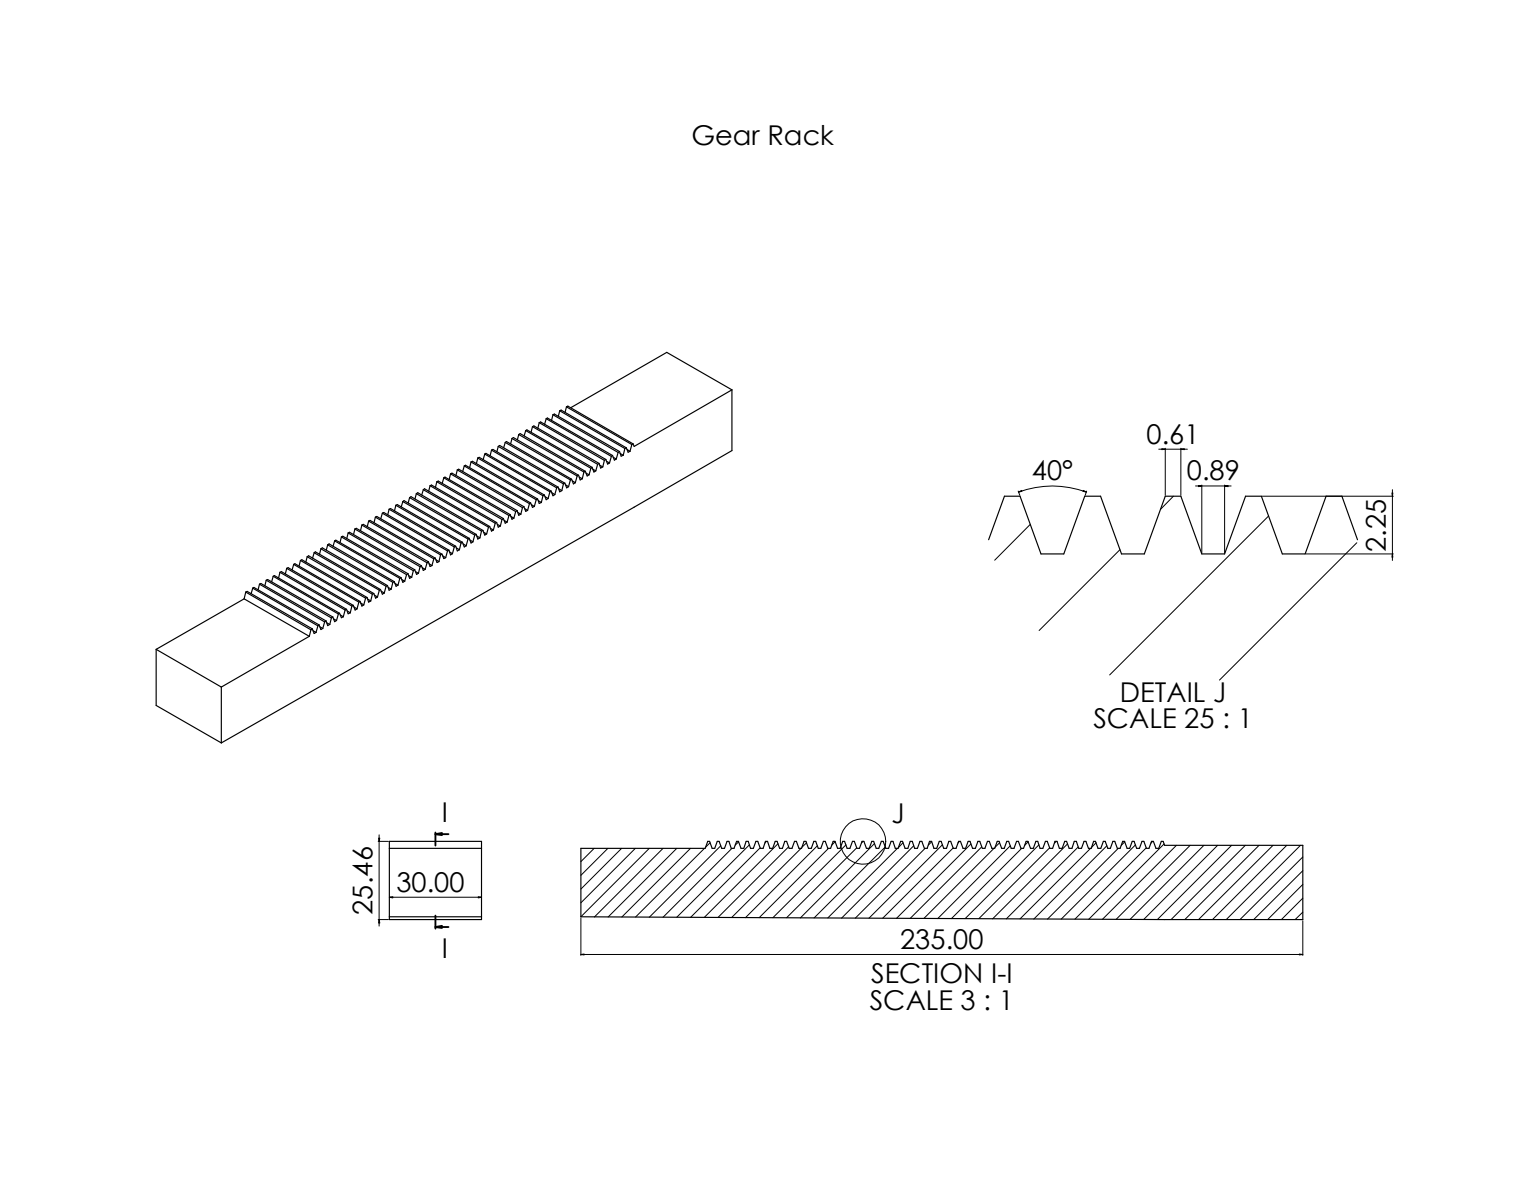
ISO-10303-21;
HEADER;
FILE_DESCRIPTION (('STEP AP214'),
    '1' );
FILE_NAME ('Gear Rack.step',
    '2026-10-21T18:33:49',
    ( '' ),
    ( '' ),
    'SwSTEP 2.0',
    'SolidWorks 2025',
    '' );
FILE_SCHEMA (( 'AUTOMOTIVE_DESIGN' ));
ENDSEC;

DATA;
#3=EDGE_CURVE ( 'NONE', #15101, #1867, #14100, .T. ) ;
#5=DIRECTION ( 'NONE',  ( 0.000000000000000000, 1.000000000000000000, 0.000000000000000000 ) ) ;
#8=FACE_OUTER_BOUND ( 'NONE', #9764, .T. ) ;
#9=EDGE_CURVE ( 'NONE', #4281, #6184, #12794, .T. ) ;
#10=CARTESIAN_POINT ( 'NONE',  ( -68.99615306438082030, 67.98345733813023628, 15.00000000000006928 ) ) ;
#22=ORIENTED_EDGE ( 'NONE', *, *, #922, .F. ) ;
#25=ORIENTED_EDGE ( 'NONE', *, *, #4430, .T. ) ;
#29=VECTOR ( 'NONE', #2801, 1000.000000000000000 ) ;
#33=CARTESIAN_POINT ( 'NONE',  ( -68.99615306438083451, 95.64293533166268446, -15.00000000000001421 ) ) ;
#34=ORIENTED_EDGE ( 'NONE', *, *, #18366, .F. ) ;
#43=CARTESIAN_POINT ( 'NONE',  ( -71.24615306438076345, 119.9567435045637609, 15.00000000000006928 ) ) ;
#54=ORIENTED_EDGE ( 'NONE', *, *, #5988, .F. ) ;
#57=DIRECTION ( 'NONE',  ( 0.000000000000000000, 0.000000000000000000, 1.000000000000000000 ) ) ;
#59=CARTESIAN_POINT ( 'NONE',  ( -71.24615306438080609, 110.5319655545637403, -15.00000000000001421 ) ) ;
#67=DIRECTION ( 'NONE',  ( 1.000000000000000000, 0.000000000000000000, 0.000000000000000000 ) ) ;
#68=DIRECTION ( 'NONE',  ( 0.000000000000000000, 0.000000000000000000, -1.000000000000000000 ) ) ;
#69=LINE ( 'NONE', #1924, #3643 ) ;
#73=LINE ( 'NONE', #1738, #2546 ) ;
#74=CARTESIAN_POINT ( 'NONE',  ( -71.24615306438114715, 12.25372266522925457, -15.00000000000001421 ) ) ;
#76=CARTESIAN_POINT ( 'NONE',  ( -68.99615306438099083, 39.70912348813027393, -15.00000000000001421 ) ) ;
#77=ORIENTED_EDGE ( 'NONE', *, *, #12373, .F. ) ;
#78=ORIENTED_EDGE ( 'NONE', *, *, #14054, .T. ) ;
#79=VECTOR ( 'NONE', #3026, 1000.000000000000000 ) ;
#80=FACE_OUTER_BOUND ( 'NONE', #8908, .T. ) ;
#82=VECTOR ( 'NONE', #10770, 1000.000000000000000 ) ;
#87=CARTESIAN_POINT ( 'NONE',  ( -71.24615306438086293, 87.65194626522927024, 15.00000000000006928 ) ) ;
#88=CARTESIAN_POINT ( 'NONE',  ( -71.24615306438103346, 41.41692725456378099, 15.00000000000006928 ) ) ;
#93=ORIENTED_EDGE ( 'NONE', *, *, #600, .F. ) ;
#95=AXIS2_PLACEMENT_3D ( 'NONE', #13870, #16563, #957 ) ;
#100=VECTOR ( 'NONE', #7999, 1000.000000000000000 ) ;
#101=CARTESIAN_POINT ( 'NONE',  ( -71.24615306438103346, 46.81124181522922356, -167.1454815528550739 ) ) ;
#102=ORIENTED_EDGE ( 'NONE', *, *, #5033, .T. ) ;
#103=VERTEX_POINT ( 'NONE', #8932 ) ;
#105=EDGE_CURVE ( 'NONE', #6184, #7713, #7257, .T. ) ;
#106=DIRECTION ( 'NONE',  ( 0.000000000000000000, 0.000000000000000000, 1.000000000000000000 ) ) ;
#107=CARTESIAN_POINT ( 'NONE',  ( -68.99615306438077766, 111.3508985816626335, 15.00000000000006928 ) ) ;
#108=DIRECTION ( 'NONE',  ( 0.9396926207859110924, 0.3420201433256612189, 4.890320548438462711E-16 ) ) ;
#109=CARTESIAN_POINT ( 'NONE',  ( -68.99615306438083451, 96.25779118813026969, 15.00000000000006928 ) ) ;
#112=CARTESIAN_POINT ( 'NONE',  ( -68.99615306438094819, 64.84186468813030046, -167.1454815528550739 ) ) ;
#115=VERTEX_POINT ( 'NONE', #11567 ) ;
#120=ADVANCED_FACE ( 'NONE', ( #317 ), #17523, .T. ) ;
#123=EDGE_CURVE ( 'NONE', #14184, #1161, #17431, .T. ) ;
#127=ORIENTED_EDGE ( 'NONE', *, *, #11107, .F. ) ;
#131=DIRECTION ( 'NONE',  ( 0.000000000000000000, 1.000000000000000000, 0.000000000000000000 ) ) ;
#132=CLOSED_SHELL ( 'NONE', ( #16819, #11674, #2033, #11644, #4371, #4122, #1296, #5932, #17847, #120, #2885, #7783, #14078, #8551, #16458, #7777, #18333, #11455, #10717, #14761, #5893, #8655, #18440, #16557, #12743, #9060, #2113, #2878, #10557, #2402, #8018, #1483, #10883, #4144, #6355, #12130, #16320, #4815, #13864, #11004, #16568, #13389, #1952, #7426, #15874, #4708, #2702, #9166, #6647, #9938, #17322, #16215, #6855, #13752, #18352, #9497, #4258, #1742, #6653, #8457, #4789, #9269, #18511, #11812, #1620, #13520, #17365, #6946, #1859, #1613, #14320, #1393, #8249, #8120, #5145, #15892, #8683, #10886, #4488, #15641, #15634, #1683, #17355, #13695, #2863, #11359, #9380, #16584, #2602, #1587, #18091, #10091, #697, #5265, #11665, #1664, #1494, #15112, #7329, #13942, #12957, #5269, #13366, #4588, #17837, #11471, #8147, #8734, #4244, #11669, #7993, #15996, #11378, #16587, #15586, #9173, #1719, #9985, #9137, #3228, #3620, #3217, #7092, #3899, #10422, #4564, #11884, #18090, #10942, #9980, #5134, #5026, #2281, #4013, #13406, #12017, #13887, #8689, #14413, #199, #11412, #7110, #12033, #2993, #2286, #360, #17572, #10733, #12952, #12754, #9744, #1961, #13863, #8387, #17357, #7212, #8267, #16341, #10832, #3777, #7577, #14524, #13388, #3293, #4798, #16330, #4522, #14219, #18302, #4015, #3342, #248, #17345, #4135, #15214, #12844, #9850, #14995, #14426, #12814, #8137, #5256, #5374, #4240, #691, #4541, #672, #7328, #12390, #3982, #7563, #1284, #2154, #15527, #5570, #7390, #1348, #13976, #16311 ) ) ;
#133=ORIENTED_EDGE ( 'NONE', *, *, #16066, .F. ) ;
#135=ORIENTED_EDGE ( 'NONE', *, *, #18293, .T. ) ;
#136=VECTOR ( 'NONE', #9589, 1000.000000000000000 ) ;
#137=EDGE_CURVE ( 'NONE', #18033, #6955, #3220, .T. ) ;
#140=EDGE_CURVE ( 'NONE', #5342, #10434, #506, .T. ) ;
#141=AXIS2_PLACEMENT_3D ( 'NONE', #1798, #14535, #303 ) ;
#142=CARTESIAN_POINT ( 'NONE',  ( -71.24615306438106188, 35.13374195456378146, 15.00000000000006928 ) ) ;
#146=VECTOR ( 'NONE', #7240, 1000.000000000000114 ) ;
#158=DIRECTION ( 'NONE',  ( 0.000000000000000000, 0.000000000000000000, -1.000000000000000000 ) ) ;
#160=CARTESIAN_POINT ( 'NONE',  ( -68.99615306438087714, 64.84186468813027204, 15.00000000000006928 ) ) ;
#161=LINE ( 'NONE', #5851, #4306 ) ;
#163=CARTESIAN_POINT ( 'NONE',  ( -71.24615306438072082, 129.3815214545637104, -15.00000000000001421 ) ) ;
#165=DIRECTION ( 'NONE',  ( 0.000000000000000000, 1.000000000000000000, 0.000000000000000000 ) ) ;
#167=ORIENTED_EDGE ( 'NONE', *, *, #3319, .T. ) ;
#168=DIRECTION ( 'NONE',  ( 0.000000000000000000, -1.000000000000000000, 0.000000000000000000 ) ) ;
#172=VECTOR ( 'NONE', #13804, 1000.000000000000000 ) ;
#174=VECTOR ( 'NONE', #6629, 999.9999999999998863 ) ;
#178=EDGE_LOOP ( 'NONE', ( #16402, #10742, #3348, #2661 ) ) ;
#182=VECTOR ( 'NONE', #7830, 1000.000000000000000 ) ;
#185=ORIENTED_EDGE ( 'NONE', *, *, #7525, .T. ) ;
#189=DIRECTION ( 'NONE',  ( -0.9396926207859084279, 0.3420201433256686574, -4.890320548438448905E-16 ) ) ;
#196=CARTESIAN_POINT ( 'NONE',  ( -93.73308511844572877, 147.7866419848965052, 15.00000000000006928 ) ) ;
#198=ORIENTED_EDGE ( 'NONE', *, *, #17480, .F. ) ;
#199=ADVANCED_FACE ( 'NONE', ( #6677 ), #6475, .T. ) ;
#202=LINE ( 'NONE', #14676, #5765 ) ;
#207=CARTESIAN_POINT ( 'NONE',  ( -68.99615306438072082, 139.6252324316626812, -15.00000000000001421 ) ) ;
#211=CARTESIAN_POINT ( 'NONE',  ( -71.24615306438094819, 65.66079771522920794, 15.00000000000006928 ) ) ;
#213=ORIENTED_EDGE ( 'NONE', *, *, #3679, .F. ) ;
#218=DIRECTION ( 'NONE',  ( 0.000000000000000000, 0.000000000000000000, 1.000000000000000000 ) ) ;
#222=FACE_OUTER_BOUND ( 'NONE', #11208, .T. ) ;
#224=CARTESIAN_POINT ( 'NONE',  ( -68.99615306438066398, 143.3816809381303585, -15.00000000000001421 ) ) ;
#226=EDGE_CURVE ( 'NONE', #10713, #3636, #7893, .T. ) ;
#228=ORIENTED_EDGE ( 'NONE', *, *, #586, .F. ) ;
#230=EDGE_LOOP ( 'NONE', ( #6684, #5867, #2533, #3953 ) ) ;
#232=EDGE_CURVE ( 'NONE', #7225, #15152, #10982, .T. ) ;
#235=CARTESIAN_POINT ( 'NONE',  ( -68.99615306438097662, 57.94382353166266597, 15.00000000000006928 ) ) ;
#238=CARTESIAN_POINT ( 'NONE',  ( -68.99615306438094819, 52.27549408813023746, -15.00000000000001421 ) ) ;
#239=CARTESIAN_POINT ( 'NONE',  ( -68.99615306438091977, 76.79337943166271430, 15.00000000000006928 ) ) ;
#242=EDGE_CURVE ( 'NONE', #13281, #15993, #13414, .T. ) ;
#243=CARTESIAN_POINT ( 'NONE',  ( 0.000000000000000000, -47.21335801510345220, 0.000000000000000000 ) ) ;
#245=DIRECTION ( 'NONE',  ( 0.000000000000000000, 1.000000000000000000, 0.000000000000000000 ) ) ;
#246=CARTESIAN_POINT ( 'NONE',  ( -68.99615306438089135, 67.36860148166267948, -15.00000000000001421 ) ) ;
#248=ADVANCED_FACE ( 'NONE', ( #16665 ), #17710, .T. ) ;
#250=EDGE_CURVE ( 'NONE', #2407, #15787, #4070, .T. ) ;
#252=DIRECTION ( 'NONE',  ( 0.000000000000000000, 0.000000000000000000, 1.000000000000000000 ) ) ;
#254=EDGE_LOOP ( 'NONE', ( #4957, #10703, #17741, #2803 ) ) ;
#260=DIRECTION ( 'NONE',  ( 1.000000000000000000, 0.000000000000000000, 0.000000000000000000 ) ) ;
#261=VECTOR ( 'NONE', #17294, 1000.000000000000000 ) ;
#276=LINE ( 'NONE', #12841, #12086 ) ;
#277=CARTESIAN_POINT ( 'NONE',  ( -71.24615306438070661, 137.9174286652292096, -15.00000000000001421 ) ) ;
#278=CARTESIAN_POINT ( 'NONE',  ( -68.99615306438091977, 76.79337943166271430, 15.00000000000006928 ) ) ;
#279=DIRECTION ( 'NONE',  ( -0.9396926207859097602, 0.3420201433256649937, 1.086737899652991371E-16 ) ) ;
#280=CARTESIAN_POINT ( 'NONE',  ( -93.73308511844572877, 147.7866419848965052, -167.1454815528550739 ) ) ;
#281=CARTESIAN_POINT ( 'NONE',  ( -71.24615306438117557, 2.828944715229236628, -15.00000000000001421 ) ) ;
#282=ORIENTED_EDGE ( 'NONE', *, *, #10987, .T. ) ;
#287=CARTESIAN_POINT ( 'NONE',  ( -71.24615306438091977, 78.22716831522920700, -167.1454815528550739 ) ) ;
#288=VERTEX_POINT ( 'NONE', #1257 ) ;
#289=LINE ( 'NONE', #11809, #4058 ) ;
#291=ORIENTED_EDGE ( 'NONE', *, *, #13628, .T. ) ;
#292=VECTOR ( 'NONE', #17881, 1000.000000000000000 ) ;
#294=AXIS2_PLACEMENT_3D ( 'NONE', #10449, #2985, #15881 ) ;
#296=LINE ( 'NONE', #5733, #146 ) ;
#298=LINE ( 'NONE', #4419, #17998 ) ;
#300=ORIENTED_EDGE ( 'NONE', *, *, #349, .T. ) ;
#303=DIRECTION ( 'NONE',  ( -0.9396926207859083169, 0.3420201433256687129, 0.000000000000000000 ) ) ;
#308=PLANE ( 'NONE',  #11935 ) ;
#312=AXIS2_PLACEMENT_3D ( 'NONE', #18500, #6897, #18319 ) ;
#316=VECTOR ( 'NONE', #2722, 1000.000000000000000 ) ;
#317=FACE_OUTER_BOUND ( 'NONE', #5144, .T. ) ;
#320=LINE ( 'NONE', #12982, #15345 ) ;
#324=FACE_OUTER_BOUND ( 'NONE', #5532, .T. ) ;
#327=CARTESIAN_POINT ( 'NONE',  ( -71.24615306438086293, 101.1071876045637055, 15.00000000000006928 ) ) ;
#333=EDGE_CURVE ( 'NONE', #677, #12056, #6961, .T. ) ;
#338=ORIENTED_EDGE ( 'NONE', *, *, #1743, .T. ) ;
#339=ORIENTED_EDGE ( 'NONE', *, *, #18046, .F. ) ;
#341=EDGE_LOOP ( 'NONE', ( #13382, #1827, #3873, #1999 ) ) ;
#342=EDGE_CURVE ( 'NONE', #6852, #6867, #8831, .T. ) ;
#344=EDGE_CURVE ( 'NONE', #16643, #10257, #17318, .T. ) ;
#346=LINE ( 'NONE', #14229, #2566 ) ;
#349=EDGE_CURVE ( 'NONE', #6911, #16349, #396, .T. ) ;
#354=AXIS2_PLACEMENT_3D ( 'NONE', #17589, #6266, #16189 ) ;
#360=ADVANCED_FACE ( 'NONE', ( #11718 ), #4683, .T. ) ;
#364=EDGE_LOOP ( 'NONE', ( #17923, #6580, #8232, #7279 ) ) ;
#366=EDGE_CURVE ( 'NONE', #16976, #11956, #1702, .T. ) ;
#368=( LENGTH_UNIT ( ) NAMED_UNIT ( * ) SI_UNIT ( .MILLI., .METRE. ) );
#371=AXIS2_PLACEMENT_3D ( 'NONE', #10964, #16647, #17683 ) ;
#372=EDGE_LOOP ( 'NONE', ( #7742, #5661, #16335, #12943 ) ) ;
#376=EDGE_CURVE ( 'NONE', #3236, #18474, #3199, .T. ) ;
#379=AXIS2_PLACEMENT_3D ( 'NONE', #9478, #9862, #8069 ) ;
#381=DIRECTION ( 'NONE',  ( 0.9396926207859097602, 0.3420201433256649937, -1.086737899652991371E-16 ) ) ;
#382=ORIENTED_EDGE ( 'NONE', *, *, #14734, .F. ) ;
#383=DIRECTION ( 'NONE',  ( 0.000000000000000000, 1.000000000000000000, 0.000000000000000000 ) ) ;
#385=VECTOR ( 'NONE', #2920, 999.9999999999998863 ) ;
#387=DIRECTION ( 'NONE',  ( 0.000000000000000000, 1.000000000000000000, 0.000000000000000000 ) ) ;
#393=AXIS2_PLACEMENT_3D ( 'NONE', #6338, #7848, #6238 ) ;
#396=LINE ( 'NONE', #4417, #4324 ) ;
#403=DIRECTION ( 'NONE',  ( -0.9396926207859103153, 0.3420201433256634949, -4.890320548438458766E-16 ) ) ;
#405=DIRECTION ( 'NONE',  ( 1.000000000000000000, 0.000000000000000000, 0.000000000000000000 ) ) ;
#406=DIRECTION ( 'NONE',  ( 0.000000000000000000, 0.000000000000000000, 1.000000000000000000 ) ) ;
#407=ORIENTED_EDGE ( 'NONE', *, *, #6384, .T. ) ;
#409=VERTEX_POINT ( 'NONE', #8909 ) ;
#410=VECTOR ( 'NONE', #11298, 1000.000000000000000 ) ;
#411=FACE_OUTER_BOUND ( 'NONE', #8890, .T. ) ;
#413=ORIENTED_EDGE ( 'NONE', *, *, #7885, .T. ) ;
#418=CARTESIAN_POINT ( 'NONE',  ( -71.24615306438117557, 6.859408104563785358, -15.00000000000001421 ) ) ;
#419=ORIENTED_EDGE ( 'NONE', *, *, #16175, .T. ) ;
#422=VECTOR ( 'NONE', #7146, 1000.000000000000000 ) ;
#423=PLANE ( 'NONE',  #11407 ) ;
#425=VERTEX_POINT ( 'NONE', #6170 ) ;
#427=CARTESIAN_POINT ( 'NONE',  ( -68.99615306438070661, 136.4836397816626743, -167.1454815528550739 ) ) ;
#438=ORIENTED_EDGE ( 'NONE', *, *, #10980, .F. ) ;
#442=LINE ( 'NONE', #4723, #8228 ) ;
#444=PLANE ( 'NONE',  #8468 ) ;
#446=ORIENTED_EDGE ( 'NONE', *, *, #6478, .T. ) ;
#448=CARTESIAN_POINT ( 'NONE',  ( -71.24615306438118978, 0.5762228045637974860, -15.00000000000001421 ) ) ;
#450=FACE_OUTER_BOUND ( 'NONE', #16283, .T. ) ;
#455=VERTEX_POINT ( 'NONE', #1621 ) ;
#459=EDGE_CURVE ( 'NONE', #18478, #6989, #7332, .T. ) ;
#462=ORIENTED_EDGE ( 'NONE', *, *, #9043, .F. ) ;
#463=ORIENTED_EDGE ( 'NONE', *, *, #6166, .F. ) ;
#464=VECTOR ( 'NONE', #12334, 1000.000000000000000 ) ;
#471=CARTESIAN_POINT ( 'NONE',  ( -71.24615306438091977, 72.83285375456371469, 15.00000000000006928 ) ) ;
#473=DIRECTION ( 'NONE',  ( 0.3420201433256686574, -0.9396926207859084279, 0.000000000000000000 ) ) ;
#474=PLANE ( 'NONE',  #12259 ) ;
#478=EDGE_CURVE ( 'NONE', #12432, #2231, #13393, .T. ) ;
#483=DIRECTION ( 'NONE',  ( -1.000000000000000000, 0.000000000000000000, -5.022391976381918634E-16 ) ) ;
#490=CARTESIAN_POINT ( 'NONE',  ( -68.99615306438077766, 111.3508985816626335, -167.1454815528550739 ) ) ;
#494=LINE ( 'NONE', #576, #5416 ) ;
#495=ORIENTED_EDGE ( 'NONE', *, *, #6626, .T. ) ;
#499=CARTESIAN_POINT ( 'NONE',  ( -71.24615306438114715, 10.00100075456375492, -167.1454815528550739 ) ) ;
#500=ORIENTED_EDGE ( 'NONE', *, *, #3536, .F. ) ;
#501=ORIENTED_EDGE ( 'NONE', *, *, #3133, .T. ) ;
#506=LINE ( 'NONE', #10147, #14475 ) ;
#508=ORIENTED_EDGE ( 'NONE', *, *, #8600, .F. ) ;
#509=LINE ( 'NONE', #239, #10786 ) ;
#515=DIRECTION ( 'NONE',  ( -0.9396926207859008784, 0.3420201433256891965, 0.000000000000000000 ) ) ;
#520=ORIENTED_EDGE ( 'NONE', *, *, #4378, .T. ) ;
#521=ORIENTED_EDGE ( 'NONE', *, *, #1743, .F. ) ;
#527=CARTESIAN_POINT ( 'NONE',  ( -68.99615306438094819, 54.80223088166269463, 15.00000000000006928 ) ) ;
#529=CARTESIAN_POINT ( 'NONE',  ( -68.99615306438074924, 121.3905323881302962, -167.1454815528550739 ) ) ;
#531=CARTESIAN_POINT ( 'NONE',  ( -71.24615306438101925, 31.99214930456378880, 15.00000000000006928 ) ) ;
#533=VECTOR ( 'NONE', #2270, 1000.000000000000000 ) ;
#536=LINE ( 'NONE', #14927, #15963 ) ;
#547=CARTESIAN_POINT ( 'NONE',  ( -71.24615306438089135, 81.36876096522922808, 15.00000000000006928 ) ) ;
#555=LINE ( 'NONE', #16078, #14389 ) ;
#557=DIRECTION ( 'NONE',  ( -0.9396926207859093161, 0.3420201433256661594, 0.000000000000000000 ) ) ;
#558=VECTOR ( 'NONE', #1688, 1000.000000000000000 ) ;
#560=EDGE_CURVE ( 'NONE', #11029, #18478, #7961, .T. ) ;
#562=DIRECTION ( 'NONE',  ( 0.000000000000000000, 0.000000000000000000, 1.000000000000000000 ) ) ;
#564=ORIENTED_EDGE ( 'NONE', *, *, #8838, .T. ) ;
#568=DIRECTION ( 'NONE',  ( 0.3420201433256649937, -0.9396926207859097602, 0.000000000000000000 ) ) ;
#574=CARTESIAN_POINT ( 'NONE',  ( -71.24615306438076345, 132.5231141045637457, -15.00000000000001421 ) ) ;
#576=CARTESIAN_POINT ( 'NONE',  ( -71.24615306438084872, 72.83285375456374311, 15.00000000000006928 ) ) ;
#581=DIRECTION ( 'NONE',  ( -0.9396926207859084279, 0.3420201433256686574, 1.086737899652989892E-16 ) ) ;
#584=CARTESIAN_POINT ( 'NONE',  ( -71.24615306438091977, 71.94398301522919326, 15.00000000000006928 ) ) ;
#585=ORIENTED_EDGE ( 'NONE', *, *, #478, .F. ) ;
#586=EDGE_CURVE ( 'NONE', #15423, #5470, #3374, .T. ) ;
#587=EDGE_CURVE ( 'NONE', #1317, #10161, #1984, .T. ) ;
#589=ORIENTED_EDGE ( 'NONE', *, *, #5376, .F. ) ;
#590=VECTOR ( 'NONE', #9664, 1000.000000000000000 ) ;
#593=VERTEX_POINT ( 'NONE', #12274 ) ;
#594=CARTESIAN_POINT ( 'NONE',  ( -68.99615306438083451, 95.64293533166268446, -167.1454815528550739 ) ) ;
#596=DIRECTION ( 'NONE',  ( -0.9396926207859171987, 0.3420201433256445100, -4.890320548438495251E-16 ) ) ;
#599=VECTOR ( 'NONE', #9080, 1000.000000000000000 ) ;
#600=EDGE_CURVE ( 'NONE', #16048, #10561, #5150, .T. ) ;
#603=PLANE ( 'NONE',  #8410 ) ;
#613=DIRECTION ( 'NONE',  ( 0.000000000000000000, 0.000000000000000000, 1.000000000000000000 ) ) ;
#617=VECTOR ( 'NONE', #5671, 1000.000000000000000 ) ;
#618=EDGE_LOOP ( 'NONE', ( #14564, #14000, #6336, #1242 ) ) ;
#619=LINE ( 'NONE', #17908, #9368 ) ;
#625=CARTESIAN_POINT ( 'NONE',  ( -68.99615306438089135, 79.93497208166267853, -167.1454815528550739 ) ) ;
#628=CARTESIAN_POINT ( 'NONE',  ( -71.24615306438089135, 84.51035361522924916, -167.1454815528550739 ) ) ;
#629=DIRECTION ( 'NONE',  ( 0.3420201433256649937, -0.9396926207859097602, 0.000000000000000000 ) ) ;
#631=DIRECTION ( 'NONE',  ( 0.000000000000000000, 0.000000000000000000, 1.000000000000000000 ) ) ;
#633=ORIENTED_EDGE ( 'NONE', *, *, #7187, .F. ) ;
#636=CARTESIAN_POINT ( 'NONE',  ( -71.24615306438086293, 90.79353891522923448, 15.00000000000006928 ) ) ;
#638=ORIENTED_EDGE ( 'NONE', *, *, #9, .F. ) ;
#639=DIRECTION ( 'NONE',  ( 0.000000000000000000, 1.000000000000000000, 0.000000000000000000 ) ) ;
#645=LINE ( 'NONE', #6439, #5474 ) ;
#649=DIRECTION ( 'NONE',  ( 0.000000000000000000, 0.000000000000000000, 1.000000000000000000 ) ) ;
#650=DIRECTION ( 'NONE',  ( 0.000000000000000000, 0.000000000000000000, -1.000000000000000000 ) ) ;
#651=PLANE ( 'NONE',  #16727 ) ;
#652=LINE ( 'NONE', #7583, #6407 ) ;
#653=LINE ( 'NONE', #5038, #16770 ) ;
#657=DIRECTION ( 'NONE',  ( 0.9396926207859097602, 0.3420201433256649937, -1.086737899652991371E-16 ) ) ;
#663=VERTEX_POINT ( 'NONE', #5536 ) ;
#664=ORIENTED_EDGE ( 'NONE', *, *, #16224, .F. ) ;
#668=LINE ( 'NONE', #15256, #2163 ) ;
#671=ORIENTED_EDGE ( 'NONE', *, *, #12194, .T. ) ;
#672=ADVANCED_FACE ( 'NONE', ( #7128 ), #8252, .T. ) ;
#675=VECTOR ( 'NONE', #2082, 1000.000000000000000 ) ;
#677=VERTEX_POINT ( 'NONE', #15453 ) ;
#684=FACE_OUTER_BOUND ( 'NONE', #230, .T. ) ;
#686=VECTOR ( 'NONE', #9007, 1000.000000000000000 ) ;
#688=LINE ( 'NONE', #4887, #17550 ) ;
#689=VERTEX_POINT ( 'NONE', #6938 ) ;
#691=ADVANCED_FACE ( 'NONE', ( #15360 ), #11052, .T. ) ;
#693=AXIS2_PLACEMENT_3D ( 'NONE', #2208, #12136, #2384 ) ;
#694=ORIENTED_EDGE ( 'NONE', *, *, #12829, .T. ) ;
#697=ADVANCED_FACE ( 'NONE', ( #8543 ), #8438, .T. ) ;
#698=ORIENTED_EDGE ( 'NONE', *, *, #15200, .T. ) ;
#699=EDGE_CURVE ( 'NONE', #12065, #18179, #4050, .T. ) ;
#702=DIRECTION ( 'NONE',  ( 0.9396926207859097602, 0.3420201433256649381, 4.890320548438455808E-16 ) ) ;
#704=EDGE_CURVE ( 'NONE', #3211, #1616, #14247, .T. ) ;
#711=ORIENTED_EDGE ( 'NONE', *, *, #17825, .T. ) ;
#714=LINE ( 'NONE', #6406, #14338 ) ;
#716=EDGE_CURVE ( 'NONE', #3636, #2613, #10963, .T. ) ;
#722=DIRECTION ( 'NONE',  ( 0.9396926207859185309, 0.3420201433256406798, -1.086737899653001478E-16 ) ) ;
#723=LINE ( 'NONE', #6211, #4284 ) ;
#724=ORIENTED_EDGE ( 'NONE', *, *, #2535, .T. ) ;
#725=FACE_OUTER_BOUND ( 'NONE', #5235, .T. ) ;
#729=ORIENTED_EDGE ( 'NONE', *, *, #18046, .T. ) ;
#731=CARTESIAN_POINT ( 'NONE',  ( -68.99615306438083451, 101.9261206316626698, -15.00000000000001421 ) ) ;
#732=DIRECTION ( 'NONE',  ( 0.000000000000000000, 0.000000000000000000, -1.000000000000000000 ) ) ;
#733=FACE_OUTER_BOUND ( 'NONE', #14539, .T. ) ;
#736=VECTOR ( 'NONE', #16621, 1000.000000000000000 ) ;
#737=VECTOR ( 'NONE', #7847, 1000.000000000000000 ) ;
#738=LINE ( 'NONE', #6614, #17449 ) ;
#740=ORIENTED_EDGE ( 'NONE', *, *, #13031, .T. ) ;
#743=ORIENTED_EDGE ( 'NONE', *, *, #17825, .F. ) ;
#744=EDGE_LOOP ( 'NONE', ( #10644, #10859, #13993, #8792 ) ) ;
#750=CARTESIAN_POINT ( 'NONE',  ( -71.24615306438106188, 34.24487121522926003, -167.1454815528550739 ) ) ;
#751=DIRECTION ( 'NONE',  ( -0.9396926207859068736, 0.3420201433256726542, 0.000000000000000000 ) ) ;
#754=DIRECTION ( 'NONE',  ( 0.000000000000000000, 0.000000000000000000, 1.000000000000000000 ) ) ;
#760=ORIENTED_EDGE ( 'NONE', *, *, #9977, .T. ) ;
#761=AXIS2_PLACEMENT_3D ( 'NONE', #9787, #18401, #5568 ) ;
#762=EDGE_CURVE ( 'NONE', #13170, #4868, #14675, .T. ) ;
#765=CARTESIAN_POINT ( 'NONE',  ( -68.99615306438089135, 79.93497208166267853, -15.00000000000001421 ) ) ;
#770=CARTESIAN_POINT ( 'NONE',  ( -68.99615306438093398, 55.41708673813027985, -15.00000000000001421 ) ) ;
#771=DIRECTION ( 'NONE',  ( 0.000000000000000000, 0.000000000000000000, 1.000000000000000000 ) ) ;
#772=DIRECTION ( 'NONE',  ( 0.000000000000000000, 1.000000000000000000, 0.000000000000000000 ) ) ;
#773=VERTEX_POINT ( 'NONE', #14509 ) ;
#775=CARTESIAN_POINT ( 'NONE',  ( -71.24615306438109030, 31.99214930456376038, -167.1454815528550739 ) ) ;
#776=ORIENTED_EDGE ( 'NONE', *, *, #15222, .T. ) ;
#783=ORIENTED_EDGE ( 'NONE', *, *, #8501, .F. ) ;
#786=EDGE_CURVE ( 'NONE', #3445, #7663, #276, .T. ) ;
#789=DIRECTION ( 'NONE',  ( 0.000000000000000000, 0.000000000000000000, 1.000000000000000000 ) ) ;
#790=ORIENTED_EDGE ( 'NONE', *, *, #9217, .T. ) ;
#792=EDGE_CURVE ( 'NONE', #14885, #13327, #7392, .T. ) ;
#793=DIRECTION ( 'NONE',  ( 0.3420201433256686574, 0.9396926207859084279, -0.000000000000000000 ) ) ;
#794=VERTEX_POINT ( 'NONE', #4665 ) ;
#795=EDGE_CURVE ( 'NONE', #3445, #14282, #1597, .T. ) ;
#797=VERTEX_POINT ( 'NONE', #1868 ) ;
#808=PLANE ( 'NONE',  #6070 ) ;
#810=ORIENTED_EDGE ( 'NONE', *, *, #7346, .F. ) ;
#811=PLANE ( 'NONE',  #4935 ) ;
#814=DIRECTION ( 'NONE',  ( -0.9396926207859084279, 0.3420201433256686574, 1.086737899652989892E-16 ) ) ;
#816=PLANE ( 'NONE',  #16541 ) ;
#817=ORIENTED_EDGE ( 'NONE', *, *, #18293, .F. ) ;
#823=CARTESIAN_POINT ( 'NONE',  ( -68.99615306438094819, 64.84186468813030046, -15.00000000000001421 ) ) ;
#824=ORIENTED_EDGE ( 'NONE', *, *, #14638, .T. ) ;
#825=DIRECTION ( 'NONE',  ( 0.000000000000000000, 1.000000000000000000, 0.000000000000000000 ) ) ;
#826=CARTESIAN_POINT ( 'NONE',  ( -68.99615306438080609, 105.6825691381303045, -15.00000000000001421 ) ) ;
#831=ORIENTED_EDGE ( 'NONE', *, *, #18311, .F. ) ;
#839=DIRECTION ( 'NONE',  ( 0.3420201433256481738, -0.9396926207859158664, 0.000000000000000000 ) ) ;
#842=EDGE_LOOP ( 'NONE', ( #4394, #7797, #7453, #15371 ) ) ;
#844=DIRECTION ( 'NONE',  ( 0.000000000000000000, 0.000000000000000000, -1.000000000000000000 ) ) ;
#846=DIRECTION ( 'NONE',  ( -0.9396926207859069846, 0.3420201433256723766, 1.086737899652988166E-16 ) ) ;
#852=DIRECTION ( 'NONE',  ( 0.000000000000000000, 0.000000000000000000, 1.000000000000000000 ) ) ;
#854=LINE ( 'NONE', #17968, #13566 ) ;
#858=VECTOR ( 'NONE', #7679, 999.9999999999998863 ) ;
#863=CARTESIAN_POINT ( 'NONE',  ( -68.99615306438110451, 5.151604338130280070, 15.00000000000006928 ) ) ;
#865=CARTESIAN_POINT ( 'NONE',  ( -71.24615306438070661, 141.0590213152292449, -167.1454815528550739 ) ) ;
#866=ORIENTED_EDGE ( 'NONE', *, *, #15274, .T. ) ;
#869=ORIENTED_EDGE ( 'NONE', *, *, #6051, .T. ) ;
#876=ORIENTED_EDGE ( 'NONE', *, *, #587, .F. ) ;
#881=VERTEX_POINT ( 'NONE', #4402 ) ;
#886=VECTOR ( 'NONE', #5156, 999.9999999999998863 ) ;
#887=DIRECTION ( 'NONE',  ( 0.000000000000000000, 0.000000000000000000, -1.000000000000000000 ) ) ;
#894=LINE ( 'NONE', #16235, #100 ) ;
#895=ORIENTED_EDGE ( 'NONE', *, *, #333, .F. ) ;
#900=DIRECTION ( 'NONE',  ( 1.000000000000000000, 0.000000000000000000, 0.000000000000000000 ) ) ;
#901=ORIENTED_EDGE ( 'NONE', *, *, #13495, .T. ) ;
#903=EDGE_CURVE ( 'NONE', #18067, #18272, #17218, .T. ) ;
#907=EDGE_CURVE ( 'NONE', #9806, #11339, #8716, .T. ) ;
#910=ORIENTED_EDGE ( 'NONE', *, *, #13180, .T. ) ;
#912=DIRECTION ( 'NONE',  ( 1.000000000000000000, 0.000000000000000000, -1.434969136109119680E-16 ) ) ;
#913=FACE_OUTER_BOUND ( 'NONE', #3223, .T. ) ;
#915=ORIENTED_EDGE ( 'NONE', *, *, #2895, .F. ) ;
#917=VECTOR ( 'NONE', #6803, 1000.000000000000000 ) ;
#921=VECTOR ( 'NONE', #6892, 1000.000000000000000 ) ;
#922=EDGE_CURVE ( 'NONE', #10354, #6955, #14771, .T. ) ;
#923=ORIENTED_EDGE ( 'NONE', *, *, #11202, .T. ) ;
#926=ORIENTED_EDGE ( 'NONE', *, *, #14093, .F. ) ;
#930=EDGE_CURVE ( 'NONE', #5159, #18464, #2044, .T. ) ;
#933=VECTOR ( 'NONE', #4425, 1000.000000000000000 ) ;
#935=VECTOR ( 'NONE', #17439, 1000.000000000000114 ) ;
#936=CARTESIAN_POINT ( 'NONE',  ( -68.99615306438094819, 64.22700883166265839, -167.1454815528550739 ) ) ;
#940=DIRECTION ( 'NONE',  ( 1.000000000000000000, 0.000000000000000000, 0.000000000000000000 ) ) ;
#943=ORIENTED_EDGE ( 'NONE', *, *, #13071, .T. ) ;
#945=DIRECTION ( 'NONE',  ( 0.3420201433256407353, -0.9396926207859186420, 0.000000000000000000 ) ) ;
#950=VECTOR ( 'NONE', #1065, 1000.000000000000000 ) ;
#953=ORIENTED_EDGE ( 'NONE', *, *, #16934, .T. ) ;
#956=CARTESIAN_POINT ( 'NONE',  ( -71.24615306438097662, 57.12489050456376560, -15.00000000000001421 ) ) ;
#957=DIRECTION ( 'NONE',  ( -0.9396926207859084279, 0.3420201433256686574, 0.000000000000000000 ) ) ;
#960=DIRECTION ( 'NONE',  ( 0.000000000000000000, 0.000000000000000000, -1.000000000000000000 ) ) ;
#965=ORIENTED_EDGE ( 'NONE', *, *, #11845, .T. ) ;
#969=LINE ( 'NONE', #17982, #8971 ) ;
#977=FACE_OUTER_BOUND ( 'NONE', #9258, .T. ) ;
#978=ORIENTED_EDGE ( 'NONE', *, *, #7449, .T. ) ;
#983=LINE ( 'NONE', #5281, #7196 ) ;
#984=CARTESIAN_POINT ( 'NONE',  ( -68.99615306438100504, 42.85071613813029501, -15.00000000000001421 ) ) ;
#988=CARTESIAN_POINT ( 'NONE',  ( -71.24615306438091977, 75.97444640456376419, 15.00000000000006928 ) ) ;
#991=VECTOR ( 'NONE', #5970, 1000.000000000000000 ) ;
#995=ORIENTED_EDGE ( 'NONE', *, *, #7003, .T. ) ;
#1003=DIRECTION ( 'NONE',  ( 0.000000000000000000, 0.000000000000000000, 1.000000000000000000 ) ) ;
#1006=FACE_OUTER_BOUND ( 'NONE', #11409, .T. ) ;
#1011=DIRECTION ( 'NONE',  ( 0.000000000000000000, 1.000000000000000000, 0.000000000000000000 ) ) ;
#1013=ORIENTED_EDGE ( 'NONE', *, *, #11348, .F. ) ;
#1017=EDGE_LOOP ( 'NONE', ( #4962, #4427, #3232, #11663 ) ) ;
#1019=LINE ( 'NONE', #2037, #18246 ) ;
#1022=VERTEX_POINT ( 'NONE', #17767 ) ;
#1028=ORIENTED_EDGE ( 'NONE', *, *, #8577, .F. ) ;
#1030=DIRECTION ( 'NONE',  ( -0.9396926207859022107, 0.3420201433256853663, 0.000000000000000000 ) ) ;
#1031=CARTESIAN_POINT ( 'NONE',  ( -68.99615306438069240, 121.3905323881302678, 15.00000000000006928 ) ) ;
#1032=VECTOR ( 'NONE', #279, 1000.000000000000000 ) ;
#1048=CARTESIAN_POINT ( 'NONE',  ( -71.24615306438080609, 104.2487802545637408, -15.00000000000001421 ) ) ;
#1057=ORIENTED_EDGE ( 'NONE', *, *, #13713, .F. ) ;
#1061=PLANE ( 'NONE',  #11505 ) ;
#1064=CARTESIAN_POINT ( 'NONE',  ( -68.99615306438100504, 45.37745293166267402, -15.00000000000001421 ) ) ;
#1065=DIRECTION ( 'NONE',  ( -0.9396926207859167546, 0.3420201433256456203, 1.086737899652999506E-16 ) ) ;
#1068=DIRECTION ( 'NONE',  ( 1.000000000000000000, 0.000000000000000000, 0.000000000000000000 ) ) ;
#1074=EDGE_CURVE ( 'NONE', #7990, #15187, #15432, .T. ) ;
#1076=EDGE_CURVE ( 'NONE', #6989, #4422, #2617, .T. ) ;
#1077=DIRECTION ( 'NONE',  ( 0.9396926207859135349, 0.3420201433256546686, 0.000000000000000000 ) ) ;
#1082=ORIENTED_EDGE ( 'NONE', *, *, #6863, .T. ) ;
#1088=EDGE_LOOP ( 'NONE', ( #7238, #671, #17616, #2992 ) ) ;
#1090=DIRECTION ( 'NONE',  ( 0.000000000000000000, 0.000000000000000000, 1.000000000000000000 ) ) ;
#1093=FACE_OUTER_BOUND ( 'NONE', #6815, .T. ) ;
#1094=LINE ( 'NONE', #12504, #13236 ) ;
#1098=CARTESIAN_POINT ( 'NONE',  ( -71.24615306438103346, 40.52805651522925245, -15.00000000000001421 ) ) ;
#1106=CARTESIAN_POINT ( 'NONE',  ( -71.24615306438109030, 24.82009326522924297, 15.00000000000006928 ) ) ;
#1107=DIRECTION ( 'NONE',  ( 0.3420201433256481738, -0.9396926207859158664, 0.000000000000000000 ) ) ;
#1108=DIRECTION ( 'NONE',  ( 0.000000000000000000, 0.000000000000000000, 1.000000000000000000 ) ) ;
#1110=LINE ( 'NONE', #13923, #617 ) ;
#1112=CARTESIAN_POINT ( 'NONE',  ( -68.99615306438117557, 1.395155831662692192, -15.00000000000001421 ) ) ;
#1121=PLANE ( 'NONE',  #17134 ) ;
#1129=ORIENTED_EDGE ( 'NONE', *, *, #14826, .T. ) ;
#1136=ORIENTED_EDGE ( 'NONE', *, *, #8714, .T. ) ;
#1144=DIRECTION ( 'NONE',  ( 0.9396926207859110924, 0.3420201433256611634, 0.000000000000000000 ) ) ;
#1145=CARTESIAN_POINT ( 'NONE',  ( -71.24615306438079188, 112.7846874652292399, -167.1454815528550739 ) ) ;
#1146=CARTESIAN_POINT ( 'NONE',  ( -71.24615306438077766, 113.6735582045637045, -15.00000000000001421 ) ) ;
#1150=CARTESIAN_POINT ( 'NONE',  ( -94.45685920050698314, -47.21335801510345220, -15.00000000000001421 ) ) ;
#1154=CARTESIAN_POINT ( 'NONE',  ( -71.24615306438070661, 187.7866419848965052, -167.1454815528550739 ) ) ;
#1158=ORIENTED_EDGE ( 'NONE', *, *, #5375, .T. ) ;
#1161=VERTEX_POINT ( 'NONE', #9914 ) ;
#1162=EDGE_CURVE ( 'NONE', #5195, #5717, #8229, .T. ) ;
#1165=LINE ( 'NONE', #7065, #14167 ) ;
#1167=VERTEX_POINT ( 'NONE', #12644 ) ;
#1174=CARTESIAN_POINT ( 'NONE',  ( -71.24615306438079188, 113.6735582045637045, -15.00000000000001421 ) ) ;
#1176=EDGE_CURVE ( 'NONE', #8598, #5018, #18146, .T. ) ;
#1177=CARTESIAN_POINT ( 'NONE',  ( -68.99615306438074924, 121.3905323881302962, -15.00000000000001421 ) ) ;
#1178=VERTEX_POINT ( 'NONE', #13742 ) ;
#1181=ORIENTED_EDGE ( 'NONE', *, *, #10655, .T. ) ;
#1182=DIRECTION ( 'NONE',  ( 0.9396926207859097602, 0.3420201433256649937, -1.086737899652991371E-16 ) ) ;
#1183=VECTOR ( 'NONE', #13108, 1000.000000000000114 ) ;
#1188=EDGE_CURVE ( 'NONE', #18272, #5560, #346, .T. ) ;
#1189=DIRECTION ( 'NONE',  ( 0.000000000000000000, 0.000000000000000000, -1.000000000000000000 ) ) ;
#1191=LINE ( 'NONE', #2388, #921 ) ;
#1193=PLANE ( 'NONE',  #15871 ) ;
#1194=VECTOR ( 'NONE', #8379, 1000.000000000000000 ) ;
#1196=ORIENTED_EDGE ( 'NONE', *, *, #12856, .T. ) ;
#1197=LINE ( 'NONE', #5490, #8699 ) ;
#1201=LINE ( 'NONE', #3900, #6019 ) ;
#1202=LINE ( 'NONE', #15607, #11135 ) ;
#1204=CARTESIAN_POINT ( 'NONE',  ( -71.24615306438117557, 6.859408104563785358, -167.1454815528550739 ) ) ;
#1212=ORIENTED_EDGE ( 'NONE', *, *, #3868, .T. ) ;
#1215=DIRECTION ( 'NONE',  ( 0.000000000000000000, 0.000000000000000000, 1.000000000000000000 ) ) ;
#1219=CARTESIAN_POINT ( 'NONE',  ( -71.24615306438094819, 66.54966845456371516, 15.00000000000006928 ) ) ;
#1221=EDGE_LOOP ( 'NONE', ( #3061, #6392, #5611, #17061 ) ) ;
#1222=VECTOR ( 'NONE', #4657, 1000.000000000000000 ) ;
#1225=DIRECTION ( 'NONE',  ( 0.9396926207859171987, 0.3420201433256444545, -1.086737899652999999E-16 ) ) ;
#1226=ORIENTED_EDGE ( 'NONE', *, *, #7620, .T. ) ;
#1230=VERTEX_POINT ( 'NONE', #14391 ) ;
#1233=VECTOR ( 'NONE', #6721, 1000.000000000000114 ) ;
#1242=ORIENTED_EDGE ( 'NONE', *, *, #7340, .F. ) ;
#1243=DIRECTION ( 'NONE',  ( 0.000000000000000000, 1.000000000000000000, 0.000000000000000000 ) ) ;
#1246=DIRECTION ( 'NONE',  ( -0.9396926207859068736, 0.3420201433256726542, 1.086737899652988043E-16 ) ) ;
#1251=VECTOR ( 'NONE', #17613, 1000.000000000000000 ) ;
#1257=CARTESIAN_POINT ( 'NONE',  ( -71.24615306438089135, 85.39922435456371375, -15.00000000000001421 ) ) ;
#1261=VERTEX_POINT ( 'NONE', #17913 ) ;
#1264=LINE ( 'NONE', #12691, #11810 ) ;
#1268=PLANE ( 'NONE',  #14700 ) ;
#1269=EDGE_CURVE ( 'NONE', #13855, #11938, #442, .T. ) ;
#1271=EDGE_CURVE ( 'NONE', #14048, #12123, #11852, .T. ) ;
#1275=EDGE_CURVE ( 'NONE', #6461, #5649, #7644, .T. ) ;
#1277=CARTESIAN_POINT ( 'NONE',  ( -68.99615306438100504, 39.09426763166271002, -167.1454815528550739 ) ) ;
#1281=ORIENTED_EDGE ( 'NONE', *, *, #1838, .T. ) ;
#1284=ADVANCED_FACE ( 'NONE', ( #10445 ), #17638, .T. ) ;
#1287=PLANE ( 'NONE',  #7582 ) ;
#1292=DIRECTION ( 'NONE',  ( 0.000000000000000000, 0.000000000000000000, 1.000000000000000000 ) ) ;
#1295=EDGE_LOOP ( 'NONE', ( #11443, #1864, #4182, #1863 ) ) ;
#1296=ADVANCED_FACE ( 'NONE', ( #725 ), #811, .T. ) ;
#1303=ORIENTED_EDGE ( 'NONE', *, *, #9270, .T. ) ;
#1306=CARTESIAN_POINT ( 'NONE',  ( -68.99615306438094819, 70.51019413166270056, -167.1454815528550739 ) ) ;
#1309=CARTESIAN_POINT ( 'NONE',  ( -68.99615306438077766, 123.9172691816626610, -167.1454815528550739 ) ) ;
#1310=CARTESIAN_POINT ( 'NONE',  ( -71.24615306438086293, 87.65194626522927024, -15.00000000000001421 ) ) ;
#1312=ORIENTED_EDGE ( 'NONE', *, *, #15097, .T. ) ;
#1315=AXIS2_PLACEMENT_3D ( 'NONE', #12349, #13837, #16264 ) ;
#1317=VERTEX_POINT ( 'NONE', #16413 ) ;
#1318=CARTESIAN_POINT ( 'NONE',  ( -68.99615306438070661, 124.5321250381302463, 15.00000000000006928 ) ) ;
#1321=ORIENTED_EDGE ( 'NONE', *, *, #5948, .T. ) ;
#1322=LINE ( 'NONE', #4025, #1514 ) ;
#1326=EDGE_LOOP ( 'NONE', ( #17659, #2695, #11593, #11689 ) ) ;
#1328=VECTOR ( 'NONE', #6888, 1000.000000000000000 ) ;
#1329=AXIS2_PLACEMENT_3D ( 'NONE', #12687, #9772, #2750 ) ;
#1330=CARTESIAN_POINT ( 'NONE',  ( -68.99615306438077766, 123.9172691816626610, 15.00000000000006928 ) ) ;
#1333=CARTESIAN_POINT ( 'NONE',  ( -71.24615306438076345, 119.0678727652292253, -15.00000000000001421 ) ) ;
#1335=ORIENTED_EDGE ( 'NONE', *, *, #1955, .T. ) ;
#1337=AXIS2_PLACEMENT_3D ( 'NONE', #5488, #5388, #2600 ) ;
#1339=DIRECTION ( 'NONE',  ( 0.000000000000000000, 1.000000000000000000, 0.000000000000000000 ) ) ;
#1345=VERTEX_POINT ( 'NONE', #6127 ) ;
#1346=CARTESIAN_POINT ( 'NONE',  ( -68.99615306438086293, 93.11619853813030545, -167.1454815528550739 ) ) ;
#1348=ADVANCED_FACE ( 'NONE', ( #3426 ), #11941, .F. ) ;
#1350=DIRECTION ( 'NONE',  ( 0.9396926207859145341, 0.3420201433256520596, -1.086737899652996918E-16 ) ) ;
#1359=CARTESIAN_POINT ( 'NONE',  ( -71.24615306438113294, 16.28418605456381130, -15.00000000000001421 ) ) ;
#1361=VECTOR ( 'NONE', #3702, 1000.000000000000000 ) ;
#1362=ORIENTED_EDGE ( 'NONE', *, *, #12939, .F. ) ;
#1364=VECTOR ( 'NONE', #13661, 1000.000000000000000 ) ;
#1366=LINE ( 'NONE', #15572, #10483 ) ;
#1371=LINE ( 'NONE', #4348, #2465 ) ;
#1373=DIRECTION ( 'NONE',  ( 1.000000000000000000, 0.000000000000000000, 0.000000000000000000 ) ) ;
#1376=EDGE_LOOP ( 'NONE', ( #11061, #102, #5489, #7491 ) ) ;
#1378=VECTOR ( 'NONE', #1756, 1000.000000000000114 ) ;
#1384=ORIENTED_EDGE ( 'NONE', *, *, #15430, .T. ) ;
#1388=ORIENTED_EDGE ( 'NONE', *, *, #3398, .T. ) ;
#1389=DIRECTION ( 'NONE',  ( 0.000000000000000000, 1.000000000000000000, 0.000000000000000000 ) ) ;
#1393=ADVANCED_FACE ( 'NONE', ( #18167 ), #2448, .T. ) ;
#1396=LINE ( 'NONE', #14119, #8408 ) ;
#1397=LINE ( 'NONE', #14298, #14637 ) ;
#1406=CARTESIAN_POINT ( 'NONE',  ( -68.99615306438109030, 17.10311908166270456, 15.00000000000006928 ) ) ;
#1409=ORIENTED_EDGE ( 'NONE', *, *, #12225, .F. ) ;
#1411=FACE_OUTER_BOUND ( 'NONE', #8639, .T. ) ;
#1418=LINE ( 'NONE', #7121, #16123 ) ;
#1422=ORIENTED_EDGE ( 'NONE', *, *, #17047, .T. ) ;
#1425=EDGE_CURVE ( 'NONE', #15985, #9812, #6533, .T. ) ;
#1427=DIRECTION ( 'NONE',  ( 0.000000000000000000, 0.000000000000000000, 1.000000000000000000 ) ) ;
#1428=CARTESIAN_POINT ( 'NONE',  ( -68.99615306438106188, 23.38630438166269698, 15.00000000000006928 ) ) ;
#1432=LINE ( 'NONE', #1154, #8770 ) ;
#1434=EDGE_LOOP ( 'NONE', ( #6050, #2066, #16636, #4642 ) ) ;
#1435=CARTESIAN_POINT ( 'NONE',  ( -68.99615306438084872, 77.40823528813027110, 15.00000000000006928 ) ) ;
#1449=LINE ( 'NONE', #15934, #17350 ) ;
#1452=ORIENTED_EDGE ( 'NONE', *, *, #344, .T. ) ;
#1454=VERTEX_POINT ( 'NONE', #11037 ) ;
#1455=ORIENTED_EDGE ( 'NONE', *, *, #11815, .T. ) ;
#1460=VERTEX_POINT ( 'NONE', #10275 ) ;
#1463=DIRECTION ( 'NONE',  ( 0.9396926207859084279, 0.3420201433256686574, -1.086737899652989892E-16 ) ) ;
#1464=DIRECTION ( 'NONE',  ( 0.000000000000000000, 0.000000000000000000, 1.000000000000000000 ) ) ;
#1465=DIRECTION ( 'NONE',  ( 0.000000000000000000, 0.000000000000000000, -1.000000000000000000 ) ) ;
#1467=ORIENTED_EDGE ( 'NONE', *, *, #13031, .F. ) ;
#1468=PLANE ( 'NONE',  #7795 ) ;
#1469=AXIS2_PLACEMENT_3D ( 'NONE', #9795, #9990, #12519 ) ;
#1470=LINE ( 'NONE', #7366, #10220 ) ;
#1475=EDGE_CURVE ( 'NONE', #11152, #12417, #4207, .T. ) ;
#1477=CARTESIAN_POINT ( 'NONE',  ( -68.99615306438120399, -1.746436818337276931, -15.00000000000001421 ) ) ;
#1478=ORIENTED_EDGE ( 'NONE', *, *, #12242, .F. ) ;
#1480=VECTOR ( 'NONE', #6149, 1000.000000000000000 ) ;
#1482=ORIENTED_EDGE ( 'NONE', *, *, #9753, .F. ) ;
#1483=ADVANCED_FACE ( 'NONE', ( #1411 ), #5955, .T. ) ;
#1484=AXIS2_PLACEMENT_3D ( 'NONE', #18009, #16226, #9221 ) ;
#1486=DIRECTION ( 'NONE',  ( 0.000000000000000000, 0.000000000000000000, 1.000000000000000000 ) ) ;
#1487=CARTESIAN_POINT ( 'NONE',  ( -71.24615306438076345, 119.9567435045637609, -167.1454815528550739 ) ) ;
#1490=CARTESIAN_POINT ( 'NONE',  ( -68.99615306438094819, 54.80223088166269463, -15.00000000000001421 ) ) ;
#1491=CARTESIAN_POINT ( 'NONE',  ( -68.99615306438077766, 115.1073470881302541, -167.1454815528550739 ) ) ;
#1492=EDGE_LOOP ( 'NONE', ( #3530, #10028, #18416, #8612 ) ) ;
#1494=ADVANCED_FACE ( 'NONE', ( #1673 ), #15883, .T. ) ;
#1499=EDGE_CURVE ( 'NONE', #16011, #4288, #11679, .T. ) ;
#1500=CARTESIAN_POINT ( 'NONE',  ( -68.99615306438083451, 96.25779118813026969, -15.00000000000001421 ) ) ;
#1501=VECTOR ( 'NONE', #11263, 999.9999999999998863 ) ;
#1503=ORIENTED_EDGE ( 'NONE', *, *, #8170, .T. ) ;
#1509=LINE ( 'NONE', #8625, #8478 ) ;
#1510=AXIS2_PLACEMENT_3D ( 'NONE', #11710, #6160, #4861 ) ;
#1511=CARTESIAN_POINT ( 'NONE',  ( -68.99615306438080609, 108.8241617881302545, -15.00000000000001421 ) ) ;
#1512=EDGE_CURVE ( 'NONE', #425, #18243, #17284, .T. ) ;
#1514=VECTOR ( 'NONE', #5414, 999.9999999999998863 ) ;
#1516=VECTOR ( 'NONE', #2698, 1000.000000000000000 ) ;
#1519=VERTEX_POINT ( 'NONE', #12751 ) ;
#1522=ORIENTED_EDGE ( 'NONE', *, *, #8000, .F. ) ;
#1527=VECTOR ( 'NONE', #9452, 1000.000000000000000 ) ;
#1533=DIRECTION ( 'NONE',  ( 1.000000000000000000, 0.000000000000000000, 0.000000000000000000 ) ) ;
#1534=DIRECTION ( 'NONE',  ( 0.3420201433256686574, 0.9396926207859084279, -0.000000000000000000 ) ) ;
#1535=VERTEX_POINT ( 'NONE', #4302 ) ;
#1538=DIRECTION ( 'NONE',  ( 0.9396926207859148672, 0.3420201433256507273, 0.000000000000000000 ) ) ;
#1543=LINE ( 'NONE', #2766, #3559 ) ;
#1544=ORIENTED_EDGE ( 'NONE', *, *, #15274, .F. ) ;
#1545=EDGE_LOOP ( 'NONE', ( #2115, #5640, #5377, #8327 ) ) ;
#1547=ORIENTED_EDGE ( 'NONE', *, *, #16169, .F. ) ;
#1550=ORIENTED_EDGE ( 'NONE', *, *, #13051, .T. ) ;
#1552=ORIENTED_EDGE ( 'NONE', *, *, #7421, .T. ) ;
#1553=CARTESIAN_POINT ( 'NONE',  ( -68.99615306438070661, 140.2400882881302948, -15.00000000000001421 ) ) ;
#1555=DIRECTION ( 'NONE',  ( 0.000000000000000000, 0.000000000000000000, 1.000000000000000000 ) ) ;
#1558=AXIS2_PLACEMENT_3D ( 'NONE', #9037, #14726, #7811 ) ;
#1559=CARTESIAN_POINT ( 'NONE',  ( -68.99615306438072082, 127.0588618316627105, -167.1454815528550739 ) ) ;
#1565=VECTOR ( 'NONE', #8531, 1000.000000000000000 ) ;
#1566=CARTESIAN_POINT ( 'NONE',  ( -68.99615306438094819, 70.51019413166270056, -15.00000000000001421 ) ) ;
#1569=ORIENTED_EDGE ( 'NONE', *, *, #3664, .F. ) ;
#1572=VECTOR ( 'NONE', #9277, 1000.000000000000000 ) ;
#1576=CARTESIAN_POINT ( 'NONE',  ( -71.24615306438106188, 37.38646386522923137, -15.00000000000001421 ) ) ;
#1581=PLANE ( 'NONE',  #6951 ) ;
#1582=ORIENTED_EDGE ( 'NONE', *, *, #9376, .T. ) ;
#1587=ADVANCED_FACE ( 'NONE', ( #2907 ), #8693, .T. ) ;
#1591=DIRECTION ( 'NONE',  ( 0.000000000000000000, 1.000000000000000000, 0.000000000000000000 ) ) ;
#1594=EDGE_LOOP ( 'NONE', ( #5775, #9382, #2860, #1057 ) ) ;
#1595=VECTOR ( 'NONE', #6503, 1000.000000000000000 ) ;
#1597=LINE ( 'NONE', #17127, #15379 ) ;
#1609=LINE ( 'NONE', #17494, #12670 ) ;
#1613=ADVANCED_FACE ( 'NONE', ( #17468 ), #13270, .T. ) ;
#1616=VERTEX_POINT ( 'NONE', #8880 ) ;
#1617=AXIS2_PLACEMENT_3D ( 'NONE', #17088, #18415, #11303 ) ;
#1619=ORIENTED_EDGE ( 'NONE', *, *, #795, .T. ) ;
#1620=ADVANCED_FACE ( 'NONE', ( #450 ), #11946, .T. ) ;
#1621=CARTESIAN_POINT ( 'NONE',  ( -68.99615306438089135, 86.21815738166266385, -15.00000000000001421 ) ) ;
#1622=EDGE_CURVE ( 'NONE', #288, #455, #4830, .T. ) ;
#1624=LINE ( 'NONE', #7334, #18309 ) ;
#1626=ORIENTED_EDGE ( 'NONE', *, *, #3642, .T. ) ;
#1627=EDGE_CURVE ( 'NONE', #2025, #11979, #10549, .T. ) ;
#1633=FACE_OUTER_BOUND ( 'NONE', #16999, .T. ) ;
#1637=VECTOR ( 'NONE', #1965, 1000.000000000000000 ) ;
#1641=ORIENTED_EDGE ( 'NONE', *, *, #14385, .T. ) ;
#1642=VECTOR ( 'NONE', #3579, 1000.000000000000000 ) ;
#1644=VECTOR ( 'NONE', #9718, 1000.000000000000000 ) ;
#1645=AXIS2_PLACEMENT_3D ( 'NONE', #15236, #839, #5130 ) ;
#1648=DIRECTION ( 'NONE',  ( 0.000000000000000000, 1.000000000000000000, 0.000000000000000000 ) ) ;
#1649=LINE ( 'NONE', #13075, #8345 ) ;
#1650=CARTESIAN_POINT ( 'NONE',  ( -68.99615306438094819, 51.66063823166267355, 15.00000000000006928 ) ) ;
#1651=DIRECTION ( 'NONE',  ( 0.000000000000000000, 0.000000000000000000, -1.000000000000000000 ) ) ;
#1652=ORIENTED_EDGE ( 'NONE', *, *, #11348, .T. ) ;
#1653=DIRECTION ( 'NONE',  ( 1.000000000000000000, 0.000000000000000000, 0.000000000000000000 ) ) ;
#1654=CARTESIAN_POINT ( 'NONE',  ( -71.24615306438109030, 31.10327856522923540, -167.1454815528550739 ) ) ;
#1658=AXIS2_PLACEMENT_3D ( 'NONE', #8609, #14313, #12919 ) ;
#1662=VERTEX_POINT ( 'NONE', #4932 ) ;
#1664=ADVANCED_FACE ( 'NONE', ( #3518 ), #9151, .T. ) ;
#1670=PLANE ( 'NONE',  #4317 ) ;
#1671=ORIENTED_EDGE ( 'NONE', *, *, #12257, .F. ) ;
#1673=FACE_OUTER_BOUND ( 'NONE', #10403, .T. ) ;
#1674=CARTESIAN_POINT ( 'NONE',  ( -71.24615306438080609, 103.3599095152292193, -167.1454815528550739 ) ) ;
#1678=LINE ( 'NONE', #15889, #13452 ) ;
#1680=DIRECTION ( 'NONE',  ( -0.9396926207859008784, 0.3420201433256891965, -4.890320548438409462E-16 ) ) ;
#1681=CARTESIAN_POINT ( 'NONE',  ( -68.99615306438077766, 114.4924912316626688, 15.00000000000006928 ) ) ;
#1683=ADVANCED_FACE ( 'NONE', ( #16145 ), #6424, .T. ) ;
#1684=ORIENTED_EDGE ( 'NONE', *, *, #18102, .F. ) ;
#1685=ORIENTED_EDGE ( 'NONE', *, *, #6372, .F. ) ;
#1686=DIRECTION ( 'NONE',  ( 0.000000000000000000, 0.000000000000000000, 1.000000000000000000 ) ) ;
#1687=CARTESIAN_POINT ( 'NONE',  ( -68.99615306438083451, 102.5409764881302692, -167.1454815528550739 ) ) ;
#1688=DIRECTION ( 'NONE',  ( 0.000000000000000000, 1.000000000000000000, 0.000000000000000000 ) ) ;
#1692=ORIENTED_EDGE ( 'NONE', *, *, #9138, .F. ) ;
#1696=EDGE_LOOP ( 'NONE', ( #13023, #4065, #7411, #10027 ) ) ;
#1697=CARTESIAN_POINT ( 'NONE',  ( -68.99615306438106188, 23.38630438166269698, -167.1454815528550739 ) ) ;
#1702=LINE ( 'NONE', #16087, #17458 ) ;
#1704=CARTESIAN_POINT ( 'NONE',  ( -68.99615306438117557, 2.010011688130281193, 15.00000000000006928 ) ) ;
#1706=ORIENTED_EDGE ( 'NONE', *, *, #8132, .F. ) ;
#1707=EDGE_CURVE ( 'NONE', #14706, #2059, #13179, .T. ) ;
#1709=CARTESIAN_POINT ( 'NONE',  ( -68.99615306438073503, 105.6825691381302761, 15.00000000000006928 ) ) ;
#1716=VERTEX_POINT ( 'NONE', #1851 ) ;
#1718=ORIENTED_EDGE ( 'NONE', *, *, #903, .F. ) ;
#1719=ADVANCED_FACE ( 'NONE', ( #9711 ), #5392, .T. ) ;
#1721=EDGE_CURVE ( 'NONE', #7210, #14794, #5491, .T. ) ;
#1722=ORIENTED_EDGE ( 'NONE', *, *, #15781, .F. ) ;
#1730=DIRECTION ( 'NONE',  ( -0.9396926207859069846, 0.3420201433256723766, 1.086737899652988166E-16 ) ) ;
#1731=CARTESIAN_POINT ( 'NONE',  ( -71.24615306438076345, 132.5231141045637457, 15.00000000000006928 ) ) ;
#1733=ORIENTED_EDGE ( 'NONE', *, *, #16224, .T. ) ;
#1734=PLANE ( 'NONE',  #3910 ) ;
#1737=ORIENTED_EDGE ( 'NONE', *, *, #5821, .T. ) ;
#1738=CARTESIAN_POINT ( 'NONE',  ( -68.99615306438109030, 17.71797493813028268, -167.1454815528550739 ) ) ;
#1742=ADVANCED_FACE ( 'NONE', ( #6607 ), #6898, .T. ) ;
#1743=EDGE_CURVE ( 'NONE', #4878, #13376, #18026, .T. ) ;
#1745=VERTEX_POINT ( 'NONE', #18129 ) ;
#1751=VECTOR ( 'NONE', #2825, 1000.000000000000000 ) ;
#1756=DIRECTION ( 'NONE',  ( -0.9396926207859171987, 0.3420201433256444545, 1.086737899652999999E-16 ) ) ;
#1759=CARTESIAN_POINT ( 'NONE',  ( -71.24615306438076345, 125.3510580652292248, 15.00000000000006928 ) ) ;
#1760=ORIENTED_EDGE ( 'NONE', *, *, #18165, .T. ) ;
#1772=LINE ( 'NONE', #1871, #3126 ) ;
#1775=LINE ( 'NONE', #1428, #14980 ) ;
#1776=ORIENTED_EDGE ( 'NONE', *, *, #16329, .F. ) ;
#1777=AXIS2_PLACEMENT_3D ( 'NONE', #6183, #16658, #11066 ) ;
#1782=DIRECTION ( 'NONE',  ( 0.9396926207859157554, 0.3420201433256481738, 4.890320548438487362E-16 ) ) ;
#1783=ORIENTED_EDGE ( 'NONE', *, *, #5382, .T. ) ;
#1790=VECTOR ( 'NONE', #11526, 1000.000000000000114 ) ;
#1791=DIRECTION ( 'NONE',  ( 0.000000000000000000, 0.000000000000000000, 1.000000000000000000 ) ) ;
#1793=CARTESIAN_POINT ( 'NONE',  ( -68.99615306438072082, 133.3420471316626958, 15.00000000000006928 ) ) ;
#1797=DIRECTION ( 'NONE',  ( 0.000000000000000000, 1.000000000000000000, 0.000000000000000000 ) ) ;
#1798=CARTESIAN_POINT ( 'NONE',  ( -68.99615306438106188, 30.28434553813027108, -167.1454815528550739 ) ) ;
#1800=EDGE_CURVE ( 'NONE', #17240, #9888, #2217, .T. ) ;
#1802=ORIENTED_EDGE ( 'NONE', *, *, #13045, .T. ) ;
#1803=VECTOR ( 'NONE', #8241, 1000.000000000000114 ) ;
#1804=CARTESIAN_POINT ( 'NONE',  ( -93.54007869656271623, 187.7866419848965052, -167.1454815528550739 ) ) ;
#1806=VECTOR ( 'NONE', #12722, 1000.000000000000000 ) ;
#1807=FACE_OUTER_BOUND ( 'NONE', #3297, .T. ) ;
#1812=VECTOR ( 'NONE', #17999, 1000.000000000000000 ) ;
#1815=ORIENTED_EDGE ( 'NONE', *, *, #15689, .T. ) ;
#1818=DIRECTION ( 'NONE',  ( 0.000000000000000000, 0.000000000000000000, 1.000000000000000000 ) ) ;
#1821=DIRECTION ( 'NONE',  ( 0.000000000000000000, 0.000000000000000000, 1.000000000000000000 ) ) ;
#1827=ORIENTED_EDGE ( 'NONE', *, *, #10358, .T. ) ;
#1828=VECTOR ( 'NONE', #11972, 1000.000000000000000 ) ;
#1829=LINE ( 'NONE', #3233, #12097 ) ;
#1835=VECTOR ( 'NONE', #10206, 1000.000000000000000 ) ;
#1836=ORIENTED_EDGE ( 'NONE', *, *, #15430, .F. ) ;
#1837=ORIENTED_EDGE ( 'NONE', *, *, #14416, .T. ) ;
#1838=EDGE_CURVE ( 'NONE', #14417, #5330, #4515, .T. ) ;
#1839=VERTEX_POINT ( 'NONE', #1899 ) ;
#1846=DIRECTION ( 'NONE',  ( 0.000000000000000000, 1.000000000000000000, 0.000000000000000000 ) ) ;
#1848=LINE ( 'NONE', #448, #5404 ) ;
#1851=CARTESIAN_POINT ( 'NONE',  ( -71.24615306438094819, 66.54966845456371516, -15.00000000000001421 ) ) ;
#1854=CARTESIAN_POINT ( 'NONE',  ( -71.24615306438070661, 135.6647067545637242, -167.1454815528550739 ) ) ;
#1859=ADVANCED_FACE ( 'NONE', ( #1633 ), #13321, .T. ) ;
#1863=ORIENTED_EDGE ( 'NONE', *, *, #4574, .F. ) ;
#1864=ORIENTED_EDGE ( 'NONE', *, *, #15087, .T. ) ;
#1867=VERTEX_POINT ( 'NONE', #15936 ) ;
#1868=CARTESIAN_POINT ( 'NONE',  ( -68.99615306438072082, 127.6737176881302958, -15.00000000000001421 ) ) ;
#1869=CARTESIAN_POINT ( 'NONE',  ( -68.99615306438111872, 11.43478963813029914, -15.00000000000001421 ) ) ;
#1871=CARTESIAN_POINT ( 'NONE',  ( -68.99615306438117557, 4.536748481662661092, 15.00000000000006928 ) ) ;
#1873=DIRECTION ( 'NONE',  ( 0.000000000000000000, 0.000000000000000000, 1.000000000000000000 ) ) ;
#1875=DIRECTION ( 'NONE',  ( 0.000000000000000000, 0.000000000000000000, -1.000000000000000000 ) ) ;
#1878=CARTESIAN_POINT ( 'NONE',  ( -68.99615306438086293, 89.35975003166268493, -167.1454815528550739 ) ) ;
#1881=PLANE ( 'NONE',  #7756 ) ;
#1883=DIRECTION ( 'NONE',  ( 0.000000000000000000, 0.000000000000000000, 1.000000000000000000 ) ) ;
#1886=AXIS2_PLACEMENT_3D ( 'NONE', #16649, #8687, #3844 ) ;
#1887=EDGE_LOOP ( 'NONE', ( #13670, #1802, #10861, #14344 ) ) ;
#1890=VECTOR ( 'NONE', #14889, 1000.000000000000000 ) ;
#1892=LINE ( 'NONE', #16184, #10888 ) ;
#1899=CARTESIAN_POINT ( 'NONE',  ( -71.24615306438120399, 0.5762228045637918239, -15.00000000000001421 ) ) ;
#1901=ORIENTED_EDGE ( 'NONE', *, *, #10256, .T. ) ;
#1902=LINE ( 'NONE', #1804, #13137 ) ;
#1909=EDGE_LOOP ( 'NONE', ( #2214, #7127, #13459, #10693 ) ) ;
#1915=DIRECTION ( 'NONE',  ( 0.9396926207859084279, 0.3420201433256686574, -1.086737899652989892E-16 ) ) ;
#1917=LINE ( 'NONE', #2959, #18274 ) ;
#1918=PLANE ( 'NONE',  #3131 ) ;
#1919=ORIENTED_EDGE ( 'NONE', *, *, #8256, .T. ) ;
#1924=CARTESIAN_POINT ( 'NONE',  ( -68.99615306438080609, 108.2093059316626693, -15.00000000000001421 ) ) ;
#1929=CARTESIAN_POINT ( 'NONE',  ( -71.24615306438111872, 22.56737135456379661, -167.1454815528550739 ) ) ;
#1930=VECTOR ( 'NONE', #702, 1000.000000000000114 ) ;
#1941=VECTOR ( 'NONE', #8824, 1000.000000000000114 ) ;
#1943=EDGE_CURVE ( 'NONE', #15911, #13807, #6093, .T. ) ;
#1948=VECTOR ( 'NONE', #14398, 1000.000000000000000 ) ;
#1949=LINE ( 'NONE', #13357, #7829 ) ;
#1950=LINE ( 'NONE', #5879, #11998 ) ;
#1952=ADVANCED_FACE ( 'NONE', ( #8401 ), #14112, .T. ) ;
#1954=EDGE_LOOP ( 'NONE', ( #8661, #729, #3298, #2153 ) ) ;
#1955=EDGE_CURVE ( 'NONE', #13329, #18188, #11727, .T. ) ;
#1958=EDGE_CURVE ( 'NONE', #6487, #4021, #4185, .T. ) ;
#1961=ADVANCED_FACE ( 'NONE', ( #13227 ), #11306, .T. ) ;
#1964=ORIENTED_EDGE ( 'NONE', *, *, #5009, .T. ) ;
#1965=DIRECTION ( 'NONE',  ( 0.000000000000000000, 0.000000000000000000, 1.000000000000000000 ) ) ;
#1967=CARTESIAN_POINT ( 'NONE',  ( -68.99615306438100504, 48.51904558166270220, -167.1454815528550739 ) ) ;
#1968=EDGE_CURVE ( 'NONE', #7210, #13855, #12283, .T. ) ;
#1971=LINE ( 'NONE', #7670, #2547 ) ;
#1973=ORIENTED_EDGE ( 'NONE', *, *, #6042, .F. ) ;
#1976=CARTESIAN_POINT ( 'NONE',  ( -71.24615306438100504, 53.09442711522921599, 15.00000000000006928 ) ) ;
#1979=PLANE ( 'NONE',  #5827 ) ;
#1983=ORIENTED_EDGE ( 'NONE', *, *, #18140, .T. ) ;
#1984=LINE ( 'NONE', #9369, #10395 ) ;
#1986=LINE ( 'NONE', #13395, #15924 ) ;
#1989=DIRECTION ( 'NONE',  ( -0.9396926207859171987, 0.3420201433256444545, 0.000000000000000000 ) ) ;
#1999=ORIENTED_EDGE ( 'NONE', *, *, #7664, .F. ) ;
#2001=LINE ( 'NONE', #12297, #12639 ) ;
#2002=ORIENTED_EDGE ( 'NONE', *, *, #3001, .F. ) ;
#2007=ORIENTED_EDGE ( 'NONE', *, *, #8577, .T. ) ;
#2015=ORIENTED_EDGE ( 'NONE', *, *, #7574, .T. ) ;
#2023=LINE ( 'NONE', #14834, #4275 ) ;
#2025=VERTEX_POINT ( 'NONE', #17694 ) ;
#2027=CARTESIAN_POINT ( 'NONE',  ( -68.99615306438094819, 51.66063823166267355, -167.1454815528550739 ) ) ;
#2033=ADVANCED_FACE ( 'NONE', ( #13776 ), #2081, .T. ) ;
#2037=CARTESIAN_POINT ( 'NONE',  ( -68.99615306438067819, 145.9084177316626949, -15.00000000000001421 ) ) ;
#2044=LINE ( 'NONE', #6337, #7611 ) ;
#2051=PRODUCT ( 'Gear Rack', 'Gear Rack', '', ( #9143 ) ) ;
#2054=EDGE_CURVE ( 'NONE', #2374, #15750, #9108, .T. ) ;
#2055=CARTESIAN_POINT ( 'NONE',  ( -71.24615306438076345, 123.0983361545637109, -15.00000000000001421 ) ) ;
#2057=DIRECTION ( 'NONE',  ( 0.3420201433256686574, 0.9396926207859084279, -0.000000000000000000 ) ) ;
#2059=VERTEX_POINT ( 'NONE', #5162 ) ;
#2066=ORIENTED_EDGE ( 'NONE', *, *, #5268, .T. ) ;
#2067=EDGE_CURVE ( 'NONE', #17780, #8569, #9558, .T. ) ;
#2072=FACE_OUTER_BOUND ( 'NONE', #7816, .T. ) ;
#2073=EDGE_CURVE ( 'NONE', #14401, #7613, #15264, .T. ) ;
#2074=ORIENTED_EDGE ( 'NONE', *, *, #12359, .T. ) ;
#2076=VECTOR ( 'NONE', #613, 1000.000000000000000 ) ;
#2077=CARTESIAN_POINT ( 'NONE',  ( -68.99615306438109030, 17.10311908166270456, -167.1454815528550739 ) ) ;
#2079=DIRECTION ( 'NONE',  ( 0.3420201433256444545, 0.9396926207859171987, -0.000000000000000000 ) ) ;
#2081=PLANE ( 'NONE',  #7307 ) ;
#2082=DIRECTION ( 'NONE',  ( 0.000000000000000000, 1.000000000000000000, 0.000000000000000000 ) ) ;
#2086=DIRECTION ( 'NONE',  ( -0.9396926207859084279, 0.3420201433256686574, 1.086737899652989892E-16 ) ) ;
#2088=PLANE ( 'NONE',  #6821 ) ;
#2089=VERTEX_POINT ( 'NONE', #10740 ) ;
#2090=VECTOR ( 'NONE', #6349, 1000.000000000000000 ) ;
#2094=LINE ( 'NONE', #4984, #4533 ) ;
#2095=ORIENTED_EDGE ( 'NONE', *, *, #4863, .T. ) ;
#2096=DIRECTION ( 'NONE',  ( 0.000000000000000000, 0.000000000000000000, 1.000000000000000000 ) ) ;
#2097=VECTOR ( 'NONE', #3251, 1000.000000000000000 ) ;
#2098=FACE_OUTER_BOUND ( 'NONE', #1017, .T. ) ;
#2109=ORIENTED_EDGE ( 'NONE', *, *, #14412, .F. ) ;
#2113=ADVANCED_FACE ( 'NONE', ( #2233 ), #16628, .T. ) ;
#2115=ORIENTED_EDGE ( 'NONE', *, *, #8256, .F. ) ;
#2116=DIRECTION ( 'NONE',  ( 0.000000000000000000, 0.000000000000000000, -1.000000000000000000 ) ) ;
#2119=ORIENTED_EDGE ( 'NONE', *, *, #16116, .T. ) ;
#2122=CARTESIAN_POINT ( 'NONE',  ( -68.99615306438089135, 67.98345733813025049, -167.1454815528550739 ) ) ;
#2128=LINE ( 'NONE', #636, #11201 ) ;
#2133=EDGE_LOOP ( 'NONE', ( #7653, #4068, #17292, #12384 ) ) ;
#2136=DIRECTION ( 'NONE',  ( -0.004825104377941397994, -0.9999883591161159435, 5.580147892302267848E-19 ) ) ;
#2140=CARTESIAN_POINT ( 'NONE',  ( -71.24615306438073503, 129.3815214545637104, -167.1454815528550739 ) ) ;
#2141=CARTESIAN_POINT ( 'NONE',  ( -68.99615306438070661, 118.2489397381302467, 15.00000000000006928 ) ) ;
#2142=CARTESIAN_POINT ( 'NONE',  ( -71.24615306438084872, 94.82400230456377699, -15.00000000000001421 ) ) ;
#2144=ORIENTED_EDGE ( 'NONE', *, *, #3, .T. ) ;
#2151=VECTOR ( 'NONE', #5320, 1000.000000000000000 ) ;
#2152=CARTESIAN_POINT ( 'NONE',  ( -71.24615306438073503, 128.4926507152292459, 15.00000000000006928 ) ) ;
#2153=ORIENTED_EDGE ( 'NONE', *, *, #6537, .F. ) ;
#2154=ADVANCED_FACE ( 'NONE', ( #9168 ), #13460, .T. ) ;
#2155=ORIENTED_EDGE ( 'NONE', *, *, #8376, .F. ) ;
#2157=VECTOR ( 'NONE', #3561, 1000.000000000000000 ) ;
#2159=CARTESIAN_POINT ( 'NONE',  ( -71.24615306438086293, 101.1071876045637055, -15.00000000000001421 ) ) ;
#2160=LINE ( 'NONE', #7686, #15678 ) ;
#2163=VECTOR ( 'NONE', #3558, 1000.000000000000000 ) ;
#2165=ORIENTED_EDGE ( 'NONE', *, *, #9280, .T. ) ;
#2166=EDGE_CURVE ( 'NONE', #15084, #12932, #645, .T. ) ;
#2167=CARTESIAN_POINT ( 'NONE',  ( -68.99615306438100504, 42.85071613813029501, -167.1454815528550739 ) ) ;
#2168=CARTESIAN_POINT ( 'NONE',  ( -71.24615306438080609, 110.5319655545637403, -167.1454815528550739 ) ) ;
#2174=ORIENTED_EDGE ( 'NONE', *, *, #4199, .T. ) ;
#2179=VECTOR ( 'NONE', #649, 1000.000000000000000 ) ;
#2183=ORIENTED_EDGE ( 'NONE', *, *, #2073, .T. ) ;
#2186=EDGE_CURVE ( 'NONE', #6852, #11754, #7944, .T. ) ;
#2197=VECTOR ( 'NONE', #722, 1000.000000000000114 ) ;
#2198=CARTESIAN_POINT ( 'NONE',  ( -68.99615306438097662, 61.08541618166268705, 15.00000000000006928 ) ) ;
#2200=ORIENTED_EDGE ( 'NONE', *, *, #7616, .F. ) ;
#2201=DIRECTION ( 'NONE',  ( 0.000000000000000000, 1.000000000000000000, 0.000000000000000000 ) ) ;
#2204=AXIS2_PLACEMENT_3D ( 'NONE', #13352, #8877, #11943 ) ;
#2208=CARTESIAN_POINT ( 'NONE',  ( -68.99615306438074924, 121.3905323881302962, -167.1454815528550739 ) ) ;
#2214=ORIENTED_EDGE ( 'NONE', *, *, #4450, .F. ) ;
#2215=VECTOR ( 'NONE', #12400, 1000.000000000000000 ) ;
#2217=LINE ( 'NONE', #16616, #4948 ) ;
#2228=CARTESIAN_POINT ( 'NONE',  ( -68.99615306438111872, 14.57638228813026871, 15.00000000000006928 ) ) ;
#2230=ORIENTED_EDGE ( 'NONE', *, *, #704, .F. ) ;
#2231=VERTEX_POINT ( 'NONE', #15135 ) ;
#2233=FACE_OUTER_BOUND ( 'NONE', #6669, .T. ) ;
#2234=VECTOR ( 'NONE', #4103, 1000.000000000000000 ) ;
#2237=AXIS2_PLACEMENT_3D ( 'NONE', #12474, #11059, #16746 ) ;
#2239=CARTESIAN_POINT ( 'NONE',  ( -70.27900850916093134, -47.21335801510345220, -15.00000000000001599 ) ) ;
#2241=DIRECTION ( 'NONE',  ( 0.000000000000000000, 1.000000000000000000, 0.000000000000000000 ) ) ;
#2244=ORIENTED_EDGE ( 'NONE', *, *, #5261, .F. ) ;
#2245=DIRECTION ( 'NONE',  ( 0.000000000000000000, 1.000000000000000000, 0.000000000000000000 ) ) ;
#2249=AXIS2_PLACEMENT_3D ( 'NONE', #1277, #9879, #13042 ) ;
#2252=FACE_OUTER_BOUND ( 'NONE', #17882, .T. ) ;
#2253=ORIENTED_EDGE ( 'NONE', *, *, #16029, .F. ) ;
#2254=ORIENTED_EDGE ( 'NONE', *, *, #3450, .T. ) ;
#2261=DIRECTION ( 'NONE',  ( 0.000000000000000000, 0.000000000000000000, -1.000000000000000000 ) ) ;
#2263=CARTESIAN_POINT ( 'NONE',  ( -71.24615306438106188, 34.24487121522926003, 15.00000000000006928 ) ) ;
#2264=CARTESIAN_POINT ( 'NONE',  ( -70.27900850916086029, -2.213358015103419341, 15.00000000000006928 ) ) ;
#2265=CARTESIAN_POINT ( 'NONE',  ( -71.24615306438100504, 53.98329785456373742, -167.1454815528550739 ) ) ;
#2268=FACE_OUTER_BOUND ( 'NONE', #1954, .T. ) ;
#2270=DIRECTION ( 'NONE',  ( 0.000000000000000000, 1.000000000000000000, 0.000000000000000000 ) ) ;
#2274=LINE ( 'NONE', #15279, #11732 ) ;
#2278=VERTEX_POINT ( 'NONE', #9910 ) ;
#2281=ADVANCED_FACE ( 'NONE', ( #2705 ), #1121, .T. ) ;
#2286=ADVANCED_FACE ( 'NONE', ( #12449 ), #7020, .T. ) ;
#2290=ORIENTED_EDGE ( 'NONE', *, *, #13858, .T. ) ;
#2294=ORIENTED_EDGE ( 'NONE', *, *, #13854, .T. ) ;
#2297=VERTEX_POINT ( 'NONE', #5408 ) ;
#2298=EDGE_CURVE ( 'NONE', #17894, #16077, #2615, .T. ) ;
#2309=DIRECTION ( 'NONE',  ( 0.000000000000000000, 1.000000000000000000, 0.000000000000000000 ) ) ;
#2313=DIRECTION ( 'NONE',  ( 0.3420201433256481738, 0.9396926207859158664, -0.000000000000000000 ) ) ;
#2315=VERTEX_POINT ( 'NONE', #4459 ) ;
#2323=LINE ( 'NONE', #15048, #6891 ) ;
#2324=DIRECTION ( 'NONE',  ( 0.000000000000000000, 1.000000000000000000, 0.000000000000000000 ) ) ;
#2332=DIRECTION ( 'NONE',  ( 0.000000000000000000, 0.000000000000000000, -1.000000000000000000 ) ) ;
#2336=EDGE_LOOP ( 'NONE', ( #8107, #15470, #9093, #6408 ) ) ;
#2338=CARTESIAN_POINT ( 'NONE',  ( -71.24615306438087714, 66.54966845456374358, 15.00000000000006928 ) ) ;
#2339=PLANE ( 'NONE',  #12656 ) ;
#2344=CARTESIAN_POINT ( 'NONE',  ( -68.99615306438080609, 105.0677132816627051, 15.00000000000006928 ) ) ;
#2345=ORIENTED_EDGE ( 'NONE', *, *, #14096, .T. ) ;
#2346=LINE ( 'NONE', #2167, #5422 ) ;
#2347=DIRECTION ( 'NONE',  ( 0.9396926207859043201, 0.3420201433256802037, 4.890320548438427212E-16 ) ) ;
#2354=CARTESIAN_POINT ( 'NONE',  ( -68.99615306438094819, 70.51019413166270056, -15.00000000000001421 ) ) ;
#2355=ORIENTED_EDGE ( 'NONE', *, *, #16481, .F. ) ;
#2357=EDGE_LOOP ( 'NONE', ( #11397, #13604, #10066, #13559 ) ) ;
#2361=DIRECTION ( 'NONE',  ( 0.000000000000000000, 1.000000000000000000, 0.000000000000000000 ) ) ;
#2368=CARTESIAN_POINT ( 'NONE',  ( -68.99615306438089135, 86.21815738166266385, -167.1454815528550739 ) ) ;
#2374=VERTEX_POINT ( 'NONE', #15791 ) ;
#2376=VECTOR ( 'NONE', #8342, 1000.000000000000000 ) ;
#2380=ORIENTED_EDGE ( 'NONE', *, *, #10405, .T. ) ;
#2384=DIRECTION ( 'NONE',  ( -0.9396926207859158664, 0.3420201433256481738, 0.000000000000000000 ) ) ;
#2386=ORIENTED_EDGE ( 'NONE', *, *, #2186, .F. ) ;
#2388=CARTESIAN_POINT ( 'NONE',  ( -71.24615306438079188, 88.54081700456376325, 15.00000000000006928 ) ) ;
#2393=ORIENTED_EDGE ( 'NONE', *, *, #14584, .T. ) ;
#2394=CARTESIAN_POINT ( 'NONE',  ( -68.99615306438094819, 70.51019413166270056, 15.00000000000006928 ) ) ;
#2396=DIRECTION ( 'NONE',  ( 1.000000000000000000, 0.000000000000000000, 0.000000000000000000 ) ) ;
#2397=FACE_OUTER_BOUND ( 'NONE', #4607, .T. ) ;
#2399=ORIENTED_EDGE ( 'NONE', *, *, #4688, .F. ) ;
#2402=ADVANCED_FACE ( 'NONE', ( #80 ), #4547, .T. ) ;
#2404=CARTESIAN_POINT ( 'NONE',  ( -68.99615306438106188, 23.38630438166270054, -15.00000000000001421 ) ) ;
#2406=VECTOR ( 'NONE', #1225, 1000.000000000000114 ) ;
#2407=VERTEX_POINT ( 'NONE', #11763 ) ;
#2413=ORIENTED_EDGE ( 'NONE', *, *, #1475, .F. ) ;
#2419=CARTESIAN_POINT ( 'NONE',  ( -68.99615306438101925, 17.71797493813025781, 15.00000000000006928 ) ) ;
#2420=DIRECTION ( 'NONE',  ( -0.9396926207859084279, 0.3420201433256686574, -4.890320548438448905E-16 ) ) ;
#2422=CARTESIAN_POINT ( 'NONE',  ( -68.99615306438086293, 93.11619853813030545, -15.00000000000001421 ) ) ;
#2428=LINE ( 'NONE', #5131, #4251 ) ;
#2432=LINE ( 'NONE', #15244, #1527 ) ;
#2433=VERTEX_POINT ( 'NONE', #6125 ) ;
#2434=VECTOR ( 'NONE', #5211, 1000.000000000000000 ) ;
#2436=LINE ( 'NONE', #3646, #14886 ) ;
#2437=EDGE_LOOP ( 'NONE', ( #11266, #13234, #13523, #9074 ) ) ;
#2441=ORIENTED_EDGE ( 'NONE', *, *, #17055, .T. ) ;
#2443=DIRECTION ( 'NONE',  ( 0.000000000000000000, 1.000000000000000000, 0.000000000000000000 ) ) ;
#2444=DIRECTION ( 'NONE',  ( 0.000000000000000000, 0.000000000000000000, -1.000000000000000000 ) ) ;
#2446=VECTOR ( 'NONE', #1011, 1000.000000000000000 ) ;
#2448=PLANE ( 'NONE',  #2237 ) ;
#2454=ORIENTED_EDGE ( 'NONE', *, *, #13495, .F. ) ;
#2455=DIRECTION ( 'NONE',  ( 0.000000000000000000, 0.000000000000000000, 1.000000000000000000 ) ) ;
#2459=ORIENTED_EDGE ( 'NONE', *, *, #11119, .T. ) ;
#2465=VECTOR ( 'NONE', #18294, 1000.000000000000000 ) ;
#2469=ORIENTED_EDGE ( 'NONE', *, *, #16993, .T. ) ;
#2478=ORIENTED_EDGE ( 'NONE', *, *, #9167, .T. ) ;
#2479=PLANE ( 'NONE',  #11044 ) ;
#2482=VECTOR ( 'NONE', #7749, 1000.000000000000000 ) ;
#2487=ORIENTED_EDGE ( 'NONE', *, *, #16152, .F. ) ;
#2488=VECTOR ( 'NONE', #5761, 1000.000000000000000 ) ;
#2492=EDGE_CURVE ( 'NONE', #12417, #10310, #7283, .T. ) ;
#2500=CARTESIAN_POINT ( 'NONE',  ( -68.99615306438077766, 117.6340838816626899, 15.00000000000006928 ) ) ;
#2505=FACE_OUTER_BOUND ( 'NONE', #10827, .T. ) ;
#2507=CARTESIAN_POINT ( 'NONE',  ( -68.99615306438083451, 102.5409764881302692, -167.1454815528550739 ) ) ;
#2510=FACE_OUTER_BOUND ( 'NONE', #11346, .T. ) ;
#2512=VERTEX_POINT ( 'NONE', #7452 ) ;
#2516=EDGE_CURVE ( 'NONE', #2231, #11979, #17457, .T. ) ;
#2529=DIRECTION ( 'NONE',  ( 0.9396926207859148672, 0.3420201433256507273, 4.890320548438483418E-16 ) ) ;
#2533=ORIENTED_EDGE ( 'NONE', *, *, #7319, .T. ) ;
#2535=EDGE_CURVE ( 'NONE', #9465, #1454, #13347, .T. ) ;
#2537=EDGE_CURVE ( 'NONE', #18088, #11181, #3799, .T. ) ;
#2538=VERTEX_POINT ( 'NONE', #16607 ) ;
#2539=EDGE_CURVE ( 'NONE', #12123, #16319, #619, .T. ) ;
#2541=DIRECTION ( 'NONE',  ( 0.000000000000000000, 0.000000000000000000, 1.000000000000000000 ) ) ;
#2542=LINE ( 'NONE', #9456, #13117 ) ;
#2546=VECTOR ( 'NONE', #13082, 1000.000000000000000 ) ;
#2547=VECTOR ( 'NONE', #13470, 1000.000000000000000 ) ;
#2555=DIRECTION ( 'NONE',  ( 0.000000000000000000, 0.000000000000000000, -1.000000000000000000 ) ) ;
#2556=LINE ( 'NONE', #4053, #10533 ) ;
#2558=DIRECTION ( 'NONE',  ( 0.9396926207859084279, 0.3420201433256686574, -1.086737899652989892E-16 ) ) ;
#2561=DIRECTION ( 'NONE',  ( -0.9396926207859093161, 0.3420201433256661594, 1.086737899652990878E-16 ) ) ;
#2564=ORIENTED_EDGE ( 'NONE', *, *, #18180, .F. ) ;
#2565=DIRECTION ( 'NONE',  ( 0.3420201433256444545, -0.9396926207859171987, 0.000000000000000000 ) ) ;
#2566=VECTOR ( 'NONE', #14567, 1000.000000000000000 ) ;
#2567=CARTESIAN_POINT ( 'NONE',  ( -71.24615306438089135, 82.25763170456374951, -167.1454815528550739 ) ) ;
#2574=VECTOR ( 'NONE', #18223, 1000.000000000000000 ) ;
#2576=CARTESIAN_POINT ( 'NONE',  ( -71.24615306438073503, 128.4926507152292459, -15.00000000000001421 ) ) ;
#2577=VERTEX_POINT ( 'NONE', #5096 ) ;
#2578=ORIENTED_EDGE ( 'NONE', *, *, #11481, .T. ) ;
#2588=ORIENTED_EDGE ( 'NONE', *, *, #9820, .F. ) ;
#2590=CARTESIAN_POINT ( 'NONE',  ( -68.99615306438094819, 64.22700883166265839, -15.00000000000001421 ) ) ;
#2591=ORIENTED_EDGE ( 'NONE', *, *, #3525, .F. ) ;
#2593=ORIENTED_EDGE ( 'NONE', *, *, #15561, .F. ) ;
#2598=CARTESIAN_POINT ( 'NONE',  ( -68.99615306438077766, 111.3508985816626335, -167.1454815528550739 ) ) ;
#2600=DIRECTION ( 'NONE',  ( 0.000000000000000000, 0.000000000000000000, -1.000000000000000000 ) ) ;
#2601=ORIENTED_EDGE ( 'NONE', *, *, #560, .F. ) ;
#2602=ADVANCED_FACE ( 'NONE', ( #12038 ), #10813, .T. ) ;
#2603=CARTESIAN_POINT ( 'NONE',  ( -71.24615306438080609, 109.6430948152292189, 15.00000000000006928 ) ) ;
#2605=LINE ( 'NONE', #1112, #15405 ) ;
#2608=EDGE_LOOP ( 'NONE', ( #4885, #10142, #8906, #11620 ) ) ;
#2609=DIRECTION ( 'NONE',  ( 0.000000000000000000, 1.000000000000000000, 0.000000000000000000 ) ) ;
#2610=CARTESIAN_POINT ( 'NONE',  ( -68.99615306438072082, 130.2004544816626890, 15.00000000000006928 ) ) ;
#2611=DIRECTION ( 'NONE',  ( -0.9396926207859069846, 0.3420201433256723766, -4.890320548438442003E-16 ) ) ;
#2613=VERTEX_POINT ( 'NONE', #18013 ) ;
#2615=LINE ( 'NONE', #8313, #6675 ) ;
#2617=LINE ( 'NONE', #2419, #174 ) ;
#2621=EDGE_CURVE ( 'NONE', #15787, #14076, #16508, .T. ) ;
#2625=ORIENTED_EDGE ( 'NONE', *, *, #14181, .F. ) ;
#2626=FACE_OUTER_BOUND ( 'NONE', #17993, .T. ) ;
#2630=CARTESIAN_POINT ( 'NONE',  ( -68.99615306438077766, 111.3508985816626335, -15.00000000000001421 ) ) ;
#2631=ORIENTED_EDGE ( 'NONE', *, *, #3655, .T. ) ;
#2639=PLANE ( 'NONE',  #6340 ) ;
#2640=EDGE_CURVE ( 'NONE', #11938, #13177, #7818, .T. ) ;
#2642=DIRECTION ( 'NONE',  ( 0.000000000000000000, 0.000000000000000000, 1.000000000000000000 ) ) ;
#2648=VECTOR ( 'NONE', #7974, 1000.000000000000114 ) ;
#2649=EDGE_LOOP ( 'NONE', ( #3464, #7315, #8248, #10385 ) ) ;
#2654=ORIENTED_EDGE ( 'NONE', *, *, #1622, .T. ) ;
#2656=ORIENTED_EDGE ( 'NONE', *, *, #3673, .F. ) ;
#2659=CARTESIAN_POINT ( 'NONE',  ( -71.24615306438090556, 63.40807580456378645, 15.00000000000006928 ) ) ;
#2660=DIRECTION ( 'NONE',  ( 0.000000000000000000, 0.000000000000000000, 1.000000000000000000 ) ) ;
#2661=ORIENTED_EDGE ( 'NONE', *, *, #12027, .F. ) ;
#2662=ORIENTED_EDGE ( 'NONE', *, *, #7620, .F. ) ;
#2664=DIRECTION ( 'NONE',  ( 0.000000000000000000, 1.000000000000000000, 0.000000000000000000 ) ) ;
#2667=ORIENTED_EDGE ( 'NONE', *, *, #7976, .T. ) ;
#2668=PLANE ( 'NONE',  #14664 ) ;
#2675=AXIS2_PLACEMENT_3D ( 'NONE', #15951, #17437, #6110 ) ;
#2677=ORIENTED_EDGE ( 'NONE', *, *, #7820, .T. ) ;
#2681=CARTESIAN_POINT ( 'NONE',  ( -68.99615306438100504, 45.99230878813026635, -15.00000000000001421 ) ) ;
#2685=CARTESIAN_POINT ( 'NONE',  ( -68.99615306438077766, 124.5321250381302747, 15.00000000000006928 ) ) ;
#2689=CARTESIAN_POINT ( 'NONE',  ( -68.99615306438113294, -1.131580961869758761, 15.00000000000006928 ) ) ;
#2694=PLANE ( 'NONE',  #5736 ) ;
#2695=ORIENTED_EDGE ( 'NONE', *, *, #2298, .T. ) ;
#2697=DIRECTION ( 'NONE',  ( -0.9396926207859103153, 0.3420201433256635504, 1.086737899652991987E-16 ) ) ;
#2698=DIRECTION ( 'NONE',  ( 0.000000000000000000, 0.000000000000000000, 1.000000000000000000 ) ) ;
#2701=AXIS2_PLACEMENT_3D ( 'NONE', #14597, #10673, #557 ) ;
#2702=ADVANCED_FACE ( 'NONE', ( #7084 ), #11104, .T. ) ;
#2703=VERTEX_POINT ( 'NONE', #15409 ) ;
#2704=AXIS2_PLACEMENT_3D ( 'NONE', #12165, #13845, #11966 ) ;
#2705=FACE_OUTER_BOUND ( 'NONE', #1326, .T. ) ;
#2711=ORIENTED_EDGE ( 'NONE', *, *, #5283, .T. ) ;
#2718=AXIS2_PLACEMENT_3D ( 'NONE', #8535, #6930, #14242 ) ;
#2719=DIRECTION ( 'NONE',  ( 1.000000000000000000, 0.000000000000000000, 0.000000000000000000 ) ) ;
#2720=ORIENTED_EDGE ( 'NONE', *, *, #4266, .F. ) ;
#2722=DIRECTION ( 'NONE',  ( 0.000000000000000000, 0.000000000000000000, 1.000000000000000000 ) ) ;
#2723=ORIENTED_EDGE ( 'NONE', *, *, #6624, .F. ) ;
#2724=ORIENTED_EDGE ( 'NONE', *, *, #13713, .T. ) ;
#2726=ORIENTED_EDGE ( 'NONE', *, *, #1275, .F. ) ;
#2727=VECTOR ( 'NONE', #12412, 1000.000000000000000 ) ;
#2731=LINE ( 'NONE', #15906, #15205 ) ;
#2732=EDGE_CURVE ( 'NONE', #4878, #17628, #3984, .T. ) ;
#2737=VERTEX_POINT ( 'NONE', #18409 ) ;
#2745=ORIENTED_EDGE ( 'NONE', *, *, #11252, .F. ) ;
#2750=DIRECTION ( 'NONE',  ( -0.9396926207859084279, 0.3420201433256686574, 0.000000000000000000 ) ) ;
#2752=EDGE_CURVE ( 'NONE', #6089, #14417, #16984, .T. ) ;
#2753=ORIENTED_EDGE ( 'NONE', *, *, #15986, .F. ) ;
#2761=ORIENTED_EDGE ( 'NONE', *, *, #1627, .T. ) ;
#2766=CARTESIAN_POINT ( 'NONE',  ( -68.99615306438087714, 55.41708673813025854, 15.00000000000006928 ) ) ;
#2770=VECTOR ( 'NONE', #10254, 1000.000000000000000 ) ;
#2774=LINE ( 'NONE', #2869, #9746 ) ;
#2782=CARTESIAN_POINT ( 'NONE',  ( -71.24615306438117557, 3.717815454563750954, -167.1454815528550739 ) ) ;
#2784=EDGE_CURVE ( 'NONE', #9825, #13777, #7258, .T. ) ;
#2785=VECTOR ( 'NONE', #16964, 1000.000000000000000 ) ;
#2789=LINE ( 'NONE', #5387, #4291 ) ;
#2790=LINE ( 'NONE', #7090, #11775 ) ;
#2792=LINE ( 'NONE', #5391, #9581 ) ;
#2793=VECTOR ( 'NONE', #11700, 1000.000000000000000 ) ;
#2795=DIRECTION ( 'NONE',  ( 0.000000000000000000, 0.000000000000000000, -1.000000000000000000 ) ) ;
#2798=CARTESIAN_POINT ( 'NONE',  ( -68.99615306438106188, 26.52789703166272162, 15.00000000000006928 ) ) ;
#2799=CARTESIAN_POINT ( 'NONE',  ( -71.24615306438120399, 0.5762228045637918239, -167.1454815528550739 ) ) ;
#2801=DIRECTION ( 'NONE',  ( 0.000000000000000000, 1.000000000000000000, 0.000000000000000000 ) ) ;
#2803=ORIENTED_EDGE ( 'NONE', *, *, #7483, .F. ) ;
#2804=ORIENTED_EDGE ( 'NONE', *, *, #17315, .T. ) ;
#2810=CARTESIAN_POINT ( 'NONE',  ( -68.99615306438074924, 120.7756765316626542, 15.00000000000006928 ) ) ;
#2812=ORIENTED_EDGE ( 'NONE', *, *, #7926, .T. ) ;
#2817=CARTESIAN_POINT ( 'NONE',  ( -68.99615306438111872, 7.678341131662685726, -167.1454815528550739 ) ) ;
#2821=VECTOR ( 'NONE', #4174, 1000.000000000000000 ) ;
#2822=DIRECTION ( 'NONE',  ( 0.3420201433256649937, -0.9396926207859097602, 0.000000000000000000 ) ) ;
#2825=DIRECTION ( 'NONE',  ( 0.000000000000000000, 1.000000000000000000, 0.000000000000000000 ) ) ;
#2826=ORIENTED_EDGE ( 'NONE', *, *, #14984, .T. ) ;
#2827=EDGE_LOOP ( 'NONE', ( #16884, #5507, #2478, #6522 ) ) ;
#2829=ORIENTED_EDGE ( 'NONE', *, *, #13086, .T. ) ;
#2830=VECTOR ( 'NONE', #1846, 1000.000000000000000 ) ;
#2832=DIRECTION ( 'NONE',  ( 0.9396926207859171987, 0.3420201433256444545, 0.000000000000000000 ) ) ;
#2833=CARTESIAN_POINT ( 'NONE',  ( -71.24615306438070661, 141.9478920545637664, 15.00000000000006928 ) ) ;
#2842=CARTESIAN_POINT ( 'NONE',  ( -68.99615306438089135, 83.07656473166271383, -167.1454815528550739 ) ) ;
#2843=CARTESIAN_POINT ( 'NONE',  ( -71.24615306438120399, 0.5762228045637918239, -167.1454815528550739 ) ) ;
#2845=VECTOR ( 'NONE', #10436, 1000.000000000000000 ) ;
#2846=VECTOR ( 'NONE', #7707, 1000.000000000000000 ) ;
#2850=EDGE_LOOP ( 'NONE', ( #5631, #7903, #1550, #6173 ) ) ;
#2853=AXIS2_PLACEMENT_3D ( 'NONE', #16279, #3469, #10214 ) ;
#2854=ORIENTED_EDGE ( 'NONE', *, *, #4143, .F. ) ;
#2856=VECTOR ( 'NONE', #6153, 1000.000000000000000 ) ;
#2860=ORIENTED_EDGE ( 'NONE', *, *, #18204, .T. ) ;
#2863=ADVANCED_FACE ( 'NONE', ( #12494 ), #8175, .T. ) ;
#2864=PLANE ( 'NONE',  #12332 ) ;
#2869=CARTESIAN_POINT ( 'NONE',  ( -68.99615306438063556, 137.0984956381302879, 15.00000000000006928 ) ) ;
#2871=EDGE_LOOP ( 'NONE', ( #12399, #16730, #1652, #15681 ) ) ;
#2873=VERTEX_POINT ( 'NONE', #11179 ) ;
#2874=EDGE_CURVE ( 'NONE', #6902, #11029, #5178, .T. ) ;
#2878=ADVANCED_FACE ( 'NONE', ( #6861 ), #16667, .T. ) ;
#2881=DIRECTION ( 'NONE',  ( 0.000000000000000000, 1.000000000000000000, 0.000000000000000000 ) ) ;
#2885=ADVANCED_FACE ( 'NONE', ( #15278 ), #4071, .T. ) ;
#2886=CARTESIAN_POINT ( 'NONE',  ( -71.24615306438109030, 25.70896400456376796, -15.00000000000001421 ) ) ;
#2887=LINE ( 'NONE', #4446, #5435 ) ;
#2891=FACE_OUTER_BOUND ( 'NONE', #13092, .T. ) ;
#2892=EDGE_CURVE ( 'NONE', #6902, #6728, #1165, .T. ) ;
#2895=EDGE_CURVE ( 'NONE', #6955, #10161, #6962, .T. ) ;
#2896=DIRECTION ( 'NONE',  ( -0.9396926207859068736, 0.3420201433256726542, 0.000000000000000000 ) ) ;
#2897=ORIENTED_EDGE ( 'NONE', *, *, #2784, .T. ) ;
#2899=EDGE_CURVE ( 'NONE', #4662, #14342, #16588, .T. ) ;
#2900=DIRECTION ( 'NONE',  ( 0.3420201433256701007, -0.9396926207859078728, 0.000000000000000000 ) ) ;
#2901=ORIENTED_EDGE ( 'NONE', *, *, #8952, .T. ) ;
#2907=FACE_OUTER_BOUND ( 'NONE', #6040, .T. ) ;
#2912=LINE ( 'NONE', #7204, #15592 ) ;
#2913=LINE ( 'NONE', #11250, #16427 ) ;
#2915=CARTESIAN_POINT ( 'NONE',  ( -71.24615306438080609, 115.9262801152292042, -15.00000000000001421 ) ) ;
#2916=LINE ( 'NONE', #196, #17336 ) ;
#2920=DIRECTION ( 'NONE',  ( 0.9396926207859135349, 0.3420201433256547241, -1.086737899652995685E-16 ) ) ;
#2923=LINE ( 'NONE', #7221, #1835 ) ;
#2925=LINE ( 'NONE', #7398, #11989 ) ;
#2928=CARTESIAN_POINT ( 'NONE',  ( -71.24615306438111872, 18.53690796522925055, 15.00000000000006928 ) ) ;
#2933=VERTEX_POINT ( 'NONE', #13984 ) ;
#2934=DIRECTION ( 'NONE',  ( 0.000000000000000000, 1.000000000000000000, 0.000000000000000000 ) ) ;
#2936=PLANE ( 'NONE',  #16182 ) ;
#2941=EDGE_LOOP ( 'NONE', ( #12024, #1626, #8222, #4413 ) ) ;
#2943=DIRECTION ( 'NONE',  ( 0.000000000000000000, 0.000000000000000000, 1.000000000000000000 ) ) ;
#2945=DIRECTION ( 'NONE',  ( 0.000000000000000000, 1.000000000000000000, 0.000000000000000000 ) ) ;
#2946=EDGE_LOOP ( 'NONE', ( #1692, #2804, #8014, #17354 ) ) ;
#2947=DIRECTION ( 'NONE',  ( 1.000000000000000000, 0.000000000000000000, 0.000000000000000000 ) ) ;
#2959=CARTESIAN_POINT ( 'NONE',  ( -68.99615306438093398, 42.85071613813026659, 15.00000000000006928 ) ) ;
#2967=ORIENTED_EDGE ( 'NONE', *, *, #9394, .F. ) ;
#2970=LINE ( 'NONE', #1477, #6272 ) ;
#2971=EDGE_LOOP ( 'NONE', ( #13344, #13626, #11676, #4312 ) ) ;
#2972=EDGE_CURVE ( 'NONE', #4999, #13143, #10222, .T. ) ;
#2974=EDGE_CURVE ( 'NONE', #8996, #17731, #3200, .T. ) ;
#2980=DIRECTION ( 'NONE',  ( 0.000000000000000000, 1.000000000000000000, 0.000000000000000000 ) ) ;
#2985=DIRECTION ( 'NONE',  ( 0.3420201433256612189, -0.9396926207859112035, 0.000000000000000000 ) ) ;
#2986=DIRECTION ( 'NONE',  ( 0.000000000000000000, 1.000000000000000000, 0.000000000000000000 ) ) ;
#2992=ORIENTED_EDGE ( 'NONE', *, *, #3112, .F. ) ;
#2993=ADVANCED_FACE ( 'NONE', ( #4508 ), #10049, .T. ) ;
#2994=LINE ( 'NONE', #15445, #1790 ) ;
#2995=VECTOR ( 'NONE', #8546, 1000.000000000000000 ) ;
#2996=CARTESIAN_POINT ( 'NONE',  ( -68.99615306438094819, 71.12504998813029999, -15.00000000000001421 ) ) ;
#2999=EDGE_CURVE ( 'NONE', #5330, #5342, #13049, .T. ) ;
#3001=EDGE_CURVE ( 'NONE', #13376, #5348, #8739, .T. ) ;
#3003=ORIENTED_EDGE ( 'NONE', *, *, #13710, .T. ) ;
#3008=EDGE_CURVE ( 'NONE', #13332, #15988, #296, .T. ) ;
#3011=FACE_OUTER_BOUND ( 'NONE', #4358, .T. ) ;
#3015=EDGE_LOOP ( 'NONE', ( #1478, #13689, #12574, #8836 ) ) ;
#3016=DIRECTION ( 'NONE',  ( 0.9396926207859145341, 0.3420201433256520596, 0.000000000000000000 ) ) ;
#3020=ORIENTED_EDGE ( 'NONE', *, *, #16481, .T. ) ;
#3022=AXIS2_PLACEMENT_3D ( 'NONE', #243, #168, #5933 ) ;
#3026=DIRECTION ( 'NONE',  ( 0.000000000000000000, 0.000000000000000000, 1.000000000000000000 ) ) ;
#3036=DIRECTION ( 'NONE',  ( 0.000000000000000000, 1.000000000000000000, 0.000000000000000000 ) ) ;
#3039=VECTOR ( 'NONE', #8549, 1000.000000000000000 ) ;
#3043=DIRECTION ( 'NONE',  ( -0.9396926207859088720, 0.3420201433256675472, -4.890320548438450878E-16 ) ) ;
#3045=ORIENTED_EDGE ( 'NONE', *, *, #6673, .F. ) ;
#3058=CARTESIAN_POINT ( 'NONE',  ( -68.99615306438100504, 48.51904558166270220, -167.1454815528550739 ) ) ;
#3061=ORIENTED_EDGE ( 'NONE', *, *, #5283, .F. ) ;
#3062=VECTOR ( 'NONE', #10050, 1000.000000000000000 ) ;
#3064=CARTESIAN_POINT ( 'NONE',  ( -68.99615306438094819, 55.41708673813027985, -167.1454815528550739 ) ) ;
#3071=ORIENTED_EDGE ( 'NONE', *, *, #12937, .F. ) ;
#3075=ORIENTED_EDGE ( 'NONE', *, *, #9770, .T. ) ;
#3083=CARTESIAN_POINT ( 'NONE',  ( -71.24615306438103346, 40.52805651522925245, 15.00000000000006928 ) ) ;
#3084=VECTOR ( 'NONE', #4411, 1000.000000000000000 ) ;
#3090=EDGE_CURVE ( 'NONE', #15763, #4483, #15666, .T. ) ;
#3091=EDGE_CURVE ( 'NONE', #16133, #15911, #2160, .T. ) ;
#3096=CARTESIAN_POINT ( 'NONE',  ( -68.99615306438111872, 13.96152643166267993, -15.00000000000001421 ) ) ;
#3098=VECTOR ( 'NONE', #12885, 1000.000000000000000 ) ;
#3099=VECTOR ( 'NONE', #10921, 1000.000000000000000 ) ;
#3104=FACE_OUTER_BOUND ( 'NONE', #8926, .T. ) ;
#3106=EDGE_CURVE ( 'NONE', #4868, #11956, #4685, .T. ) ;
#3107=CARTESIAN_POINT ( 'NONE',  ( -68.99615306438089135, 83.07656473166271383, 15.00000000000006928 ) ) ;
#3109=DIRECTION ( 'NONE',  ( 0.3420201433256686574, -0.9396926207859084279, 0.000000000000000000 ) ) ;
#3112=EDGE_CURVE ( 'NONE', #4238, #15911, #11986, .T. ) ;
#3113=ORIENTED_EDGE ( 'NONE', *, *, #1188, .F. ) ;
#3118=VERTEX_POINT ( 'NONE', #3560 ) ;
#3120=CARTESIAN_POINT ( 'NONE',  ( -68.99615306438117557, 4.536748481662661092, -167.1454815528550739 ) ) ;
#3121=LINE ( 'NONE', #14347, #3062 ) ;
#3123=ORIENTED_EDGE ( 'NONE', *, *, #242, .T. ) ;
#3126=VECTOR ( 'NONE', #4581, 1000.000000000000000 ) ;
#3127=DIRECTION ( 'NONE',  ( 0.000000000000000000, 0.000000000000000000, 1.000000000000000000 ) ) ;
#3131=AXIS2_PLACEMENT_3D ( 'NONE', #6194, #17615, #1651 ) ;
#3132=ORIENTED_EDGE ( 'NONE', *, *, #9786, .F. ) ;
#3133=EDGE_CURVE ( 'NONE', #7544, #881, #1892, .T. ) ;
#3135=EDGE_CURVE ( 'NONE', #5784, #12176, #10400, .T. ) ;
#3139=VECTOR ( 'NONE', #15929, 1000.000000000000000 ) ;
#3141=VECTOR ( 'NONE', #10571, 1000.000000000000114 ) ;
#3147=LINE ( 'NONE', #4367, #10144 ) ;
#3148=LINE ( 'NONE', #15860, #12291 ) ;
#3161=ORIENTED_EDGE ( 'NONE', *, *, #9186, .F. ) ;
#3162=ORIENTED_EDGE ( 'NONE', *, *, #3781, .T. ) ;
#3166=CARTESIAN_POINT ( 'NONE',  ( -68.99615306438094819, 64.22700883166265839, 15.00000000000006928 ) ) ;
#3171=DIRECTION ( 'NONE',  ( 0.3420201433256649937, 0.9396926207859097602, -0.000000000000000000 ) ) ;
#3179=VERTEX_POINT ( 'NONE', #12090 ) ;
#3184=DIRECTION ( 'NONE',  ( 1.000000000000000000, 0.000000000000000000, 0.000000000000000000 ) ) ;
#3186=LINE ( 'NONE', #281, #12301 ) ;
#3191=CARTESIAN_POINT ( 'NONE',  ( -68.99615306438117557, 1.395155831662693524, -15.00000000000001421 ) ) ;
#3193=DIRECTION ( 'NONE',  ( 0.000000000000000000, 0.000000000000000000, 1.000000000000000000 ) ) ;
#3197=VERTEX_POINT ( 'NONE', #8254 ) ;
#3198=EDGE_CURVE ( 'NONE', #16032, #15619, #18260, .T. ) ;
#3199=LINE ( 'NONE', #17234, #3139 ) ;
#3200=LINE ( 'NONE', #13125, #5506 ) ;
#3201=CARTESIAN_POINT ( 'NONE',  ( -68.99615306438086293, 92.50134268166266338, -15.00000000000001421 ) ) ;
#3202=ORIENTED_EDGE ( 'NONE', *, *, #1512, .T. ) ;
#3204=EDGE_CURVE ( 'NONE', #14281, #13941, #9549, .T. ) ;
#3205=LINE ( 'NONE', #10406, #11096 ) ;
#3206=DIRECTION ( 'NONE',  ( 0.000000000000000000, 1.000000000000000000, 0.000000000000000000 ) ) ;
#3207=CARTESIAN_POINT ( 'NONE',  ( -71.24615306438080609, 115.9262801152292042, -167.1454815528550739 ) ) ;
#3211=VERTEX_POINT ( 'NONE', #956 ) ;
#3217=ADVANCED_FACE ( 'NONE', ( #6754 ), #1061, .T. ) ;
#3218=ORIENTED_EDGE ( 'NONE', *, *, #6166, .T. ) ;
#3220=LINE ( 'NONE', #10421, #10009 ) ;
#3223=EDGE_LOOP ( 'NONE', ( #15642, #13398, #13303, #18519 ) ) ;
#3225=LINE ( 'NONE', #1650, #17649 ) ;
#3227=VERTEX_POINT ( 'NONE', #5538 ) ;
#3228=ADVANCED_FACE ( 'NONE', ( #6839 ), #18073, .T. ) ;
#3229=PLANE ( 'NONE',  #3022 ) ;
#3230=CARTESIAN_POINT ( 'NONE',  ( -71.24615306438114715, 12.25372266522925457, -167.1454815528550739 ) ) ;
#3232=ORIENTED_EDGE ( 'NONE', *, *, #6624, .T. ) ;
#3233=CARTESIAN_POINT ( 'NONE',  ( -71.24615306438094819, 68.80239036522922902, -15.00000000000001421 ) ) ;
#3234=VECTOR ( 'NONE', #9115, 1000.000000000000000 ) ;
#3235=CARTESIAN_POINT ( 'NONE',  ( -71.24615306438076345, 132.5231141045637457, -167.1454815528550739 ) ) ;
#3236=VERTEX_POINT ( 'NONE', #12471 ) ;
#3237=ORIENTED_EDGE ( 'NONE', *, *, #6537, .T. ) ;
#3242=DIRECTION ( 'NONE',  ( 0.000000000000000000, 0.000000000000000000, -1.000000000000000000 ) ) ;
#3244=CARTESIAN_POINT ( 'NONE',  ( -71.24615306438089135, 85.39922435456371375, -167.1454815528550739 ) ) ;
#3249=DIRECTION ( 'NONE',  ( 0.9396926207859084279, 0.3420201433256686574, 0.000000000000000000 ) ) ;
#3251=DIRECTION ( 'NONE',  ( 0.000000000000000000, 1.000000000000000000, 0.000000000000000000 ) ) ;
#3259=VECTOR ( 'NONE', #14561, 999.9999999999998863 ) ;
#3260=EDGE_LOOP ( 'NONE', ( #5457, #11693, #5313, #13019 ) ) ;
#3261=CARTESIAN_POINT ( 'NONE',  ( -68.99615306438091977, 73.65178678166269322, 15.00000000000006928 ) ) ;
#3263=CARTESIAN_POINT ( 'NONE',  ( -68.99615306438076345, 96.25779118813024127, 15.00000000000006928 ) ) ;
#3264=CARTESIAN_POINT ( 'NONE',  ( -94.45685920050698314, -2.213358015103445098, -15.00000000000001421 ) ) ;
#3268=ORIENTED_EDGE ( 'NONE', *, *, #232, .T. ) ;
#3273=DIRECTION ( 'NONE',  ( 0.000000000000000000, 1.000000000000000000, 0.000000000000000000 ) ) ;
#3274=VERTEX_POINT ( 'NONE', #5334 ) ;
#3277=ORIENTED_EDGE ( 'NONE', *, *, #9487, .F. ) ;
#3280=EDGE_CURVE ( 'NONE', #5742, #12056, #8153, .T. ) ;
#3282=DIRECTION ( 'NONE',  ( 0.000000000000000000, 0.000000000000000000, -1.000000000000000000 ) ) ;
#3283=CARTESIAN_POINT ( 'NONE',  ( -68.99615306438082030, 83.69142058813027063, 15.00000000000006928 ) ) ;
#3284=LINE ( 'NONE', #17586, #4839 ) ;
#3285=ORIENTED_EDGE ( 'NONE', *, *, #16606, .T. ) ;
#3286=ORIENTED_EDGE ( 'NONE', *, *, #12003, .T. ) ;
#3288=CARTESIAN_POINT ( 'NONE',  ( -71.24615306438067819, 144.2006139652292518, 15.00000000000006928 ) ) ;
#3290=CARTESIAN_POINT ( 'NONE',  ( -71.24615306438070661, 135.6647067545637242, -15.00000000000001421 ) ) ;
#3292=VECTOR ( 'NONE', #14577, 1000.000000000000000 ) ;
#3293=ADVANCED_FACE ( 'NONE', ( #6940 ), #5251, .T. ) ;
#3294=FACE_OUTER_BOUND ( 'NONE', #11784, .T. ) ;
#3295=ORIENTED_EDGE ( 'NONE', *, *, #1425, .T. ) ;
#3297=EDGE_LOOP ( 'NONE', ( #12103, #7207, #13916, #8729 ) ) ;
#3298=ORIENTED_EDGE ( 'NONE', *, *, #15306, .T. ) ;
#3302=EDGE_CURVE ( 'NONE', #1161, #12615, #854, .T. ) ;
#3304=ORIENTED_EDGE ( 'NONE', *, *, #13286, .T. ) ;
#3308=CARTESIAN_POINT ( 'NONE',  ( -71.24615306438070661, 147.3422066152292871, -15.00000000000001421 ) ) ;
#3313=PLANE ( 'NONE',  #1558 ) ;
#3317=EDGE_CURVE ( 'NONE', #16328, #8559, #14330, .T. ) ;
#3318=LINE ( 'NONE', #12129, #17174 ) ;
#3319=EDGE_CURVE ( 'NONE', #8820, #2089, #4320, .T. ) ;
#3320=LINE ( 'NONE', #11660, #14370 ) ;
#3321=VECTOR ( 'NONE', #1797, 1000.000000000000000 ) ;
#3322=VECTOR ( 'NONE', #381, 1000.000000000000000 ) ;
#3324=ORIENTED_EDGE ( 'NONE', *, *, #5025, .T. ) ;
#3332=VERTEX_POINT ( 'NONE', #11342 ) ;
#3333=CARTESIAN_POINT ( 'NONE',  ( -71.24615306438086293, 100.2183168652291982, -15.00000000000001421 ) ) ;
#3334=VECTOR ( 'NONE', #10433, 1000.000000000000000 ) ;
#3342=ADVANCED_FACE ( 'NONE', ( #8 ), #15739, .T. ) ;
#3343=ORIENTED_EDGE ( 'NONE', *, *, #15306, .F. ) ;
#3347=ORIENTED_EDGE ( 'NONE', *, *, #123, .F. ) ;
#3348=ORIENTED_EDGE ( 'NONE', *, *, #7773, .T. ) ;
#3353=LINE ( 'NONE', #4952, #2482 ) ;
#3363=AXIS2_PLACEMENT_3D ( 'NONE', #4496, #7399, #3016 ) ;
#3365=PLANE ( 'NONE',  #1510 ) ;
#3370=VECTOR ( 'NONE', #814, 1000.000000000000114 ) ;
#3371=VERTEX_POINT ( 'NONE', #278 ) ;
#3374=LINE ( 'NONE', #14791, #18483 ) ;
#3377=LINE ( 'NONE', #10401, #4561 ) ;
#3379=CARTESIAN_POINT ( 'NONE',  ( -71.24615306438117557, 6.859408104563785358, 15.00000000000006928 ) ) ;
#3385=ORIENTED_EDGE ( 'NONE', *, *, #1707, .F. ) ;
#3386=DIRECTION ( 'NONE',  ( 0.000000000000000000, 0.000000000000000000, -1.000000000000000000 ) ) ;
#3394=AXIS2_PLACEMENT_3D ( 'NONE', #13069, #11740, #158 ) ;
#3396=CARTESIAN_POINT ( 'NONE',  ( -71.24615306438076345, 126.2399288045637462, 15.00000000000006928 ) ) ;
#3398=EDGE_CURVE ( 'NONE', #6648, #11131, #2731, .T. ) ;
#3399=AXIS2_PLACEMENT_3D ( 'NONE', #3207, #405, #16097 ) ;
#3402=DIRECTION ( 'NONE',  ( -0.9396926207859097602, 0.3420201433256649937, 1.086737899652991371E-16 ) ) ;
#3411=DIRECTION ( 'NONE',  ( 0.000000000000000000, 1.000000000000000000, 0.000000000000000000 ) ) ;
#3421=DIRECTION ( 'NONE',  ( 0.3420201433256663814, -0.9396926207859093161, 0.000000000000000000 ) ) ;
#3426=FACE_OUTER_BOUND ( 'NONE', #17703, .T. ) ;
#3428=CARTESIAN_POINT ( 'NONE',  ( -71.24615306438070661, 134.7758360152292312, 15.00000000000006928 ) ) ;
#3430=ORIENTED_EDGE ( 'NONE', *, *, #2732, .F. ) ;
#3432=LINE ( 'NONE', #14837, #6279 ) ;
#3433=AXIS2_PLACEMENT_3D ( 'NONE', #16968, #13992, #9681 ) ;
#3439=VERTEX_POINT ( 'NONE', #1511 ) ;
#3441=EDGE_CURVE ( 'NONE', #2873, #1167, #14511, .T. ) ;
#3443=DIRECTION ( 'NONE',  ( 0.000000000000000000, 1.000000000000000000, 0.000000000000000000 ) ) ;
#3444=CARTESIAN_POINT ( 'NONE',  ( -68.99615306438067819, 142.7668250816626596, -167.1454815528550739 ) ) ;
#3445=VERTEX_POINT ( 'NONE', #5625 ) ;
#3450=EDGE_CURVE ( 'NONE', #15750, #11410, #12843, .T. ) ;
#3461=PLANE ( 'NONE',  #11652 ) ;
#3464=ORIENTED_EDGE ( 'NONE', *, *, #7976, .F. ) ;
#3465=DIRECTION ( 'NONE',  ( 0.000000000000000000, 0.000000000000000000, -1.000000000000000000 ) ) ;
#3466=CARTESIAN_POINT ( 'NONE',  ( -71.24615306438107609, 13.14259340456380620, 15.00000000000006928 ) ) ;
#3468=ORIENTED_EDGE ( 'NONE', *, *, #7953, .F. ) ;
#3469=DIRECTION ( 'NONE',  ( 1.000000000000000000, 0.000000000000000000, 0.000000000000000000 ) ) ;
#3475=CARTESIAN_POINT ( 'NONE',  ( -94.45685920050698314, -2.213358015103445098, -167.1454815528550739 ) ) ;
#3477=CARTESIAN_POINT ( 'NONE',  ( -71.24615306438070661, 138.8062994045637311, -167.1454815528550739 ) ) ;
#3478=EDGE_LOOP ( 'NONE', ( #11382, #11430, #5476, #16623 ) ) ;
#3479=CARTESIAN_POINT ( 'NONE',  ( -71.24615306438069240, 187.7866419848965052, -15.00000000000001421 ) ) ;
#3481=ORIENTED_EDGE ( 'NONE', *, *, #8702, .T. ) ;
#3482=DIRECTION ( 'NONE',  ( 0.000000000000000000, 1.000000000000000000, 0.000000000000000000 ) ) ;
#3483=DIRECTION ( 'NONE',  ( 0.000000000000000000, 1.000000000000000000, 0.000000000000000000 ) ) ;
#3484=DIRECTION ( 'NONE',  ( 0.3420201433256854218, 0.9396926207859023217, -0.000000000000000000 ) ) ;
#3487=CARTESIAN_POINT ( 'NONE',  ( -68.99615306438072082, 133.3420471316626958, -167.1454815528550739 ) ) ;
#3489=CARTESIAN_POINT ( 'NONE',  ( -71.24615306438076345, 122.2094654152292037, 15.00000000000006928 ) ) ;
#3492=ORIENTED_EDGE ( 'NONE', *, *, #8170, .F. ) ;
#3508=ORIENTED_EDGE ( 'NONE', *, *, #342, .T. ) ;
#3513=CARTESIAN_POINT ( 'NONE',  ( -71.24615306438111872, 21.67850061522927518, 15.00000000000006928 ) ) ;
#3514=DIRECTION ( 'NONE',  ( 0.000000000000000000, 1.000000000000000000, 0.000000000000000000 ) ) ;
#3516=ORIENTED_EDGE ( 'NONE', *, *, #8266, .F. ) ;
#3518=FACE_OUTER_BOUND ( 'NONE', #6492, .T. ) ;
#3519=CARTESIAN_POINT ( 'NONE',  ( -71.24615306438080609, 107.3903729045637192, 15.00000000000006928 ) ) ;
#3522=ORIENTED_EDGE ( 'NONE', *, *, #7873, .T. ) ;
#3523=CARTESIAN_POINT ( 'NONE',  ( -71.24615306438076345, 123.0983361545637109, -167.1454815528550739 ) ) ;
#3525=EDGE_CURVE ( 'NONE', #15440, #6184, #10380, .T. ) ;
#3530=ORIENTED_EDGE ( 'NONE', *, *, #13071, .F. ) ;
#3531=ORIENTED_EDGE ( 'NONE', *, *, #1076, .T. ) ;
#3532=VECTOR ( 'NONE', #1591, 1000.000000000000000 ) ;
#3536=EDGE_CURVE ( 'NONE', #1454, #8559, #4093, .T. ) ;
#3540=CARTESIAN_POINT ( 'NONE',  ( -68.99615306438082030, 96.25779118813026969, -15.00000000000001421 ) ) ;
#3541=LINE ( 'NONE', #2142, #13306 ) ;
#3544=VERTEX_POINT ( 'NONE', #11109 ) ;
#3547=FACE_OUTER_BOUND ( 'NONE', #4272, .T. ) ;
#3551=CARTESIAN_POINT ( 'NONE',  ( -71.24615306438103346, 40.52805651522925245, -15.00000000000001421 ) ) ;
#3558=DIRECTION ( 'NONE',  ( 0.000000000000000000, 1.000000000000000000, 0.000000000000000000 ) ) ;
#3559=VECTOR ( 'NONE', #9971, 1000.000000000000114 ) ;
#3560=CARTESIAN_POINT ( 'NONE',  ( -68.99615306438067819, 143.3816809381303585, -15.00000000000001421 ) ) ;
#3561=DIRECTION ( 'NONE',  ( 0.000000000000000000, 1.000000000000000000, 0.000000000000000000 ) ) ;
#3562=ORIENTED_EDGE ( 'NONE', *, *, #2621, .T. ) ;
#3574=CARTESIAN_POINT ( 'NONE',  ( -68.99615306438091977, 73.65178678166269322, -15.00000000000001421 ) ) ;
#3579=DIRECTION ( 'NONE',  ( 0.000000000000000000, 0.000000000000000000, 1.000000000000000000 ) ) ;
#3580=LINE ( 'NONE', #13515, #13508 ) ;
#3581=ORIENTED_EDGE ( 'NONE', *, *, #5346, .F. ) ;
#3587=ORIENTED_EDGE ( 'NONE', *, *, #17055, .F. ) ;
#3591=LINE ( 'NONE', #9312, #9715 ) ;
#3595=AXIS2_PLACEMENT_3D ( 'NONE', #1306, #15712, #7181 ) ;
#3610=PLANE ( 'NONE',  #8080 ) ;
#3612=PLANE ( 'NONE',  #4637 ) ;
#3615=VECTOR ( 'NONE', #3483, 1000.000000000000000 ) ;
#3617=CARTESIAN_POINT ( 'NONE',  ( -94.45685920050698314, -47.21335801510345220, -15.00000000000001421 ) ) ;
#3620=ADVANCED_FACE ( 'NONE', ( #3990 ), #4278, .T. ) ;
#3626=CARTESIAN_POINT ( 'NONE',  ( -68.99615306438109030, 17.71797493813028268, -167.1454815528550739 ) ) ;
#3627=ORIENTED_EDGE ( 'NONE', *, *, #11797, .T. ) ;
#3628=VECTOR ( 'NONE', #4692, 1000.000000000000000 ) ;
#3629=VECTOR ( 'NONE', #6365, 1000.000000000000000 ) ;
#3631=DIRECTION ( 'NONE',  ( 0.000000000000000000, 1.000000000000000000, 0.000000000000000000 ) ) ;
#3636=VERTEX_POINT ( 'NONE', #18216 ) ;
#3641=EDGE_CURVE ( 'NONE', #1745, #12836, #15600, .T. ) ;
#3642=EDGE_CURVE ( 'NONE', #4254, #8291, #18313, .T. ) ;
#3643=VECTOR ( 'NONE', #11654, 1000.000000000000000 ) ;
#3646=CARTESIAN_POINT ( 'NONE',  ( -71.24615306438074924, 123.0983361545637109, -15.00000000000001421 ) ) ;
#3647=ORIENTED_EDGE ( 'NONE', *, *, #1800, .T. ) ;
#3655=EDGE_CURVE ( 'NONE', #5451, #17731, #8582, .T. ) ;
#3657=FACE_OUTER_BOUND ( 'NONE', #13859, .T. ) ;
#3658=EDGE_CURVE ( 'NONE', #5717, #3274, #3890, .T. ) ;
#3664=EDGE_CURVE ( 'NONE', #10905, #14281, #11210, .T. ) ;
#3670=VERTEX_POINT ( 'NONE', #8496 ) ;
#3671=LINE ( 'NONE', #9383, #12559 ) ;
#3673=EDGE_CURVE ( 'NONE', #18141, #12144, #11301, .T. ) ;
#3674=VECTOR ( 'NONE', #2980, 1000.000000000000000 ) ;
#3678=EDGE_LOOP ( 'NONE', ( #13136, #965, #15348, #4080 ) ) ;
#3679=EDGE_CURVE ( 'NONE', #6562, #1454, #10344, .T. ) ;
#3683=ORIENTED_EDGE ( 'NONE', *, *, #5261, .T. ) ;
#3684=CARTESIAN_POINT ( 'NONE',  ( -71.24615306438107609, 28.85055665456374285, -15.00000000000001421 ) ) ;
#3690=LINE ( 'NONE', #12018, #16151 ) ;
#3691=EDGE_CURVE ( 'NONE', #10695, #14578, #1649, .T. ) ;
#3699=CARTESIAN_POINT ( 'NONE',  ( -68.99615306438090556, 61.70027203813025807, 15.00000000000006928 ) ) ;
#3701=ORIENTED_EDGE ( 'NONE', *, *, #9610, .T. ) ;
#3702=DIRECTION ( 'NONE',  ( 0.000000000000000000, 0.000000000000000000, 1.000000000000000000 ) ) ;
#3707=ORIENTED_EDGE ( 'NONE', *, *, #10319, .F. ) ;
#3711=CARTESIAN_POINT ( 'NONE',  ( -71.24615306438096241, 44.55851990456374523, 15.00000000000006928 ) ) ;
#3713=ORIENTED_EDGE ( 'NONE', *, *, #3133, .F. ) ;
#3720=DIRECTION ( 'NONE',  ( 0.000000000000000000, 0.000000000000000000, -1.000000000000000000 ) ) ;
#3722=VERTEX_POINT ( 'NONE', #238 ) ;
#3726=CARTESIAN_POINT ( 'NONE',  ( -71.24615306438116136, 6.859408104563791575, -15.00000000000001421 ) ) ;
#3728=ORIENTED_EDGE ( 'NONE', *, *, #16106, .T. ) ;
#3729=CARTESIAN_POINT ( 'NONE',  ( -68.99615306438070661, 137.0984956381303164, -167.1454815528550739 ) ) ;
#3733=ORIENTED_EDGE ( 'NONE', *, *, #5841, .T. ) ;
#3736=ORIENTED_EDGE ( 'NONE', *, *, #3995, .T. ) ;
#3741=LINE ( 'NONE', #7849, #10560 ) ;
#3744=LINE ( 'NONE', #936, #1364 ) ;
#3747=LINE ( 'NONE', #13569, #18017 ) ;
#3753=ORIENTED_EDGE ( 'NONE', *, *, #3090, .T. ) ;
#3762=LINE ( 'NONE', #11062, #12623 ) ;
#3763=LINE ( 'NONE', #10022, #9014 ) ;
#3766=CARTESIAN_POINT ( 'NONE',  ( -68.99615306438117557, 1.395155831662692192, -167.1454815528550739 ) ) ;
#3770=EDGE_LOOP ( 'NONE', ( #9714, #2144, #9930, #5737 ) ) ;
#3771=EDGE_CURVE ( 'NONE', #4613, #16809, #17341, .T. ) ;
#3773=ORIENTED_EDGE ( 'NONE', *, *, #2054, .T. ) ;
#3776=LINE ( 'NONE', #15567, #2785 ) ;
#3777=ADVANCED_FACE ( 'NONE', ( #14719 ), #4529, .T. ) ;
#3778=ORIENTED_EDGE ( 'NONE', *, *, #4784, .F. ) ;
#3781=EDGE_CURVE ( 'NONE', #10136, #3332, #8763, .T. ) ;
#3783=DIRECTION ( 'NONE',  ( -0.9396926207859097602, 0.3420201433256649381, -4.890320548438455808E-16 ) ) ;
#3785=DIRECTION ( 'NONE',  ( 0.9396926207859097602, 0.3420201433256649937, 0.000000000000000000 ) ) ;
#3794=ORIENTED_EDGE ( 'NONE', *, *, #12315, .T. ) ;
#3795=EDGE_CURVE ( 'NONE', #6928, #1519, #10151, .T. ) ;
#3796=EDGE_CURVE ( 'NONE', #15896, #17894, #3147, .T. ) ;
#3798=ORIENTED_EDGE ( 'NONE', *, *, #5433, .T. ) ;
#3799=LINE ( 'NONE', #7642, #9671 ) ;
#3808=FACE_OUTER_BOUND ( 'NONE', #14290, .T. ) ;
#3811=FACE_OUTER_BOUND ( 'NONE', #10155, .T. ) ;
#3813=ORIENTED_EDGE ( 'NONE', *, *, #2874, .F. ) ;
#3817=CARTESIAN_POINT ( 'NONE',  ( -68.99615306438097662, 57.94382353166266597, -15.00000000000001421 ) ) ;
#3818=ORIENTED_EDGE ( 'NONE', *, *, #13838, .T. ) ;
#3831=CARTESIAN_POINT ( 'NONE',  ( -71.24615306438080609, 104.2487802545637408, 15.00000000000006928 ) ) ;
#3834=CARTESIAN_POINT ( 'NONE',  ( -71.24615306438111872, 21.67850061522927518, 15.00000000000006928 ) ) ;
#3842=CARTESIAN_POINT ( 'NONE',  ( -68.99615306438080609, 108.2093059316626693, -15.00000000000001421 ) ) ;
#3843=CARTESIAN_POINT ( 'NONE',  ( -71.24615306438104767, 19.42577870456378619, 15.00000000000006928 ) ) ;
#3844=DIRECTION ( 'NONE',  ( 0.9396926207859158664, 0.3420201433256481738, 0.000000000000000000 ) ) ;
#3853=ORIENTED_EDGE ( 'NONE', *, *, #14093, .T. ) ;
#3854=CARTESIAN_POINT ( 'NONE',  ( -68.99615306438076345, 115.1073470881302541, -15.00000000000001421 ) ) ;
#3859=VECTOR ( 'NONE', #14982, 1000.000000000000000 ) ;
#3860=VERTEX_POINT ( 'NONE', #11571 ) ;
#3863=DIRECTION ( 'NONE',  ( 0.9396926207859171987, 0.3420201433256445100, 4.890320548438495251E-16 ) ) ;
#3867=DIRECTION ( 'NONE',  ( 0.000000000000000000, 0.000000000000000000, 1.000000000000000000 ) ) ;
#3868=EDGE_CURVE ( 'NONE', #11029, #4091, #15106, .T. ) ;
#3869=CARTESIAN_POINT ( 'NONE',  ( -71.24615306438073503, 128.4926507152292459, -15.00000000000001421 ) ) ;
#3870=EDGE_LOOP ( 'NONE', ( #6331, #1737, #3798, #5123 ) ) ;
#3873=ORIENTED_EDGE ( 'NONE', *, *, #14964, .T. ) ;
#3877=CARTESIAN_POINT ( 'NONE',  ( -68.99615306438111872, 7.678341131662685726, 15.00000000000006928 ) ) ;
#3886=LINE ( 'NONE', #18308, #15661 ) ;
#3888=VECTOR ( 'NONE', #15909, 1000.000000000000000 ) ;
#3890=LINE ( 'NONE', #18413, #4445 ) ;
#3895=ORIENTED_EDGE ( 'NONE', *, *, #8390, .F. ) ;
#3896=DIRECTION ( 'NONE',  ( -0.9396926207859068736, 0.3420201433256725987, -4.890320548438441017E-16 ) ) ;
#3898=DIRECTION ( 'NONE',  ( 1.000000000000000000, 0.000000000000000000, 0.000000000000000000 ) ) ;
#3899=ADVANCED_FACE ( 'NONE', ( #15397 ), #2479, .T. ) ;
#3900=CARTESIAN_POINT ( 'NONE',  ( -71.24615306438106188, 37.38646386522923137, -167.1454815528550739 ) ) ;
#3903=VECTOR ( 'NONE', #14581, 1000.000000000000114 ) ;
#3904=PLANE ( 'NONE',  #6103 ) ;
#3907=EDGE_CURVE ( 'NONE', #3636, #4573, #8287, .T. ) ;
#3910=AXIS2_PLACEMENT_3D ( 'NONE', #10079, #7365, #7531 ) ;
#3918=CARTESIAN_POINT ( 'NONE',  ( -68.99615306438080609, 105.0677132816627051, 15.00000000000006928 ) ) ;
#3926=CARTESIAN_POINT ( 'NONE',  ( -71.24615306438109030, 28.85055665456373575, -15.00000000000001421 ) ) ;
#3930=DIRECTION ( 'NONE',  ( 0.9396926207859185309, 0.3420201433256406798, 4.890320548438501168E-16 ) ) ;
#3933=ORIENTED_EDGE ( 'NONE', *, *, #792, .T. ) ;
#3938=CARTESIAN_POINT ( 'NONE',  ( -68.99615306438100504, 42.23586028166270978, -15.00000000000001421 ) ) ;
#3940=LINE ( 'NONE', #12380, #8150 ) ;
#3941=AXIS2_PLACEMENT_3D ( 'NONE', #18324, #8105, #5493 ) ;
#3945=ORIENTED_EDGE ( 'NONE', *, *, #13961, .F. ) ;
#3949=ORIENTED_EDGE ( 'NONE', *, *, #17366, .F. ) ;
#3951=VECTOR ( 'NONE', #7908, 1000.000000000000000 ) ;
#3952=FACE_OUTER_BOUND ( 'NONE', #8891, .T. ) ;
#3953=ORIENTED_EDGE ( 'NONE', *, *, #15339, .F. ) ;
#3958=VECTOR ( 'NONE', #10997, 1000.000000000000000 ) ;
#3960=CARTESIAN_POINT ( 'NONE',  ( -71.24615306438106188, 34.24487121522926003, 15.00000000000006928 ) ) ;
#3961=CARTESIAN_POINT ( 'NONE',  ( -71.24615306438070661, 135.6647067545637242, 15.00000000000006928 ) ) ;
#3962=ORIENTED_EDGE ( 'NONE', *, *, #15355, .F. ) ;
#3964=DIRECTION ( 'NONE',  ( 0.000000000000000000, 0.000000000000000000, 1.000000000000000000 ) ) ;
#3966=ORIENTED_EDGE ( 'NONE', *, *, #12235, .F. ) ;
#3967=AXIS2_PLACEMENT_3D ( 'NONE', #3477, #9191, #14881 ) ;
#3970=DIRECTION ( 'NONE',  ( 1.000000000000000000, 0.000000000000000000, 0.000000000000000000 ) ) ;
#3971=ORIENTED_EDGE ( 'NONE', *, *, #16066, .T. ) ;
#3976=CARTESIAN_POINT ( 'NONE',  ( -71.24615306438066398, 145.0894847045637732, -15.00000000000001421 ) ) ;
#3982=ADVANCED_FACE ( 'NONE', ( #18111 ), #308, .T. ) ;
#3984=LINE ( 'NONE', #2782, #18354 ) ;
#3986=ORIENTED_EDGE ( 'NONE', *, *, #1269, .F. ) ;
#3990=FACE_OUTER_BOUND ( 'NONE', #2827, .T. ) ;
#3995=EDGE_CURVE ( 'NONE', #10484, #12065, #5915, .T. ) ;
#3997=DIRECTION ( 'NONE',  ( 0.9396926207859084279, 0.3420201433256686574, 0.000000000000000000 ) ) ;
#3999=EDGE_CURVE ( 'NONE', #10310, #15702, #1543, .T. ) ;
#4001=DIRECTION ( 'NONE',  ( -0.9396926207859093161, 0.3420201433256661594, 0.000000000000000000 ) ) ;
#4002=ORIENTED_EDGE ( 'NONE', *, *, #16212, .T. ) ;
#4004=CARTESIAN_POINT ( 'NONE',  ( -68.99615306438091977, 77.40823528813029952, -167.1454815528550739 ) ) ;
#4005=PLANE ( 'NONE',  #14942 ) ;
#4006=VECTOR ( 'NONE', #13324, 1000.000000000000000 ) ;
#4009=VECTOR ( 'NONE', #1215, 1000.000000000000000 ) ;
#4012=VECTOR ( 'NONE', #12560, 999.9999999999998863 ) ;
#4013=ADVANCED_FACE ( 'NONE', ( #14276 ), #8474, .T. ) ;
#4015=ADVANCED_FACE ( 'NONE', ( #6004 ), #11379, .T. ) ;
#4017=ORIENTED_EDGE ( 'NONE', *, *, #2067, .T. ) ;
#4021=VERTEX_POINT ( 'NONE', #11560 ) ;
#4025=CARTESIAN_POINT ( 'NONE',  ( -68.99615306438107609, 17.71797493813027558, -15.00000000000001421 ) ) ;
#4030=AXIS2_PLACEMENT_3D ( 'NONE', #6837, #4132, #11260 ) ;
#4039=VECTOR ( 'NONE', #2934, 1000.000000000000000 ) ;
#4043=ORIENTED_EDGE ( 'NONE', *, *, #5121, .T. ) ;
#4047=AXIS2_PLACEMENT_3D ( 'NONE', #4468, #10181, #8789 ) ;
#4050=LINE ( 'NONE', #11340, #9112 ) ;
#4053=CARTESIAN_POINT ( 'NONE',  ( -68.99615306438111872, 13.96152643166267993, -167.1454815528550739 ) ) ;
#4055=CARTESIAN_POINT ( 'NONE',  ( -71.24615306438097662, 60.26648315456372984, -167.1454815528550739 ) ) ;
#4058=VECTOR ( 'NONE', #1883, 1000.000000000000000 ) ;
#4061=LINE ( 'NONE', #3854, #8143 ) ;
#4063=AXIS2_PLACEMENT_3D ( 'NONE', #14838, #17747, #732 ) ;
#4064=LINE ( 'NONE', #18087, #292 ) ;
#4065=ORIENTED_EDGE ( 'NONE', *, *, #15986, .T. ) ;
#4067=EDGE_LOOP ( 'NONE', ( #11165, #1388, #11959, #17761 ) ) ;
#4068=ORIENTED_EDGE ( 'NONE', *, *, #15071, .T. ) ;
#4069=VECTOR ( 'NONE', #16024, 1000.000000000000000 ) ;
#4070=LINE ( 'NONE', #5732, #4606 ) ;
#4071=PLANE ( 'NONE',  #1329 ) ;
#4072=CARTESIAN_POINT ( 'NONE',  ( -71.24615306438099083, 50.84170520456371634, -15.00000000000001421 ) ) ;
#4075=LINE ( 'NONE', #15478, #7216 ) ;
#4076=ORIENTED_EDGE ( 'NONE', *, *, #11481, .F. ) ;
#4078=CARTESIAN_POINT ( 'NONE',  ( -71.24615306438100504, 49.95283446522918780, 15.00000000000006928 ) ) ;
#4080=ORIENTED_EDGE ( 'NONE', *, *, #5364, .F. ) ;
#4083=EDGE_CURVE ( 'NONE', #17985, #16652, #4351, .T. ) ;
#4084=ORIENTED_EDGE ( 'NONE', *, *, #1074, .T. ) ;
#4085=PLANE ( 'NONE',  #761 ) ;
#4087=DIRECTION ( 'NONE',  ( 0.000000000000000000, 1.000000000000000000, 0.000000000000000000 ) ) ;
#4091=VERTEX_POINT ( 'NONE', #6277 ) ;
#4093=LINE ( 'NONE', #1106, #11914 ) ;
#4097=CARTESIAN_POINT ( 'NONE',  ( -71.24615306438080609, 106.5015021652292404, -15.00000000000001421 ) ) ;
#4103=DIRECTION ( 'NONE',  ( 0.000000000000000000, 1.000000000000000000, 0.000000000000000000 ) ) ;
#4104=CARTESIAN_POINT ( 'NONE',  ( -68.99615306438074924, 120.7756765316626542, -15.00000000000001421 ) ) ;
#4106=CARTESIAN_POINT ( 'NONE',  ( -68.99615306438103346, 32.81108233166271759, 15.00000000000006928 ) ) ;
#4107=ORIENTED_EDGE ( 'NONE', *, *, #13378, .T. ) ;
#4122=ADVANCED_FACE ( 'NONE', ( #684 ), #4615, .T. ) ;
#4123=CARTESIAN_POINT ( 'NONE',  ( -71.24615306438076345, 126.2399288045637462, -167.1454815528550739 ) ) ;
#4127=VERTEX_POINT ( 'NONE', #584 ) ;
#4129=EDGE_CURVE ( 'NONE', #2703, #689, #12001, .T. ) ;
#4131=ORIENTED_EDGE ( 'NONE', *, *, #16690, .F. ) ;
#4132=DIRECTION ( 'NONE',  ( 0.3420201433256481738, 0.9396926207859158664, -0.000000000000000000 ) ) ;
#4133=DIRECTION ( 'NONE',  ( 0.3420201433256663814, 0.9396926207859093161, -0.000000000000000000 ) ) ;
#4134=CARTESIAN_POINT ( 'NONE',  ( -71.24615306438086293, 90.79353891522923448, -167.1454815528550739 ) ) ;
#4135=ADVANCED_FACE ( 'NONE', ( #13503 ), #13230, .T. ) ;
#4137=LINE ( 'NONE', #2344, #12630 ) ;
#4138=ORIENTED_EDGE ( 'NONE', *, *, #17597, .T. ) ;
#4143=EDGE_CURVE ( 'NONE', #6870, #14184, #4781, .T. ) ;
#4144=ADVANCED_FACE ( 'NONE', ( #10500 ), #16196, .T. ) ;
#4145=DIRECTION ( 'NONE',  ( 0.000000000000000000, 0.000000000000000000, 1.000000000000000000 ) ) ;
#4154=CARTESIAN_POINT ( 'NONE',  ( -71.24615306438111872, 18.53690796522925055, -167.1454815528550739 ) ) ;
#4155=CARTESIAN_POINT ( 'NONE',  ( -71.24615306438083451, 97.96559495456375544, 15.00000000000006928 ) ) ;
#4161=PLANE ( 'NONE',  #11694 ) ;
#4163=CARTESIAN_POINT ( 'NONE',  ( -70.27900850916093134, -47.21335801510345220, 15.00000000000008171 ) ) ;
#4164=ORIENTED_EDGE ( 'NONE', *, *, #930, .T. ) ;
#4165=DIRECTION ( 'NONE',  ( 0.000000000000000000, 1.000000000000000000, 0.000000000000000000 ) ) ;
#4170=VECTOR ( 'NONE', #1464, 1000.000000000000000 ) ;
#4172=ORIENTED_EDGE ( 'NONE', *, *, #13629, .T. ) ;
#4174=DIRECTION ( 'NONE',  ( -0.9396926207859145341, 0.3420201433256519485, 1.086737899652996918E-16 ) ) ;
#4175=DIRECTION ( 'NONE',  ( 0.000000000000000000, 0.000000000000000000, 1.000000000000000000 ) ) ;
#4176=ORIENTED_EDGE ( 'NONE', *, *, #14943, .F. ) ;
#4179=CARTESIAN_POINT ( 'NONE',  ( -68.99615306438111872, 13.96152643166267993, -167.1454815528550739 ) ) ;
#4181=DIRECTION ( 'NONE',  ( 0.000000000000000000, 0.000000000000000000, -1.000000000000000000 ) ) ;
#4182=ORIENTED_EDGE ( 'NONE', *, *, #4222, .T. ) ;
#4184=VECTOR ( 'NONE', #1463, 1000.000000000000114 ) ;
#4185=LINE ( 'NONE', #17418, #16908 ) ;
#4187=PLANE ( 'NONE',  #10809 ) ;
#4189=DIRECTION ( 'NONE',  ( 0.000000000000000000, 0.000000000000000000, 1.000000000000000000 ) ) ;
#4190=LINE ( 'NONE', #8407, #10112 ) ;
#4191=LINE ( 'NONE', #5678, #1516 ) ;
#4193=ORIENTED_EDGE ( 'NONE', *, *, #6530, .T. ) ;
#4194=AXIS2_PLACEMENT_3D ( 'NONE', #11882, #13302, #16360 ) ;
#4196=VECTOR ( 'NONE', #13032, 1000.000000000000000 ) ;
#4199=EDGE_CURVE ( 'NONE', #17497, #2231, #13407, .T. ) ;
#4204=ORIENTED_EDGE ( 'NONE', *, *, #2537, .F. ) ;
#4206=CARTESIAN_POINT ( 'NONE',  ( -71.24615306438063556, 135.6647067545637526, 15.00000000000006928 ) ) ;
#4207=LINE ( 'NONE', #1490, #1948 ) ;
#4208=LINE ( 'NONE', #1674, #8540 ) ;
#4209=CARTESIAN_POINT ( 'NONE',  ( -68.99615306438079188, 89.97460588813025595, 15.00000000000006928 ) ) ;
#4211=VECTOR ( 'NONE', #12261, 1000.000000000000000 ) ;
#4213=VECTOR ( 'NONE', #16045, 1000.000000000000114 ) ;
#4214=CARTESIAN_POINT ( 'NONE',  ( -71.24615306438106188, 38.27533460456375281, 15.00000000000006928 ) ) ;
#4215=EDGE_LOOP ( 'NONE', ( #17213, #12397, #6703, #14035 ) ) ;
#4216=LINE ( 'NONE', #2915, #14070 ) ;
#4217=LINE ( 'NONE', #1681, #16996 ) ;
#4220=VECTOR ( 'NONE', #2943, 1000.000000000000000 ) ;
#4221=ORIENTED_EDGE ( 'NONE', *, *, #12228, .F. ) ;
#4222=EDGE_CURVE ( 'NONE', #15084, #6521, #1902, .T. ) ;
#4224=CARTESIAN_POINT ( 'NONE',  ( -71.24615306438070661, 141.9478920545637664, -167.1454815528550739 ) ) ;
#4226=CARTESIAN_POINT ( 'NONE',  ( -71.24615306438109030, 25.70896400456376796, -167.1454815528550739 ) ) ;
#4231=AXIS2_PLACEMENT_3D ( 'NONE', #7587, #4589, #5979 ) ;
#4233=CARTESIAN_POINT ( 'NONE',  ( -68.99615306438104767, 24.00116023813026089, -15.00000000000001421 ) ) ;
#4234=PLANE ( 'NONE',  #5681 ) ;
#4235=EDGE_LOOP ( 'NONE', ( #638, #9998, #9682, #5180 ) ) ;
#4238=VERTEX_POINT ( 'NONE', #7513 ) ;
#4240=ADVANCED_FACE ( 'NONE', ( #3294 ), #7612, .T. ) ;
#4241=ORIENTED_EDGE ( 'NONE', *, *, #7421, .F. ) ;
#4244=ADVANCED_FACE ( 'NONE', ( #3952 ), #9471, .T. ) ;
#4247=ORIENTED_EDGE ( 'NONE', *, *, #12937, .T. ) ;
#4250=ORIENTED_EDGE ( 'NONE', *, *, #3796, .T. ) ;
#4251=VECTOR ( 'NONE', #18350, 1000.000000000000000 ) ;
#4254=VERTEX_POINT ( 'NONE', #6668 ) ;
#4258=ADVANCED_FACE ( 'NONE', ( #2268 ), #13686, .T. ) ;
#4266=EDGE_CURVE ( 'NONE', #5703, #1230, #8166, .T. ) ;
#4268=DIRECTION ( 'NONE',  ( 0.000000000000000000, 0.000000000000000000, 1.000000000000000000 ) ) ;
#4270=ORIENTED_EDGE ( 'NONE', *, *, #8011, .T. ) ;
#4272=EDGE_LOOP ( 'NONE', ( #17189, #3627, #9483, #13001 ) ) ;
#4274=DIRECTION ( 'NONE',  ( 0.3420201433256481738, -0.9396926207859158664, 0.000000000000000000 ) ) ;
#4275=VECTOR ( 'NONE', #13637, 1000.000000000000000 ) ;
#4277=DIRECTION ( 'NONE',  ( 0.000000000000000000, 0.000000000000000000, -1.000000000000000000 ) ) ;
#4278=PLANE ( 'NONE',  #1469 ) ;
#4279=PLANE ( 'NONE',  #17353 ) ;
#4280=DIRECTION ( 'NONE',  ( 0.000000000000000000, 0.000000000000000000, 1.000000000000000000 ) ) ;
#4281=VERTEX_POINT ( 'NONE', #12288 ) ;
#4284=VECTOR ( 'NONE', #9422, 1000.000000000000000 ) ;
#4285=EDGE_CURVE ( 'NONE', #16809, #16358, #5344, .T. ) ;
#4288=VERTEX_POINT ( 'NONE', #8351 ) ;
#4289=DIRECTION ( 'NONE',  ( 0.000000000000000000, 0.000000000000000000, -1.000000000000000000 ) ) ;
#4290=LINE ( 'NONE', #2610, #6906 ) ;
#4291=VECTOR ( 'NONE', #2881, 1000.000000000000000 ) ;
#4295=ORIENTED_EDGE ( 'NONE', *, *, #8314, .T. ) ;
#4296=AXIS2_PLACEMENT_3D ( 'NONE', #5778, #8682, #13088 ) ;
#4302=CARTESIAN_POINT ( 'NONE',  ( -68.99615306438077766, 114.4924912316626688, -15.00000000000001421 ) ) ;
#4303=LINE ( 'NONE', #2817, #1565 ) ;
#4306=VECTOR ( 'NONE', #10242, 1000.000000000000000 ) ;
#4307=VECTOR ( 'NONE', #15014, 1000.000000000000114 ) ;
#4308=DIRECTION ( 'NONE',  ( 0.9396926207859097602, 0.3420201433256649937, 0.000000000000000000 ) ) ;
#4309=ORIENTED_EDGE ( 'NONE', *, *, #250, .T. ) ;
#4310=EDGE_CURVE ( 'NONE', #15152, #15440, #969, .T. ) ;
#4311=CARTESIAN_POINT ( 'NONE',  ( -68.99615306438087714, 52.27549408813020904, 15.00000000000006928 ) ) ;
#4312=ORIENTED_EDGE ( 'NONE', *, *, #6375, .F. ) ;
#4315=EDGE_CURVE ( 'NONE', #13617, #4782, #4064, .T. ) ;
#4316=VECTOR ( 'NONE', #4087, 1000.000000000000000 ) ;
#4317=AXIS2_PLACEMENT_3D ( 'NONE', #625, #4727, #13091 ) ;
#4320=LINE ( 'NONE', #4580, #1183 ) ;
#4321=CARTESIAN_POINT ( 'NONE',  ( -68.99615306438091977, 76.79337943166271430, -167.1454815528550739 ) ) ;
#4324=VECTOR ( 'NONE', #10321, 1000.000000000000000 ) ;
#4326=ORIENTED_EDGE ( 'NONE', *, *, #13063, .T. ) ;
#4327=DIRECTION ( 'NONE',  ( 0.9396926207859084279, 0.3420201433256686574, 4.890320548438448905E-16 ) ) ;
#4334=ORIENTED_EDGE ( 'NONE', *, *, #11316, .T. ) ;
#4339=DIRECTION ( 'NONE',  ( -0.9396926207859158664, 0.3420201433256481738, 1.086737899652998397E-16 ) ) ;
#4340=VECTOR ( 'NONE', #3193, 1000.000000000000000 ) ;
#4341=EDGE_LOOP ( 'NONE', ( #16627, #4710, #5829, #2244 ) ) ;
#4345=EDGE_LOOP ( 'NONE', ( #5198, #13413, #15897, #2355 ) ) ;
#4348=CARTESIAN_POINT ( 'NONE',  ( -71.24615306438114715, 15.39531531522927921, -167.1454815528550739 ) ) ;
#4351=LINE ( 'NONE', #13134, #14621 ) ;
#4358=EDGE_LOOP ( 'NONE', ( #3277, #7882, #8516, #12796 ) ) ;
#4359=EDGE_CURVE ( 'NONE', #12641, #14842, #3671, .T. ) ;
#4361=EDGE_CURVE ( 'NONE', #11131, #12093, #13040, .T. ) ;
#4364=CARTESIAN_POINT ( 'NONE',  ( -71.24615306438109030, 31.10327856522923540, 15.00000000000006928 ) ) ;
#4365=ORIENTED_EDGE ( 'NONE', *, *, #9270, .F. ) ;
#4366=FACE_OUTER_BOUND ( 'NONE', #18110, .T. ) ;
#4367=CARTESIAN_POINT ( 'NONE',  ( -71.24615306438086293, 100.2183168652291982, -15.00000000000001421 ) ) ;
#4368=DIRECTION ( 'NONE',  ( 0.000000000000000000, 0.000000000000000000, -1.000000000000000000 ) ) ;
#4369=DIRECTION ( 'NONE',  ( -0.9396926207859084279, 0.3420201433256686574, -4.890320548438448905E-16 ) ) ;
#4370=ORIENTED_EDGE ( 'NONE', *, *, #8838, .F. ) ;
#4371=ADVANCED_FACE ( 'NONE', ( #7058 ), #4234, .T. ) ;
#4372=DIRECTION ( 'NONE',  ( 0.000000000000000000, 0.000000000000000000, 1.000000000000000000 ) ) ;
#4373=CARTESIAN_POINT ( 'NONE',  ( -71.24615306438080609, 109.6430948152292189, 15.00000000000006928 ) ) ;
#4374=CARTESIAN_POINT ( 'NONE',  ( -68.99615306438111872, 20.24471173166267235, -167.1454815528550739 ) ) ;
#4378=EDGE_CURVE ( 'NONE', #4994, #18486, #8555, .T. ) ;
#4388=LINE ( 'NONE', #1487, #4009 ) ;
#4393=CARTESIAN_POINT ( 'NONE',  ( -94.45685920050698314, -47.21335801510345220, -15.00000000000001421 ) ) ;
#4394=ORIENTED_EDGE ( 'NONE', *, *, #18323, .F. ) ;
#4396=CARTESIAN_POINT ( 'NONE',  ( -71.24615306438117557, 3.717815454563750954, -15.00000000000001421 ) ) ;
#4400=VERTEX_POINT ( 'NONE', #8819 ) ;
#4402=CARTESIAN_POINT ( 'NONE',  ( -68.99615306438089135, 86.83301323813024908, 15.00000000000006928 ) ) ;
#4403=CARTESIAN_POINT ( 'NONE',  ( -71.24615306438076345, 119.0678727652292253, 15.00000000000006928 ) ) ;
#4405=CARTESIAN_POINT ( 'NONE',  ( -68.99615306438116136, 2.010011688130275420, -15.00000000000001421 ) ) ;
#4407=ORIENTED_EDGE ( 'NONE', *, *, #3679, .T. ) ;
#4408=CARTESIAN_POINT ( 'NONE',  ( -68.99615306438109030, 17.71797493813028268, 15.00000000000006928 ) ) ;
#4411=DIRECTION ( 'NONE',  ( 0.9396926207859084279, 0.3420201433256686574, 4.890320548438448905E-16 ) ) ;
#4413=ORIENTED_EDGE ( 'NONE', *, *, #5009, .F. ) ;
#4415=ORIENTED_EDGE ( 'NONE', *, *, #8830, .F. ) ;
#4417=CARTESIAN_POINT ( 'NONE',  ( -71.24615306438086293, 100.2183168652291982, 15.00000000000006928 ) ) ;
#4418=CARTESIAN_POINT ( 'NONE',  ( -71.24615306438080609, 109.6430948152292189, -167.1454815528550739 ) ) ;
#4419=CARTESIAN_POINT ( 'NONE',  ( -71.24615306438076345, 131.6342433652292243, 15.00000000000006928 ) ) ;
#4420=ORIENTED_EDGE ( 'NONE', *, *, #4595, .F. ) ;
#4422=VERTEX_POINT ( 'NONE', #2928 ) ;
#4425=DIRECTION ( 'NONE',  ( -0.9396926207859069846, 0.3420201433256723766, 1.086737899652988166E-16 ) ) ;
#4427=ORIENTED_EDGE ( 'NONE', *, *, #17272, .T. ) ;
#4430=EDGE_CURVE ( 'NONE', #15988, #6870, #14339, .T. ) ;
#4434=CARTESIAN_POINT ( 'NONE',  ( -71.24615306438086293, 90.79353891522923448, -15.00000000000001421 ) ) ;
#4442=DIRECTION ( 'NONE',  ( 0.000000000000000000, 1.000000000000000000, 0.000000000000000000 ) ) ;
#4445=VECTOR ( 'NONE', #7169, 1000.000000000000000 ) ;
#4446=CARTESIAN_POINT ( 'NONE',  ( -71.24615306438093398, 50.84170520456373765, 15.00000000000006928 ) ) ;
#4450=EDGE_CURVE ( 'NONE', #5525, #15948, #17309, .T. ) ;
#4451=DIRECTION ( 'NONE',  ( 0.000000000000000000, 0.000000000000000000, 1.000000000000000000 ) ) ;
#4457=AXIS2_PLACEMENT_3D ( 'NONE', #3487, #14892, #12105 ) ;
#4458=EDGE_CURVE ( 'NONE', #18474, #4238, #15917, .T. ) ;
#4459=CARTESIAN_POINT ( 'NONE',  ( -68.99615306438111872, 8.293196988130274505, 15.00000000000006928 ) ) ;
#4467=CARTESIAN_POINT ( 'NONE',  ( -68.99615306438094819, 70.51019413166270056, 15.00000000000006928 ) ) ;
#4468=CARTESIAN_POINT ( 'NONE',  ( -71.24615306438111872, 21.67850061522927518, -167.1454815528550739 ) ) ;
#4479=PLANE ( 'NONE',  #9567 ) ;
#4483=VERTEX_POINT ( 'NONE', #10390 ) ;
#4484=ORIENTED_EDGE ( 'NONE', *, *, #6284, .F. ) ;
#4486=LINE ( 'NONE', #17389, #7548 ) ;
#4488=ADVANCED_FACE ( 'NONE', ( #4959 ), #14866, .T. ) ;
#4489=DIRECTION ( 'NONE',  ( 0.000000000000000000, 1.000000000000000000, 0.000000000000000000 ) ) ;
#4495=LINE ( 'NONE', #9179, #1828 ) ;
#4496=CARTESIAN_POINT ( 'NONE',  ( -71.24615306438111872, 19.42577870456376132, -167.1454815528550739 ) ) ;
#4497=DIRECTION ( 'NONE',  ( 0.000000000000000000, 0.000000000000000000, 1.000000000000000000 ) ) ;
#4500=PLANE ( 'NONE',  #13024 ) ;
#4508=FACE_OUTER_BOUND ( 'NONE', #14765, .T. ) ;
#4513=CARTESIAN_POINT ( 'NONE',  ( -71.24615306438096241, 41.41692725456380941, 15.00000000000006928 ) ) ;
#4515=LINE ( 'NONE', #10230, #10042 ) ;
#4516=DIRECTION ( 'NONE',  ( -0.9396926207859022107, 0.3420201433256853663, -4.890320548438416365E-16 ) ) ;
#4518=VERTEX_POINT ( 'NONE', #16005 ) ;
#4521=ORIENTED_EDGE ( 'NONE', *, *, #9593, .F. ) ;
#4522=ADVANCED_FACE ( 'NONE', ( #9181 ), #1881, .T. ) ;
#4525=AXIS2_PLACEMENT_3D ( 'NONE', #2077, #12279, #2261 ) ;
#4529=PLANE ( 'NONE',  #2675 ) ;
#4533=VECTOR ( 'NONE', #596, 999.9999999999998863 ) ;
#4534=CARTESIAN_POINT ( 'NONE',  ( -71.24615306438097662, 56.23601976522923707, -15.00000000000001421 ) ) ;
#4535=DIRECTION ( 'NONE',  ( 0.9396926207859102043, 0.3420201433256637169, 4.890320548438457780E-16 ) ) ;
#4536=CARTESIAN_POINT ( 'NONE',  ( -68.99615306438089135, 79.93497208166267853, 15.00000000000006928 ) ) ;
#4537=ORIENTED_EDGE ( 'NONE', *, *, #3771, .T. ) ;
#4541=ADVANCED_FACE ( 'NONE', ( #3547 ), #3365, .T. ) ;
#4542=CARTESIAN_POINT ( 'NONE',  ( -68.99615306438093398, 52.27549408813023035, -15.00000000000001421 ) ) ;
#4547=PLANE ( 'NONE',  #4296 ) ;
#4549=VECTOR ( 'NONE', #6656, 1000.000000000000000 ) ;
#4553=DIRECTION ( 'NONE',  ( 0.000000000000000000, 0.000000000000000000, 1.000000000000000000 ) ) ;
#4555=ORIENTED_EDGE ( 'NONE', *, *, #5293, .T. ) ;
#4556=CARTESIAN_POINT ( 'NONE',  ( -68.99615306438120399, -1.131580961869733448, 15.00000000000006928 ) ) ;
#4559=DIRECTION ( 'NONE',  ( -0.000000000000000000, 1.000000000000000000, -0.000000000000000000 ) ) ;
#4561=VECTOR ( 'NONE', #16090, 1000.000000000000000 ) ;
#4563=PLANE ( 'NONE',  #11662 ) ;
#4564=ADVANCED_FACE ( 'NONE', ( #10309 ), #13381, .T. ) ;
#4566=EDGE_CURVE ( 'NONE', #18179, #16605, #8995, .T. ) ;
#4567=AXIS2_PLACEMENT_3D ( 'NONE', #7023, #13842, #1030 ) ;
#4569=VECTOR ( 'NONE', #2455, 1000.000000000000000 ) ;
#4571=ORIENTED_EDGE ( 'NONE', *, *, #9838, .F. ) ;
#4573=VERTEX_POINT ( 'NONE', #11806 ) ;
#4574=EDGE_CURVE ( 'NONE', #8464, #6521, #12079, .T. ) ;
#4576=EDGE_CURVE ( 'NONE', #17297, #11154, #17496, .T. ) ;
#4577=EDGE_CURVE ( 'NONE', #10506, #2278, #13207, .T. ) ;
#4579=LINE ( 'NONE', #277, #18337 ) ;
#4580=CARTESIAN_POINT ( 'NONE',  ( -71.24615306438069240, 132.5231141045637742, 15.00000000000006928 ) ) ;
#4581=DIRECTION ( 'NONE',  ( 0.000000000000000000, 1.000000000000000000, 0.000000000000000000 ) ) ;
#4582=EDGE_CURVE ( 'NONE', #16328, #17297, #9264, .T. ) ;
#4586=DIRECTION ( 'NONE',  ( 0.000000000000000000, 0.000000000000000000, -1.000000000000000000 ) ) ;
#4587=VERTEX_POINT ( 'NONE', #3191 ) ;
#4588=ADVANCED_FACE ( 'NONE', ( #9088 ), #13116, .T. ) ;
#4589=DIRECTION ( 'NONE',  ( 1.000000000000000000, 0.000000000000000000, 0.000000000000000000 ) ) ;
#4591=LINE ( 'NONE', #1976, #17314 ) ;
#4595=EDGE_CURVE ( 'NONE', #8085, #15750, #4591, .T. ) ;
#4596=ORIENTED_EDGE ( 'NONE', *, *, #11100, .T. ) ;
#4599=AXIS2_PLACEMENT_3D ( 'NONE', #7553, #15974, #17640 ) ;
#4605=LINE ( 'NONE', #15667, #14693 ) ;
#4606=VECTOR ( 'NONE', #8460, 1000.000000000000000 ) ;
#4607=EDGE_LOOP ( 'NONE', ( #4521, #6484, #901, #5629 ) ) ;
#4608=VECTOR ( 'NONE', #18115, 1000.000000000000000 ) ;
#4609=CARTESIAN_POINT ( 'NONE',  ( -68.99615306438100504, 42.85071613813029501, -167.1454815528550739 ) ) ;
#4612=CARTESIAN_POINT ( 'NONE',  ( -71.24615306438100504, 50.84170520456370923, 15.00000000000006928 ) ) ;
#4613=VERTEX_POINT ( 'NONE', #7955 ) ;
#4615=PLANE ( 'NONE',  #13735 ) ;
#4623=DIRECTION ( 'NONE',  ( 0.000000000000000000, 1.000000000000000000, 0.000000000000000000 ) ) ;
#4629=VERTEX_POINT ( 'NONE', #18247 ) ;
#4631=DIRECTION ( 'NONE',  ( 0.000000000000000000, 1.000000000000000000, 0.000000000000000000 ) ) ;
#4633=CARTESIAN_POINT ( 'NONE',  ( -71.24615306438100504, 50.84170520456370923, -167.1454815528550739 ) ) ;
#4637=AXIS2_PLACEMENT_3D ( 'NONE', #17833, #3898, #3720 ) ;
#4640=LINE ( 'NONE', #13625, #9892 ) ;
#4642=ORIENTED_EDGE ( 'NONE', *, *, #6772, .F. ) ;
#4649=DIRECTION ( 'NONE',  ( 1.000000000000000000, 0.000000000000000000, 0.000000000000000000 ) ) ;
#4650=CARTESIAN_POINT ( 'NONE',  ( -68.99615306438067819, 145.9084177316626949, -15.00000000000001421 ) ) ;
#4653=DIRECTION ( 'NONE',  ( 0.000000000000000000, 0.000000000000000000, -1.000000000000000000 ) ) ;
#4655=DIRECTION ( 'NONE',  ( 0.000000000000000000, 0.000000000000000000, -1.000000000000000000 ) ) ;
#4657=DIRECTION ( 'NONE',  ( 0.000000000000000000, 1.000000000000000000, 0.000000000000000000 ) ) ;
#4658=ORIENTED_EDGE ( 'NONE', *, *, #10520, .T. ) ;
#4662=VERTEX_POINT ( 'NONE', #9539 ) ;
#4663=ORIENTED_EDGE ( 'NONE', *, *, #8830, .T. ) ;
#4664=ORIENTED_EDGE ( 'NONE', *, *, #250, .F. ) ;
#4665=CARTESIAN_POINT ( 'NONE',  ( -68.99615306438106188, 26.52789703166272162, 15.00000000000006928 ) ) ;
#4666=CARTESIAN_POINT ( 'NONE',  ( -68.99615306438089135, 83.07656473166271383, -15.00000000000001421 ) ) ;
#4667=EDGE_CURVE ( 'NONE', #2433, #16663, #2432, .T. ) ;
#4669=CARTESIAN_POINT ( 'NONE',  ( -71.24615306438079188, 104.2487802545637408, -15.00000000000001421 ) ) ;
#4673=PLANE ( 'NONE',  #5105 ) ;
#4674=CARTESIAN_POINT ( 'NONE',  ( -68.99615306438100504, 39.09426763166271002, 15.00000000000006928 ) ) ;
#4676=ORIENTED_EDGE ( 'NONE', *, *, #10256, .F. ) ;
#4680=LINE ( 'NONE', #2630, #14598 ) ;
#4682=EDGE_CURVE ( 'NONE', #677, #17987, #9639, .T. ) ;
#4683=PLANE ( 'NONE',  #11803 ) ;
#4685=LINE ( 'NONE', #14792, #12987 ) ;
#4688=EDGE_CURVE ( 'NONE', #16652, #15808, #5323, .T. ) ;
#4690=ORIENTED_EDGE ( 'NONE', *, *, #14068, .F. ) ;
#4692=DIRECTION ( 'NONE',  ( 0.000000000000000000, 0.000000000000000000, 1.000000000000000000 ) ) ;
#4697=VERTEX_POINT ( 'NONE', #13666 ) ;
#4701=ORIENTED_EDGE ( 'NONE', *, *, #15545, .T. ) ;
#4708=ADVANCED_FACE ( 'NONE', ( #11043 ), #16451, .T. ) ;
#4710=ORIENTED_EDGE ( 'NONE', *, *, #7236, .T. ) ;
#4712=CARTESIAN_POINT ( 'NONE',  ( -68.99615306438089135, 86.21815738166266385, 15.00000000000006928 ) ) ;
#4723=CARTESIAN_POINT ( 'NONE',  ( -71.24615306438111872, 21.67850061522927518, -15.00000000000001421 ) ) ;
#4727=DIRECTION ( 'NONE',  ( 1.000000000000000000, 0.000000000000000000, 0.000000000000000000 ) ) ;
#4729=DIRECTION ( 'NONE',  ( 1.000000000000000000, 0.000000000000000000, 0.000000000000000000 ) ) ;
#4730=DIRECTION ( 'NONE',  ( 1.000000000000000000, 0.000000000000000000, 0.000000000000000000 ) ) ;
#4731=CARTESIAN_POINT ( 'NONE',  ( -68.99615306438084872, 74.26664263813026423, 15.00000000000006928 ) ) ;
#4732=FACE_OUTER_BOUND ( 'NONE', #18389, .T. ) ;
#4739=EDGE_LOOP ( 'NONE', ( #17459, #9782, #11299, #2720 ) ) ;
#4740=VECTOR ( 'NONE', #17220, 1000.000000000000000 ) ;
#4743=VECTOR ( 'NONE', #252, 1000.000000000000000 ) ;
#4744=ORIENTED_EDGE ( 'NONE', *, *, #18315, .T. ) ;
#4746=CARTESIAN_POINT ( 'NONE',  ( -71.24615306438097662, 62.51920506522922949, -15.00000000000001421 ) ) ;
#4750=DIRECTION ( 'NONE',  ( 0.000000000000000000, 1.000000000000000000, 0.000000000000000000 ) ) ;
#4752=ORIENTED_EDGE ( 'NONE', *, *, #13167, .F. ) ;
#4757=CARTESIAN_POINT ( 'NONE',  ( -71.24615306438090556, 79.11603905456372843, -15.00000000000001421 ) ) ;
#4758=ORIENTED_EDGE ( 'NONE', *, *, #10967, .T. ) ;
#4763=ORIENTED_EDGE ( 'NONE', *, *, #376, .T. ) ;
#4768=CARTESIAN_POINT ( 'NONE',  ( -68.99615306438100504, 48.51904558166270220, 15.00000000000006928 ) ) ;
#4770=EDGE_CURVE ( 'NONE', #881, #8164, #13756, .T. ) ;
#4781=LINE ( 'NONE', #17698, #10736 ) ;
#4782=VERTEX_POINT ( 'NONE', #4214 ) ;
#4784=EDGE_CURVE ( 'NONE', #17387, #13044, #8616, .T. ) ;
#4785=LINE ( 'NONE', #6100, #5908 ) ;
#4788=EDGE_CURVE ( 'NONE', #2374, #11152, #2913, .T. ) ;
#4789=ADVANCED_FACE ( 'NONE', ( #2626 ), #14318, .T. ) ;
#4798=ADVANCED_FACE ( 'NONE', ( #16935 ), #8533, .T. ) ;
#4799=VECTOR ( 'NONE', #11184, 1000.000000000000000 ) ;
#4800=LINE ( 'NONE', #7981, #17071 ) ;
#4804=DIRECTION ( 'NONE',  ( 0.000000000000000000, 1.000000000000000000, 0.000000000000000000 ) ) ;
#4807=ORIENTED_EDGE ( 'NONE', *, *, #10752, .F. ) ;
#4815=ADVANCED_FACE ( 'NONE', ( #15443 ), #11424, .T. ) ;
#4818=CARTESIAN_POINT ( 'NONE',  ( -71.24615306438094819, 66.54966845456371516, -167.1454815528550739 ) ) ;
#4826=ORIENTED_EDGE ( 'NONE', *, *, #10987, .F. ) ;
#4830=LINE ( 'NONE', #9233, #8246 ) ;
#4834=ORIENTED_EDGE ( 'NONE', *, *, #3642, .F. ) ;
#4836=CARTESIAN_POINT ( 'NONE',  ( -68.99615306438074924, 120.7756765316626542, -15.00000000000001421 ) ) ;
#4838=EDGE_CURVE ( 'NONE', #4021, #8598, #15807, .T. ) ;
#4839=VECTOR ( 'NONE', #13676, 1000.000000000000114 ) ;
#4841=CARTESIAN_POINT ( 'NONE',  ( -71.24615306438074924, 116.8151508545637398, 15.00000000000006928 ) ) ;
#4843=ORIENTED_EDGE ( 'NONE', *, *, #9867, .T. ) ;
#4844=VECTOR ( 'NONE', #9370, 1000.000000000000000 ) ;
#4849=CARTESIAN_POINT ( 'NONE',  ( -71.24615306438070661, 134.7758360152292312, -167.1454815528550739 ) ) ;
#4856=CARTESIAN_POINT ( 'NONE',  ( -68.99615306438072082, 130.8153103381302742, -15.00000000000001421 ) ) ;
#4858=AXIS2_PLACEMENT_3D ( 'NONE', #10842, #13561, #751 ) ;
#4861=DIRECTION ( 'NONE',  ( 0.000000000000000000, 0.000000000000000000, -1.000000000000000000 ) ) ;
#4862=ORIENTED_EDGE ( 'NONE', *, *, #16573, .F. ) ;
#4863=EDGE_CURVE ( 'NONE', #4629, #12641, #10023, .T. ) ;
#4868=VERTEX_POINT ( 'NONE', #11330 ) ;
#4871=DIRECTION ( 'NONE',  ( 0.000000000000000000, 0.000000000000000000, 1.000000000000000000 ) ) ;
#4872=LINE ( 'NONE', #5151, #1572 ) ;
#4874=FACE_OUTER_BOUND ( 'NONE', #7173, .T. ) ;
#4876=DIRECTION ( 'NONE',  ( -1.000000000000000000, 0.000000000000000000, 1.156482317317869999E-16 ) ) ;
#4878=VERTEX_POINT ( 'NONE', #4396 ) ;
#4879=DIRECTION ( 'NONE',  ( 0.000000000000000000, 0.000000000000000000, 1.000000000000000000 ) ) ;
#4883=ORIENTED_EDGE ( 'NONE', *, *, #4682, .F. ) ;
#4885=ORIENTED_EDGE ( 'NONE', *, *, #3317, .F. ) ;
#4887=CARTESIAN_POINT ( 'NONE',  ( -68.99615306438089135, 80.54982793813027797, -167.1454815528550739 ) ) ;
#4888=VECTOR ( 'NONE', #771, 1000.000000000000000 ) ;
#4889=ORIENTED_EDGE ( 'NONE', *, *, #17853, .F. ) ;
#4891=EDGE_CURVE ( 'NONE', #11152, #11410, #7298, .T. ) ;
#4892=ORIENTED_EDGE ( 'NONE', *, *, #2972, .T. ) ;
#4893=CARTESIAN_POINT ( 'NONE',  ( -71.24615306438076345, 131.6342433652292243, -167.1454815528550739 ) ) ;
#4895=VECTOR ( 'NONE', #11384, 1000.000000000000000 ) ;
#4896=VERTEX_POINT ( 'NONE', #14405 ) ;
#4898=VECTOR ( 'NONE', #4442, 1000.000000000000000 ) ;
#4900=LINE ( 'NONE', #13696, #1251 ) ;
#4902=CARTESIAN_POINT ( 'NONE',  ( -68.99615306438089135, 67.98345733813025049, 15.00000000000006928 ) ) ;
#4903=ORIENTED_EDGE ( 'NONE', *, *, #18024, .F. ) ;
#4904=EDGE_CURVE ( 'NONE', #8741, #13368, #12755, .T. ) ;
#4906=ORIENTED_EDGE ( 'NONE', *, *, #6411, .T. ) ;
#4908=PLANE ( 'NONE',  #15609 ) ;
#4913=EDGE_CURVE ( 'NONE', #5159, #9970, #15984, .T. ) ;
#4918=ORIENTED_EDGE ( 'NONE', *, *, #8767, .T. ) ;
#4919=ORIENTED_EDGE ( 'NONE', *, *, #10289, .T. ) ;
#4920=DIRECTION ( 'NONE',  ( -0.9396926207859068736, 0.3420201433256725987, -4.890320548438441017E-16 ) ) ;
#4922=EDGE_CURVE ( 'NONE', #16527, #12968, #14499, .T. ) ;
#4923=ORIENTED_EDGE ( 'NONE', *, *, #3907, .T. ) ;
#4925=CARTESIAN_POINT ( 'NONE',  ( -71.24615306438070661, 134.7758360152292312, 15.00000000000006928 ) ) ;
#4927=CARTESIAN_POINT ( 'NONE',  ( -68.99615306438100504, 45.37745293166267402, -167.1454815528550739 ) ) ;
#4929=VECTOR ( 'NONE', #15149, 1000.000000000000000 ) ;
#4932=CARTESIAN_POINT ( 'NONE',  ( -70.27900850916093134, -47.21335801510345220, 15.00000000000008171 ) ) ;
#4935=AXIS2_PLACEMENT_3D ( 'NONE', #10718, #7549, #10542 ) ;
#4947=AXIS2_PLACEMENT_3D ( 'NONE', #13294, #473, #6150 ) ;
#4948=VECTOR ( 'NONE', #6712, 1000.000000000000000 ) ;
#4949=CARTESIAN_POINT ( 'NONE',  ( -68.99615306438104767, 14.57638228813024206, 15.00000000000006928 ) ) ;
#4952=CARTESIAN_POINT ( 'NONE',  ( -68.99615306438077766, 118.2489397381302751, -167.1454815528550739 ) ) ;
#4956=FACE_OUTER_BOUND ( 'NONE', #11769, .T. ) ;
#4957=ORIENTED_EDGE ( 'NONE', *, *, #18208, .F. ) ;
#4959=FACE_OUTER_BOUND ( 'NONE', #11051, .T. ) ;
#4960=EDGE_LOOP ( 'NONE', ( #17846, #1482, #13571, #760, #2469, #4270, #1733, #6395, #13078, #7571, #4084, #15416, #8259, #4247, #4919, #5276, #2826, #3481, #7473, #7987, #9116, #4892, #10325, #711, #1181, #869, #2183, #4138, #3853, #16104, #3531, #10402, #14983, #910, #7253, #10682, #8181, #13888, #724, #14254, #4295, #4107, #1226, #4334, #11139, #1312, #13698, #17677, #12230, #11315, #11106, #6448, #17021, #6294, #419, #13187, #5143, #18447, #13133, #18276, #3237, #15382, #5902, #4309, #3562, #15201, #1901, #3020, #8815, #10337, #13832, #1452, #7149, #11661, #1321, #5449, #2254, #14456, #14334, #3733, #9384, #4596, #282, #16026, #14950, #14336, #8829, #18133, #10516, #2578, #2897, #14825, #14633, #10014, #1384, #17929, #3794, #16129, #3304, #14672, #11824, #3933, #5419, #11486, #1964, #4918, #17349, #12116, #6464, #185, #7231, #12085, #4763, #9509, #7256, #8761, #4658, #501, #15081, #15866, #10328, #12087, #15406, #17545, #2459, #8538, #5615, #16944, #6536, #15591, #9147, #15010, #12556, #15608, #14325, #300, #13208, #2724, #3753, #14143, #18053, #790, #14733, #446, #12422, #12340, #1582, #4002, #12628, #8805, #14145, #5635, #5656, #14178, #7471, #12922, #3218, #17380, #17981, #18499, #6141, #16955, #13936, #10563, #12911, #5059, #6759, #15171, #978, #9310, #8575, #8300, #16437, #3683, #15043, #413, #167, #6864, #15114, #2007, #5967, #15585, #4326, #11291, #12061, #2829, #7661, #10133, #10674, #17738, #7840, #15463, #9814, #6604, #6964, #14868, #15040 ) ) ;
#4961=LINE ( 'NONE', #14870, #12834 ) ;
#4962=ORIENTED_EDGE ( 'NONE', *, *, #12503, .F. ) ;
#4963=ORIENTED_EDGE ( 'NONE', *, *, #17276, .F. ) ;
#4967=CARTESIAN_POINT ( 'NONE',  ( -71.24615306438117557, 5.970537365229261262, -167.1454815528550739 ) ) ;
#4968=ORIENTED_EDGE ( 'NONE', *, *, #17392, .F. ) ;
#4982=ORIENTED_EDGE ( 'NONE', *, *, #13373, .T. ) ;
#4984=CARTESIAN_POINT ( 'NONE',  ( -68.99615306438099083, 27.14275288813028553, 15.00000000000006928 ) ) ;
#4986=LINE ( 'NONE', #10797, #5094 ) ;
#4992=CARTESIAN_POINT ( 'NONE',  ( -71.24615306438069240, 126.2399288045637746, 15.00000000000006928 ) ) ;
#4994=VERTEX_POINT ( 'NONE', #11952 ) ;
#4999=VERTEX_POINT ( 'NONE', #9158 ) ;
#5004=DIRECTION ( 'NONE',  ( 1.000000000000000000, 0.000000000000000000, 0.000000000000000000 ) ) ;
#5005=( NAMED_UNIT ( * ) PLANE_ANGLE_UNIT ( ) SI_UNIT ( $, .RADIAN. ) );
#5007=CARTESIAN_POINT ( 'NONE',  ( -68.99615306438106188, 36.56753083813027416, -15.00000000000001421 ) ) ;
#5009=EDGE_CURVE ( 'NONE', #17707, #3371, #1678, .T. ) ;
#5012=DIRECTION ( 'NONE',  ( 1.000000000000000000, 0.000000000000000000, 0.000000000000000000 ) ) ;
#5015=ORIENTED_EDGE ( 'NONE', *, *, #11477, .T. ) ;
#5017=PLANE ( 'NONE',  #7790 ) ;
#5018=VERTEX_POINT ( 'NONE', #1759 ) ;
#5019=DIRECTION ( 'NONE',  ( 0.000000000000000000, 0.000000000000000000, 1.000000000000000000 ) ) ;
#5025=EDGE_CURVE ( 'NONE', #12950, #10713, #11863, .T. ) ;
#5026=ADVANCED_FACE ( 'NONE', ( #8796 ), #4563, .T. ) ;
#5027=AXIS2_PLACEMENT_3D ( 'NONE', #16455, #18157, #2332 ) ;
#5029=ORIENTED_EDGE ( 'NONE', *, *, #8501, .T. ) ;
#5032=DIRECTION ( 'NONE',  ( -0.9396926207859157554, 0.3420201433256481738, -4.890320548438487362E-16 ) ) ;
#5033=EDGE_CURVE ( 'NONE', #3439, #16762, #8884, .T. ) ;
#5037=CARTESIAN_POINT ( 'NONE',  ( -71.24615306438079188, 112.7846874652292399, -15.00000000000001421 ) ) ;
#5038=CARTESIAN_POINT ( 'NONE',  ( -71.24615306438086293, 87.65194626522927024, 15.00000000000006928 ) ) ;
#5041=CARTESIAN_POINT ( 'NONE',  ( -68.99615306438082030, 86.83301323813022066, 15.00000000000006928 ) ) ;
#5042=VECTOR ( 'NONE', #1915, 1000.000000000000114 ) ;
#5045=DIRECTION ( 'NONE',  ( 0.000000000000000000, 1.000000000000000000, 0.000000000000000000 ) ) ;
#5048=EDGE_CURVE ( 'NONE', #10428, #13041, #8112, .T. ) ;
#5049=ORIENTED_EDGE ( 'NONE', *, *, #6856, .F. ) ;
#5057=VECTOR ( 'NONE', #7051, 1000.000000000000000 ) ;
#5059=ORIENTED_EDGE ( 'NONE', *, *, #4838, .T. ) ;
#5060=CARTESIAN_POINT ( 'NONE',  ( -68.99615306438096241, 58.55867938813025120, -15.00000000000001421 ) ) ;
#5063=LINE ( 'NONE', #3766, #11447 ) ;
#5064=VERTEX_POINT ( 'NONE', #826 ) ;
#5067=CARTESIAN_POINT ( 'NONE',  ( -68.99615306438117557, 4.536748481662661092, 15.00000000000006928 ) ) ;
#5068=VERTEX_POINT ( 'NONE', #15031 ) ;
#5069=AXIS2_PLACEMENT_3D ( 'NONE', #287, #7490, #5981 ) ;
#5078=CARTESIAN_POINT ( 'NONE',  ( -68.99615306438072082, 139.6252324316626812, 15.00000000000006928 ) ) ;
#5085=CARTESIAN_POINT ( 'NONE',  ( -68.99615306438104767, 11.43478963813027249, 15.00000000000006928 ) ) ;
#5092=ORIENTED_EDGE ( 'NONE', *, *, #14103, .F. ) ;
#5093=VECTOR ( 'NONE', #13797, 1000.000000000000000 ) ;
#5094=VECTOR ( 'NONE', #7706, 1000.000000000000000 ) ;
#5096=CARTESIAN_POINT ( 'NONE',  ( -71.24615306438073503, 129.3815214545637104, -15.00000000000001421 ) ) ;
#5097=PLANE ( 'NONE',  #14166 ) ;
#5103=LINE ( 'NONE', #16417, #17146 ) ;
#5104=ORIENTED_EDGE ( 'NONE', *, *, #16684, .F. ) ;
#5105=AXIS2_PLACEMENT_3D ( 'NONE', #7674, #17493, #3465 ) ;
#5106=CARTESIAN_POINT ( 'NONE',  ( -68.99615306438083451, 99.39938383813029077, -15.00000000000001421 ) ) ;
#5108=DIRECTION ( 'NONE',  ( -0.9396926207859084279, 0.3420201433256686574, 1.086737899652989892E-16 ) ) ;
#5111=VECTOR ( 'NONE', #9467, 1000.000000000000000 ) ;
#5115=EDGE_LOOP ( 'NONE', ( #77, #740, #9702, #4076 ) ) ;
#5118=ORIENTED_EDGE ( 'NONE', *, *, #8798, .F. ) ;
#5121=EDGE_CURVE ( 'NONE', #13353, #10960, #6615, .T. ) ;
#5123=ORIENTED_EDGE ( 'NONE', *, *, #7525, .F. ) ;
#5124=VECTOR ( 'NONE', #6299, 1000.000000000000114 ) ;
#5125=AXIS2_PLACEMENT_3D ( 'NONE', #7052, #15543, #960 ) ;
#5127=PLANE ( 'NONE',  #393 ) ;
#5130=DIRECTION ( 'NONE',  ( 0.9396926207859158664, 0.3420201433256481738, 0.000000000000000000 ) ) ;
#5131=CARTESIAN_POINT ( 'NONE',  ( -71.24615306438097662, 57.12489050456376560, -167.1454815528550739 ) ) ;
#5134=ADVANCED_FACE ( 'NONE', ( #12531 ), #12339, .T. ) ;
#5136=CARTESIAN_POINT ( 'NONE',  ( -68.99615306438100504, 49.13390143813029454, 15.00000000000006928 ) ) ;
#5142=DIRECTION ( 'NONE',  ( 0.000000000000000000, 1.000000000000000000, 0.000000000000000000 ) ) ;
#5143=ORIENTED_EDGE ( 'NONE', *, *, #17480, .T. ) ;
#5144=EDGE_LOOP ( 'NONE', ( #2002, #14809, #16228, #3071 ) ) ;
#5145=ADVANCED_FACE ( 'NONE', ( #913 ), #5017, .T. ) ;
#5150=LINE ( 'NONE', #17682, #17554 ) ;
#5151=CARTESIAN_POINT ( 'NONE',  ( -71.24615306438073503, 128.4926507152292459, -167.1454815528550739 ) ) ;
#5152=DIRECTION ( 'NONE',  ( 0.9396926207859158664, 0.3420201433256481738, -1.086737899652998397E-16 ) ) ;
#5156=DIRECTION ( 'NONE',  ( 0.9396926207859171987, 0.3420201433256445100, 4.890320548438495251E-16 ) ) ;
#5158=CARTESIAN_POINT ( 'NONE',  ( -71.24615306438094819, 68.80239036522922902, -15.00000000000001421 ) ) ;
#5159=VERTEX_POINT ( 'NONE', #4104 ) ;
#5160=DIRECTION ( 'NONE',  ( 0.3420201433256612189, -0.9396926207859112035, 0.000000000000000000 ) ) ;
#5162=CARTESIAN_POINT ( 'NONE',  ( -68.99615306438100504, 42.85071613813029501, 15.00000000000006928 ) ) ;
#5163=VERTEX_POINT ( 'NONE', #16030 ) ;
#5168=VERTEX_POINT ( 'NONE', #8593 ) ;
#5170=CARTESIAN_POINT ( 'NONE',  ( -70.27900850916093134, -2.213358015103445098, -167.1454815528550739 ) ) ;
#5176=ORIENTED_EDGE ( 'NONE', *, *, #8626, .F. ) ;
#5178=LINE ( 'NONE', #1359, #6995 ) ;
#5179=CARTESIAN_POINT ( 'NONE',  ( -71.24615306438114715, 15.39531531522927921, 15.00000000000006928 ) ) ;
#5180=ORIENTED_EDGE ( 'NONE', *, *, #105, .F. ) ;
#5185=FACE_OUTER_BOUND ( 'NONE', #254, .T. ) ;
#5186=DIRECTION ( 'NONE',  ( -0.9396926207859022107, 0.3420201433256853663, 1.086737899652982620E-16 ) ) ;
#5189=AXIS2_PLACEMENT_3D ( 'NONE', #4154, #9861, #16870 ) ;
#5191=LINE ( 'NONE', #5085, #5124 ) ;
#5192=ORIENTED_EDGE ( 'NONE', *, *, #11778, .F. ) ;
#5194=CARTESIAN_POINT ( 'NONE',  ( -68.99615306438097662, 58.55867938813025830, -167.1454815528550739 ) ) ;
#5195=VERTEX_POINT ( 'NONE', #74 ) ;
#5197=VECTOR ( 'NONE', #17150, 1000.000000000000114 ) ;
#5198=ORIENTED_EDGE ( 'NONE', *, *, #6041, .F. ) ;
#5200=CARTESIAN_POINT ( 'NONE',  ( -71.24615306438111872, 22.56737135456379661, -167.1454815528550739 ) ) ;
#5203=LINE ( 'NONE', #15022, #1595 ) ;
#5206=VECTOR ( 'NONE', #17411, 1000.000000000000114 ) ;
#5207=EDGE_CURVE ( 'NONE', #10207, #16011, #11733, .T. ) ;
#5208=CARTESIAN_POINT ( 'NONE',  ( -71.24615306438111872, 19.42577870456376132, 15.00000000000006928 ) ) ;
#5209=CARTESIAN_POINT ( 'NONE',  ( -71.24615306438116136, 3.717815454563756727, -15.00000000000001421 ) ) ;
#5210=DIRECTION ( 'NONE',  ( 0.000000000000000000, 0.000000000000000000, -1.000000000000000000 ) ) ;
#5211=DIRECTION ( 'NONE',  ( 0.000000000000000000, 0.000000000000000000, 1.000000000000000000 ) ) ;
#5214=VECTOR ( 'NONE', #15008, 1000.000000000000000 ) ;
#5220=DIRECTION ( 'NONE',  ( -0.9396926207859103153, 0.3420201433256635504, 0.000000000000000000 ) ) ;
#5229=DIRECTION ( 'NONE',  ( 0.000000000000000000, 1.000000000000000000, 0.000000000000000000 ) ) ;
#5235=EDGE_LOOP ( 'NONE', ( #5301, #4701, #11050, #5833 ) ) ;
#5239=ORIENTED_EDGE ( 'NONE', *, *, #10507, .F. ) ;
#5240=LINE ( 'NONE', #13574, #12111 ) ;
#5247=EDGE_CURVE ( 'NONE', #9018, #10635, #1396, .T. ) ;
#5249=DIRECTION ( 'NONE',  ( 0.3420201433256444545, -0.9396926207859171987, 0.000000000000000000 ) ) ;
#5251=PLANE ( 'NONE',  #16543 ) ;
#5252=PLANE ( 'NONE',  #1886 ) ;
#5253=CARTESIAN_POINT ( 'NONE',  ( -68.99615306438072082, 133.9569029881302811, -167.1454815528550739 ) ) ;
#5256=ADVANCED_FACE ( 'NONE', ( #1807 ), #4005, .T. ) ;
#5258=DIRECTION ( 'NONE',  ( 0.000000000000000000, 1.000000000000000000, 0.000000000000000000 ) ) ;
#5259=DIRECTION ( 'NONE',  ( 0.000000000000000000, 0.000000000000000000, 1.000000000000000000 ) ) ;
#5261=EDGE_CURVE ( 'NONE', #9843, #13900, #4290, .T. ) ;
#5262=CARTESIAN_POINT ( 'NONE',  ( -68.99615306438080609, 105.0677132816627051, -15.00000000000001421 ) ) ;
#5265=ADVANCED_FACE ( 'NONE', ( #8925 ), #12807, .T. ) ;
#5268=EDGE_CURVE ( 'NONE', #5064, #16126, #9808, .T. ) ;
#5269=ADVANCED_FACE ( 'NONE', ( #2891 ), #15508, .T. ) ;
#5275=DIRECTION ( 'NONE',  ( 0.9396926207859102043, 0.3420201433256637724, -1.086737899652991864E-16 ) ) ;
#5276=ORIENTED_EDGE ( 'NONE', *, *, #5994, .T. ) ;
#5278=LINE ( 'NONE', #13794, #6095 ) ;
#5281=CARTESIAN_POINT ( 'NONE',  ( -71.24615306438103346, 46.81124181522922356, -15.00000000000001421 ) ) ;
#5282=PLANE ( 'NONE',  #12290 ) ;
#5283=EDGE_CURVE ( 'NONE', #8741, #4662, #4190, .T. ) ;
#5285=EDGE_LOOP ( 'NONE', ( #6716, #7854, #10820, #3707 ) ) ;
#5286=DIRECTION ( 'NONE',  ( 0.000000000000000000, 0.000000000000000000, -1.000000000000000000 ) ) ;
#5293=EDGE_CURVE ( 'NONE', #1839, #9751, #15612, .T. ) ;
#5295=FACE_OUTER_BOUND ( 'NONE', #5285, .T. ) ;
#5296=ORIENTED_EDGE ( 'NONE', *, *, #11667, .F. ) ;
#5298=CARTESIAN_POINT ( 'NONE',  ( -68.99615306438106188, 35.95267498166268894, -167.1454815528550739 ) ) ;
#5300=CARTESIAN_POINT ( 'NONE',  ( -71.24615306438120399, -0.3126479347707321610, -167.1454815528550739 ) ) ;
#5301=ORIENTED_EDGE ( 'NONE', *, *, #7319, .F. ) ;
#5304=CARTESIAN_POINT ( 'NONE',  ( -68.99615306438087714, 80.54982793813027797, -15.00000000000001421 ) ) ;
#5305=DIRECTION ( 'NONE',  ( 0.000000000000000000, 0.000000000000000000, 1.000000000000000000 ) ) ;
#5307=VERTEX_POINT ( 'NONE', #7887 ) ;
#5308=CARTESIAN_POINT ( 'NONE',  ( -71.24615306438080609, 103.3599095152292193, 15.00000000000006928 ) ) ;
#5311=ORIENTED_EDGE ( 'NONE', *, *, #12953, .F. ) ;
#5313=ORIENTED_EDGE ( 'NONE', *, *, #8487, .T. ) ;
#5317=LINE ( 'NONE', #14132, #13754 ) ;
#5320=DIRECTION ( 'NONE',  ( 0.000000000000000000, 0.000000000000000000, 1.000000000000000000 ) ) ;
#5323=LINE ( 'NONE', #15146, #1803 ) ;
#5324=ORIENTED_EDGE ( 'NONE', *, *, #5382, .F. ) ;
#5326=LINE ( 'NONE', #6452, #4929 ) ;
#5329=VECTOR ( 'NONE', #12929, 1000.000000000000000 ) ;
#5330=VERTEX_POINT ( 'NONE', #6472 ) ;
#5331=EDGE_LOOP ( 'NONE', ( #17776, #11304, #13543, #5655 ) ) ;
#5334=CARTESIAN_POINT ( 'NONE',  ( -71.24615306438114715, 13.14259340456377956, 15.00000000000006928 ) ) ;
#5335=DIRECTION ( 'NONE',  ( 0.3420201433256612189, -0.9396926207859112035, 0.000000000000000000 ) ) ;
#5336=CARTESIAN_POINT ( 'NONE',  ( -68.99615306438083451, 95.64293533166268446, 15.00000000000006928 ) ) ;
#5339=LINE ( 'NONE', #5060, #12910 ) ;
#5342=VERTEX_POINT ( 'NONE', #3574 ) ;
#5344=LINE ( 'NONE', #865, #590 ) ;
#5346=EDGE_CURVE ( 'NONE', #7186, #773, #6280, .T. ) ;
#5348=VERTEX_POINT ( 'NONE', #5067 ) ;
#5360=CARTESIAN_POINT ( 'NONE',  ( -68.99615306438089135, 79.93497208166267853, -15.00000000000001421 ) ) ;
#5362=ORIENTED_EDGE ( 'NONE', *, *, #10485, .T. ) ;
#5363=VECTOR ( 'NONE', #4497, 1000.000000000000000 ) ;
#5364=EDGE_CURVE ( 'NONE', #15862, #8464, #13602, .T. ) ;
#5369=VECTOR ( 'NONE', #11057, 1000.000000000000000 ) ;
#5371=LINE ( 'NONE', #18403, #15375 ) ;
#5374=ADVANCED_FACE ( 'NONE', ( #411 ), #2088, .T. ) ;
#5375=EDGE_CURVE ( 'NONE', #1161, #13022, #17883, .T. ) ;
#5376=EDGE_CURVE ( 'NONE', #8500, #9465, #4785, .T. ) ;
#5377=ORIENTED_EDGE ( 'NONE', *, *, #11559, .T. ) ;
#5382=EDGE_CURVE ( 'NONE', #17521, #15122, #10502, .T. ) ;
#5384=CARTESIAN_POINT ( 'NONE',  ( -71.24615306438113294, 0.5762228045638172480, 15.00000000000006928 ) ) ;
#5385=DIRECTION ( 'NONE',  ( 0.000000000000000000, 0.000000000000000000, 1.000000000000000000 ) ) ;
#5387=CARTESIAN_POINT ( 'NONE',  ( -68.99615306438117557, 4.536748481662661092, -15.00000000000001421 ) ) ;
#5388=DIRECTION ( 'NONE',  ( 1.000000000000000000, 0.000000000000000000, 0.000000000000000000 ) ) ;
#5391=CARTESIAN_POINT ( 'NONE',  ( -68.99615306438116136, 5.151604338130299610, -15.00000000000001421 ) ) ;
#5392=PLANE ( 'NONE',  #10932 ) ;
#5395=DIRECTION ( 'NONE',  ( 0.3420201433256686574, 0.9396926207859084279, -0.000000000000000000 ) ) ;
#5399=CARTESIAN_POINT ( 'NONE',  ( -68.99615306438106188, 29.66948968166269296, -167.1454815528550739 ) ) ;
#5402=EDGE_CURVE ( 'NONE', #5649, #14470, #16103, .T. ) ;
#5404=VECTOR ( 'NONE', #7648, 1000.000000000000114 ) ;
#5408=CARTESIAN_POINT ( 'NONE',  ( -68.99615306438080609, 105.6825691381303045, 15.00000000000006928 ) ) ;
#5414=DIRECTION ( 'NONE',  ( -0.9396926207859084279, 0.3420201433256687684, 1.086737899652989769E-16 ) ) ;
#5416=VECTOR ( 'NONE', #10598, 1000.000000000000114 ) ;
#5419=ORIENTED_EDGE ( 'NONE', *, *, #12634, .T. ) ;
#5422=VECTOR ( 'NONE', #13680, 1000.000000000000000 ) ;
#5423=CARTESIAN_POINT ( 'NONE',  ( -71.24615306438089135, 81.36876096522922808, 15.00000000000006928 ) ) ;
#5424=CARTESIAN_POINT ( 'NONE',  ( -68.99615306438077766, 111.9657544381302330, -15.00000000000001421 ) ) ;
#5432=DIRECTION ( 'NONE',  ( 1.000000000000000000, 0.000000000000000000, 0.000000000000000000 ) ) ;
#5433=EDGE_CURVE ( 'NONE', #8708, #16262, #688, .T. ) ;
#5435=VECTOR ( 'NONE', #4535, 1000.000000000000114 ) ;
#5436=LINE ( 'NONE', #5713, #2995 ) ;
#5446=CARTESIAN_POINT ( 'NONE',  ( -71.24615306438073503, 128.4926507152292459, 15.00000000000006928 ) ) ;
#5449=ORIENTED_EDGE ( 'NONE', *, *, #4595, .T. ) ;
#5450=VECTOR ( 'NONE', #14447, 1000.000000000000000 ) ;
#5451=VERTEX_POINT ( 'NONE', #16302 ) ;
#5457=ORIENTED_EDGE ( 'NONE', *, *, #12856, .F. ) ;
#5459=ORIENTED_EDGE ( 'NONE', *, *, #15324, .T. ) ;
#5468=CARTESIAN_POINT ( 'NONE',  ( -68.99615306438109030, 17.10311908166270456, -15.00000000000001421 ) ) ;
#5470=VERTEX_POINT ( 'NONE', #3489 ) ;
#5471=EDGE_CURVE ( 'NONE', #13044, #4868, #7796, .T. ) ;
#5473=CARTESIAN_POINT ( 'NONE',  ( -68.99615306438100504, 45.99230878813026635, -167.1454815528550739 ) ) ;
#5474=VECTOR ( 'NONE', #2136, 1000.000000000000000 ) ;
#5475=DIRECTION ( 'NONE',  ( -0.9396926207859157554, 0.3420201433256481738, -4.890320548438487362E-16 ) ) ;
#5476=ORIENTED_EDGE ( 'NONE', *, *, #8130, .T. ) ;
#5483=PRODUCT_DEFINITION_FORMATION_WITH_SPECIFIED_SOURCE ( 'ANY', '', #2051, .NOT_KNOWN. ) ;
#5486=CARTESIAN_POINT ( 'NONE',  ( -71.24615306438090556, 75.97444640456376419, -15.00000000000001421 ) ) ;
#5488=CARTESIAN_POINT ( 'NONE',  ( -68.99615306438089135, 83.07656473166271383, -167.1454815528550739 ) ) ;
#5489=ORIENTED_EDGE ( 'NONE', *, *, #15356, .T. ) ;
#5490=CARTESIAN_POINT ( 'NONE',  ( -68.99615306438093398, 39.70912348813025261, 15.00000000000006928 ) ) ;
#5491=LINE ( 'NONE', #16805, #2574 ) ;
#5493=DIRECTION ( 'NONE',  ( -0.9396926207859103153, 0.3420201433256635504, 0.000000000000000000 ) ) ;
#5504=LINE ( 'NONE', #4106, #11386 ) ;
#5506=VECTOR ( 'NONE', #5825, 1000.000000000000000 ) ;
#5507=ORIENTED_EDGE ( 'NONE', *, *, #3302, .T. ) ;
#5511=EDGE_CURVE ( 'NONE', #14653, #2315, #6565, .T. ) ;
#5516=ORIENTED_EDGE ( 'NONE', *, *, #9247, .F. ) ;
#5523=LINE ( 'NONE', #18151, #2151 ) ;
#5525=VERTEX_POINT ( 'NONE', #2354 ) ;
#5526=EDGE_CURVE ( 'NONE', #6870, #13041, #8270, .T. ) ;
#5527=CARTESIAN_POINT ( 'NONE',  ( -71.24615306438070661, 137.9174286652292096, -167.1454815528550739 ) ) ;
#5528=ORIENTED_EDGE ( 'NONE', *, *, #13180, .F. ) ;
#5531=LINE ( 'NONE', #10192, #12526 ) ;
#5532=EDGE_LOOP ( 'NONE', ( #4807, #17906, #17522, #13251 ) ) ;
#5536=CARTESIAN_POINT ( 'NONE',  ( -68.99615306438077766, 124.5321250381302747, -15.00000000000001421 ) ) ;
#5537=FACE_OUTER_BOUND ( 'NONE', #16204, .T. ) ;
#5538=CARTESIAN_POINT ( 'NONE',  ( -71.24615306438117557, 5.970537365229261262, 15.00000000000006928 ) ) ;
#5543=DIRECTION ( 'NONE',  ( -0.9396926207859171987, 0.3420201433256444545, 1.086737899652999999E-16 ) ) ;
#5545=CARTESIAN_POINT ( 'NONE',  ( -68.99615306438117557, 1.395155831662692192, 15.00000000000006928 ) ) ;
#5548=CARTESIAN_POINT ( 'NONE',  ( -71.24615306438110451, 19.42577870456376843, -15.00000000000001421 ) ) ;
#5552=ORIENTED_EDGE ( 'NONE', *, *, #11559, .F. ) ;
#5560=VERTEX_POINT ( 'NONE', #12395 ) ;
#5563=FACE_OUTER_BOUND ( 'NONE', #10523, .T. ) ;
#5566=CARTESIAN_POINT ( 'NONE',  ( -68.99615306438080609, 108.2093059316626693, -167.1454815528550739 ) ) ;
#5568=DIRECTION ( 'NONE',  ( 0.9396926207859078728, 0.3420201433256701007, 0.000000000000000000 ) ) ;
#5569=ORIENTED_EDGE ( 'NONE', *, *, #13838, .F. ) ;
#5570=ADVANCED_FACE ( 'NONE', ( #14064 ), #12292, .T. ) ;
#5572=VERTEX_POINT ( 'NONE', #13979 ) ;
#5574=CARTESIAN_POINT ( 'NONE',  ( -68.99615306438111872, 14.57638228813026871, -167.1454815528550739 ) ) ;
#5576=EDGE_CURVE ( 'NONE', #10635, #16643, #6671, .T. ) ;
#5580=CARTESIAN_POINT ( 'NONE',  ( -68.99615306438067819, 146.5232735881302801, 15.00000000000006928 ) ) ;
#5581=EDGE_LOOP ( 'NONE', ( #7254, #18182, #14154, #16294 ) ) ;
#5583=DIRECTION ( 'NONE',  ( 0.000000000000000000, 0.000000000000000000, 1.000000000000000000 ) ) ;
#5596=ORIENTED_EDGE ( 'NONE', *, *, #1958, .T. ) ;
#5600=DIRECTION ( 'NONE',  ( 0.000000000000000000, 1.000000000000000000, 0.000000000000000000 ) ) ;
#5601=ORIENTED_EDGE ( 'NONE', *, *, #11577, .F. ) ;
#5611=ORIENTED_EDGE ( 'NONE', *, *, #12373, .T. ) ;
#5613=FACE_OUTER_BOUND ( 'NONE', #4739, .T. ) ;
#5614=CARTESIAN_POINT ( 'NONE',  ( -71.24615306438117557, 5.970537365229261262, 15.00000000000006928 ) ) ;
#5615=ORIENTED_EDGE ( 'NONE', *, *, #11685, .T. ) ;
#5617=EDGE_CURVE ( 'NONE', #9665, #6928, #10314, .T. ) ;
#5623=DIRECTION ( 'NONE',  ( 0.9396926207859084279, 0.3420201433256686574, 0.000000000000000000 ) ) ;
#5625=CARTESIAN_POINT ( 'NONE',  ( -71.24615306438076345, 126.2399288045637462, -15.00000000000001421 ) ) ;
#5628=DIRECTION ( 'NONE',  ( 0.000000000000000000, 0.000000000000000000, -1.000000000000000000 ) ) ;
#5629=ORIENTED_EDGE ( 'NONE', *, *, #12634, .F. ) ;
#5631=ORIENTED_EDGE ( 'NONE', *, *, #9951, .F. ) ;
#5632=CARTESIAN_POINT ( 'NONE',  ( -71.24615306438086293, 94.82400230456377699, -167.1454815528550739 ) ) ;
#5635=ORIENTED_EDGE ( 'NONE', *, *, #9586, .T. ) ;
#5638=ORIENTED_EDGE ( 'NONE', *, *, #12667, .T. ) ;
#5640=ORIENTED_EDGE ( 'NONE', *, *, #14773, .T. ) ;
#5644=LINE ( 'NONE', #8276, #6956 ) ;
#5648=CARTESIAN_POINT ( 'NONE',  ( -68.99615306438111872, 20.24471173166267590, -15.00000000000001421 ) ) ;
#5649=VERTEX_POINT ( 'NONE', #17230 ) ;
#5650=CARTESIAN_POINT ( 'NONE',  ( -68.99615306438077766, 117.6340838816626899, -167.1454815528550739 ) ) ;
#5652=LINE ( 'NONE', #4163, #17989 ) ;
#5655=ORIENTED_EDGE ( 'NONE', *, *, #13286, .F. ) ;
#5656=ORIENTED_EDGE ( 'NONE', *, *, #5402, .T. ) ;
#5661=ORIENTED_EDGE ( 'NONE', *, *, #3673, .T. ) ;
#5662=CARTESIAN_POINT ( 'NONE',  ( -68.99615306438070661, 137.0984956381303164, 15.00000000000006928 ) ) ;
#5664=CARTESIAN_POINT ( 'NONE',  ( -68.99615306438091977, 73.65178678166269322, -167.1454815528550739 ) ) ;
#5668=CARTESIAN_POINT ( 'NONE',  ( -71.24615306438097662, 56.23601976522923707, -167.1454815528550739 ) ) ;
#5671=DIRECTION ( 'NONE',  ( 0.000000000000000000, 1.000000000000000000, 0.000000000000000000 ) ) ;
#5672=CARTESIAN_POINT ( 'NONE',  ( -68.99615306438082030, 102.5409764881302692, -15.00000000000001421 ) ) ;
#5673=DIRECTION ( 'NONE',  ( -0.9396926207859168656, 0.3420201433256456203, 0.000000000000000000 ) ) ;
#5676=DIRECTION ( 'NONE',  ( 0.3420201433256724322, 0.9396926207859070956, -0.000000000000000000 ) ) ;
#5678=CARTESIAN_POINT ( 'NONE',  ( -68.99615306438111872, 11.43478963813029914, -167.1454815528550739 ) ) ;
#5679=CARTESIAN_POINT ( 'NONE',  ( -68.99615306438083451, 98.78452798166264870, 15.00000000000006928 ) ) ;
#5681=AXIS2_PLACEMENT_3D ( 'NONE', #2843, #7138, #12949 ) ;
#5684=DIRECTION ( 'NONE',  ( 0.9396926207859171987, 0.3420201433256444545, 0.000000000000000000 ) ) ;
#5687=DIRECTION ( 'NONE',  ( 1.000000000000000000, 0.000000000000000000, 0.000000000000000000 ) ) ;
#5692=DIRECTION ( 'NONE',  ( 0.000000000000000000, 0.000000000000000000, 1.000000000000000000 ) ) ;
#5693=DIRECTION ( 'NONE',  ( 0.000000000000000000, 0.000000000000000000, 1.000000000000000000 ) ) ;
#5696=VECTOR ( 'NONE', #7827, 1000.000000000000000 ) ;
#5699=EDGE_CURVE ( 'NONE', #13839, #9806, #12084, .T. ) ;
#5701=LINE ( 'NONE', #4311, #6203 ) ;
#5702=ORIENTED_EDGE ( 'NONE', *, *, #7739, .T. ) ;
#5703=VERTEX_POINT ( 'NONE', #2152 ) ;
#5706=VECTOR ( 'NONE', #9213, 1000.000000000000000 ) ;
#5709=LINE ( 'NONE', #9650, #385 ) ;
#5711=DIRECTION ( 'NONE',  ( -0.9396926207859097602, 0.3420201433256649937, 0.000000000000000000 ) ) ;
#5713=CARTESIAN_POINT ( 'NONE',  ( -68.99615306438106188, 27.14275288813031040, -167.1454815528550739 ) ) ;
#5717=VERTEX_POINT ( 'NONE', #11978 ) ;
#5718=AXIS2_PLACEMENT_3D ( 'NONE', #17974, #5160, #16569 ) ;
#5729=ORIENTED_EDGE ( 'NONE', *, *, #13159, .F. ) ;
#5731=VECTOR ( 'NONE', #16499, 1000.000000000000114 ) ;
#5732=CARTESIAN_POINT ( 'NONE',  ( -71.24615306438103346, 43.66964916522919538, 15.00000000000006928 ) ) ;
#5733=CARTESIAN_POINT ( 'NONE',  ( -71.24615306438084872, 88.54081700456373483, -15.00000000000001421 ) ) ;
#5734=CARTESIAN_POINT ( 'NONE',  ( -71.24615306438076345, 131.6342433652292243, -15.00000000000001421 ) ) ;
#5735=VERTEX_POINT ( 'NONE', #17676 ) ;
#5736=AXIS2_PLACEMENT_3D ( 'NONE', #11121, #16808, #4001 ) ;
#5737=ORIENTED_EDGE ( 'NONE', *, *, #3319, .F. ) ;
#5739=EDGE_CURVE ( 'NONE', #12968, #12199, #4961, .T. ) ;
#5741=CARTESIAN_POINT ( 'NONE',  ( -68.99615306438089135, 83.69142058813029905, -15.00000000000001421 ) ) ;
#5742=VERTEX_POINT ( 'NONE', #16363 ) ;
#5744=CARTESIAN_POINT ( 'NONE',  ( -71.24615306438070661, 141.0590213152292449, -15.00000000000001421 ) ) ;
#5751=ORIENTED_EDGE ( 'NONE', *, *, #6626, .F. ) ;
#5754=VERTEX_POINT ( 'NONE', #6163 ) ;
#5758=ORIENTED_EDGE ( 'NONE', *, *, #6284, .T. ) ;
#5759=LINE ( 'NONE', #163, #4184 ) ;
#5760=DIRECTION ( 'NONE',  ( 0.000000000000000000, 1.000000000000000000, 0.000000000000000000 ) ) ;
#5761=DIRECTION ( 'NONE',  ( 0.000000000000000000, 1.000000000000000000, 0.000000000000000000 ) ) ;
#5764=DIRECTION ( 'NONE',  ( 0.000000000000000000, 0.000000000000000000, -1.000000000000000000 ) ) ;
#5765=VECTOR ( 'NONE', #11608, 1000.000000000000000 ) ;
#5767=VECTOR ( 'NONE', #5259, 1000.000000000000000 ) ;
#5768=PLANE ( 'NONE',  #15617 ) ;
#5772=VECTOR ( 'NONE', #6996, 1000.000000000000114 ) ;
#5774=DIRECTION ( 'NONE',  ( 0.000000000000000000, 1.000000000000000000, 0.000000000000000000 ) ) ;
#5775=ORIENTED_EDGE ( 'NONE', *, *, #7680, .F. ) ;
#5778=CARTESIAN_POINT ( 'NONE',  ( -68.99615306438111872, 20.24471173166267235, -167.1454815528550739 ) ) ;
#5781=CARTESIAN_POINT ( 'NONE',  ( 0.000000000000000000, 0.000000000000000000, 0.000000000000000000 ) ) ;
#5784=VERTEX_POINT ( 'NONE', #7494 ) ;
#5787=LINE ( 'NONE', #13015, #17675 ) ;
#5788=ORIENTED_EDGE ( 'NONE', *, *, #10166, .F. ) ;
#5791=VECTOR ( 'NONE', #3863, 999.9999999999998863 ) ;
#5792=DIRECTION ( 'NONE',  ( 0.9396926207859097602, 0.3420201433256649937, 0.000000000000000000 ) ) ;
#5795=DIRECTION ( 'NONE',  ( 0.000000000000000000, 1.000000000000000000, 0.000000000000000000 ) ) ;
#5796=ORIENTED_EDGE ( 'NONE', *, *, #8767, .F. ) ;
#5798=VECTOR ( 'NONE', #13109, 1000.000000000000000 ) ;
#5802=VECTOR ( 'NONE', #8833, 1000.000000000000000 ) ;
#5806=EDGE_CURVE ( 'NONE', #12040, #12836, #13479, .T. ) ;
#5809=ORIENTED_EDGE ( 'NONE', *, *, #13067, .T. ) ;
#5821=EDGE_CURVE ( 'NONE', #16605, #8708, #13307, .T. ) ;
#5822=EDGE_CURVE ( 'NONE', #5735, #4782, #10393, .T. ) ;
#5824=CARTESIAN_POINT ( 'NONE',  ( -68.99615306438066398, 146.5232735881302801, -15.00000000000001421 ) ) ;
#5825=DIRECTION ( 'NONE',  ( 0.000000000000000000, 1.000000000000000000, 0.000000000000000000 ) ) ;
#5827=AXIS2_PLACEMENT_3D ( 'NONE', #11713, #11886, #14600 ) ;
#5829=ORIENTED_EDGE ( 'NONE', *, *, #9043, .T. ) ;
#5833=ORIENTED_EDGE ( 'NONE', *, *, #1074, .F. ) ;
#5834=LINE ( 'NONE', #14450, #4220 ) ;
#5835=EDGE_CURVE ( 'NONE', #1745, #5859, #4680, .T. ) ;
#5839=CARTESIAN_POINT ( 'NONE',  ( -68.99615306438090556, 77.40823528813029952, -15.00000000000001421 ) ) ;
#5841=EDGE_CURVE ( 'NONE', #15702, #3179, #2542, .T. ) ;
#5842=ORIENTED_EDGE ( 'NONE', *, *, #9586, .F. ) ;
#5847=EDGE_CURVE ( 'NONE', #7166, #6487, #2436, .T. ) ;
#5850=DIRECTION ( 'NONE',  ( -0.9396926207859157554, 0.3420201433256481738, -4.890320548438487362E-16 ) ) ;
#5851=CARTESIAN_POINT ( 'NONE',  ( -71.24615306438083451, 97.07672421522921979, -15.00000000000001421 ) ) ;
#5858=LINE ( 'NONE', #3308, #4898 ) ;
#5859=VERTEX_POINT ( 'NONE', #5424 ) ;
#5860=FACE_OUTER_BOUND ( 'NONE', #10082, .T. ) ;
#5862=EDGE_LOOP ( 'NONE', ( #5924, #1837, #1129, #12780 ) ) ;
#5863=CARTESIAN_POINT ( 'NONE',  ( -71.24615306438100504, 53.09442711522921599, -15.00000000000001421 ) ) ;
#5867=ORIENTED_EDGE ( 'NONE', *, *, #12738, .T. ) ;
#5868=DIRECTION ( 'NONE',  ( 0.000000000000000000, 0.000000000000000000, 1.000000000000000000 ) ) ;
#5872=FACE_OUTER_BOUND ( 'NONE', #5115, .T. ) ;
#5873=ORIENTED_EDGE ( 'NONE', *, *, #16015, .F. ) ;
#5879=CARTESIAN_POINT ( 'NONE',  ( -68.99615306438111872, 13.96152643166267993, -15.00000000000001421 ) ) ;
#5880=DIRECTION ( 'NONE',  ( -0.9396926207858996571, 0.3420201433256928603, -4.890320548438403546E-16 ) ) ;
#5888=DIRECTION ( 'NONE',  ( 0.000000000000000000, 1.000000000000000000, 0.000000000000000000 ) ) ;
#5890=LINE ( 'NONE', #7313, #4196 ) ;
#5891=LINE ( 'NONE', #7396, #3322 ) ;
#5893=ADVANCED_FACE ( 'NONE', ( #2252 ), #16642, .T. ) ;
#5895=DIRECTION ( 'NONE',  ( 0.000000000000000000, 0.000000000000000000, 1.000000000000000000 ) ) ;
#5896=CARTESIAN_POINT ( 'NONE',  ( -68.99615306438086293, 89.35975003166268493, -15.00000000000001421 ) ) ;
#5902=ORIENTED_EDGE ( 'NONE', *, *, #8710, .T. ) ;
#5905=DIRECTION ( 'NONE',  ( 0.000000000000000000, 1.000000000000000000, 0.000000000000000000 ) ) ;
#5907=ORIENTED_EDGE ( 'NONE', *, *, #11454, .T. ) ;
#5908=VECTOR ( 'NONE', #16484, 1000.000000000000000 ) ;
#5909=CARTESIAN_POINT ( 'NONE',  ( -68.99615306438072082, 130.2004544816626890, -15.00000000000001421 ) ) ;
#5910=LINE ( 'NONE', #15935, #933 ) ;
#5913=LINE ( 'NONE', #11557, #16188 ) ;
#5915=LINE ( 'NONE', #5839, #11637 ) ;
#5917=VERTEX_POINT ( 'NONE', #1048 ) ;
#5919=VECTOR ( 'NONE', #7861, 1000.000000000000000 ) ;
#5924=ORIENTED_EDGE ( 'NONE', *, *, #6411, .F. ) ;
#5926=DIRECTION ( 'NONE',  ( 0.000000000000000000, 1.000000000000000000, 0.000000000000000000 ) ) ;
#5930=LINE ( 'NONE', #14554, #2846 ) ;
#5932=ADVANCED_FACE ( 'NONE', ( #18250 ), #12659, .T. ) ;
#5933=DIRECTION ( 'NONE',  ( 0.000000000000000000, 0.000000000000000000, -1.000000000000000000 ) ) ;
#5934=VECTOR ( 'NONE', #15699, 1000.000000000000114 ) ;
#5942=EDGE_CURVE ( 'NONE', #14470, #8569, #4217, .T. ) ;
#5946=VECTOR ( 'NONE', #4165, 1000.000000000000000 ) ;
#5948=EDGE_CURVE ( 'NONE', #8797, #8085, #5701, .T. ) ;
#5949=AXIS2_PLACEMENT_3D ( 'NONE', #15950, #13145, #17340 ) ;
#5955=PLANE ( 'NONE',  #4047 ) ;
#5959=EDGE_CURVE ( 'NONE', #11545, #15187, #7040, .T. ) ;
#5961=DIRECTION ( 'NONE',  ( 0.000000000000000000, 0.000000000000000000, -1.000000000000000000 ) ) ;
#5966=ORIENTED_EDGE ( 'NONE', *, *, #2166, .F. ) ;
#5967=ORIENTED_EDGE ( 'NONE', *, *, #15782, .T. ) ;
#5969=DIRECTION ( 'NONE',  ( 0.9396926207859097602, 0.3420201433256649937, -1.086737899652991371E-16 ) ) ;
#5970=DIRECTION ( 'NONE',  ( 0.000000000000000000, 0.000000000000000000, 1.000000000000000000 ) ) ;
#5975=VECTOR ( 'NONE', #16700, 1000.000000000000000 ) ;
#5976=DIRECTION ( 'NONE',  ( 0.000000000000000000, 1.000000000000000000, 0.000000000000000000 ) ) ;
#5979=DIRECTION ( 'NONE',  ( 0.000000000000000000, 0.000000000000000000, -1.000000000000000000 ) ) ;
#5981=DIRECTION ( 'NONE',  ( 0.000000000000000000, 0.000000000000000000, -1.000000000000000000 ) ) ;
#5983=LINE ( 'NONE', #7591, #10029 ) ;
#5988=EDGE_CURVE ( 'NONE', #13329, #4697, #10026, .T. ) ;
#5989=ORIENTED_EDGE ( 'NONE', *, *, #1958, .F. ) ;
#5992=CARTESIAN_POINT ( 'NONE',  ( -68.99615306438072082, 133.3420471316626958, -15.00000000000001421 ) ) ;
#5994=EDGE_CURVE ( 'NONE', #3227, #9065, #7122, .T. ) ;
#5996=ORIENTED_EDGE ( 'NONE', *, *, #6268, .T. ) ;
#6004=FACE_OUTER_BOUND ( 'NONE', #4341, .T. ) ;
#6007=ORIENTED_EDGE ( 'NONE', *, *, #4891, .F. ) ;
#6010=AXIS2_PLACEMENT_3D ( 'NONE', #14293, #6807, #12528 ) ;
#6016=DIRECTION ( 'NONE',  ( 0.000000000000000000, 1.000000000000000000, 0.000000000000000000 ) ) ;
#6017=LINE ( 'NONE', #16120, #14195 ) ;
#6019=VECTOR ( 'NONE', #5305, 1000.000000000000000 ) ;
#6026=AXIS2_PLACEMENT_3D ( 'NONE', #1854, #18109, #3249 ) ;
#6030=EDGE_CURVE ( 'NONE', #15808, #2407, #5531, .T. ) ;
#6033=ORIENTED_EDGE ( 'NONE', *, *, #7916, .F. ) ;
#6037=DIRECTION ( 'NONE',  ( 0.000000000000000000, 0.000000000000000000, 1.000000000000000000 ) ) ;
#6039=FACE_OUTER_BOUND ( 'NONE', #11449, .T. ) ;
#6040=EDGE_LOOP ( 'NONE', ( #12638, #17797, #2761, #15551 ) ) ;
#6041=EDGE_CURVE ( 'NONE', #12790, #9020, #12757, .T. ) ;
#6042=EDGE_CURVE ( 'NONE', #5163, #10938, #18450, .T. ) ;
#6043=CARTESIAN_POINT ( 'NONE',  ( -71.24615306438086293, 93.93513156522925556, -15.00000000000001421 ) ) ;
#6050=ORIENTED_EDGE ( 'NONE', *, *, #14387, .F. ) ;
#6051=EDGE_CURVE ( 'NONE', #6455, #14401, #17123, .T. ) ;
#6053=CARTESIAN_POINT ( 'NONE',  ( -68.99615306438072082, 140.2400882881302948, 15.00000000000006928 ) ) ;
#6061=EDGE_CURVE ( 'NONE', #6521, #13576, #2916, .T. ) ;
#6067=LINE ( 'NONE', #4669, #11499 ) ;
#6068=EDGE_CURVE ( 'NONE', #7201, #8164, #8619, .T. ) ;
#6070=AXIS2_PLACEMENT_3D ( 'NONE', #6497, #12216, #10814 ) ;
#6072=FACE_OUTER_BOUND ( 'NONE', #16035, .T. ) ;
#6078=LINE ( 'NONE', #17403, #1941 ) ;
#6081=VECTOR ( 'NONE', #8688, 1000.000000000000000 ) ;
#6089=VERTEX_POINT ( 'NONE', #2996 ) ;
#6093=LINE ( 'NONE', #8845, #16252 ) ;
#6095=VECTOR ( 'NONE', #3783, 1000.000000000000114 ) ;
#6098=CARTESIAN_POINT ( 'NONE',  ( -68.99615306438117557, 1.395155831662692192, -167.1454815528550739 ) ) ;
#6100=CARTESIAN_POINT ( 'NONE',  ( -68.99615306438106188, 24.00116023813026445, -167.1454815528550739 ) ) ;
#6101=ORIENTED_EDGE ( 'NONE', *, *, #4788, .T. ) ;
#6102=ORIENTED_EDGE ( 'NONE', *, *, #18204, .F. ) ;
#6103=AXIS2_PLACEMENT_3D ( 'NONE', #2507, #9613, #15315 ) ;
#6105=VECTOR ( 'NONE', #8423, 1000.000000000000000 ) ;
#6106=DIRECTION ( 'NONE',  ( 0.000000000000000000, 1.000000000000000000, 0.000000000000000000 ) ) ;
#6108=CARTESIAN_POINT ( 'NONE',  ( -71.24615306438067819, 145.0894847045637732, -167.1454815528550739 ) ) ;
#6110=DIRECTION ( 'NONE',  ( 0.000000000000000000, 0.000000000000000000, -1.000000000000000000 ) ) ;
#6111=DIRECTION ( 'NONE',  ( 1.000000000000000000, 0.000000000000000000, 0.000000000000000000 ) ) ;
#6113=ORIENTED_EDGE ( 'NONE', *, *, #4582, .F. ) ;
#6114=FACE_OUTER_BOUND ( 'NONE', #5581, .T. ) ;
#6122=EDGE_LOOP ( 'NONE', ( #16734, #1983, #2667, #5516 ) ) ;
#6125=CARTESIAN_POINT ( 'NONE',  ( -71.24615306438120399, -0.3126479347707322720, -15.00000000000001421 ) ) ;
#6127=CARTESIAN_POINT ( 'NONE',  ( -68.99615306438106188, 27.14275288813031040, 15.00000000000006928 ) ) ;
#6131=PLANE ( 'NONE',  #294 ) ;
#6139=LINE ( 'NONE', #16259, #17934 ) ;
#6141=ORIENTED_EDGE ( 'NONE', *, *, #8798, .T. ) ;
#6144=MANIFOLD_SOLID_BREP ( 'Boss-Extrude16', #132 ) ;
#6146=ORIENTED_EDGE ( 'NONE', *, *, #14984, .F. ) ;
#6149=DIRECTION ( 'NONE',  ( -0.9396926207859084279, 0.3420201433256686574, -4.890320548438448905E-16 ) ) ;
#6150=DIRECTION ( 'NONE',  ( 0.9396926207859084279, 0.3420201433256686574, 0.000000000000000000 ) ) ;
#6151=DIRECTION ( 'NONE',  ( -0.9999883591161159435, 0.004825104377941397994, 0.000000000000000000 ) ) ;
#6153=DIRECTION ( 'NONE',  ( 0.000000000000000000, 0.000000000000000000, 1.000000000000000000 ) ) ;
#6154=LINE ( 'NONE', #6447, #11714 ) ;
#6159=CARTESIAN_POINT ( 'NONE',  ( -68.99615306438086293, 92.50134268166266338, 15.00000000000006928 ) ) ;
#6160=DIRECTION ( 'NONE',  ( 1.000000000000000000, 0.000000000000000000, 0.000000000000000000 ) ) ;
#6161=ORIENTED_EDGE ( 'NONE', *, *, #9126, .F. ) ;
#6162=CARTESIAN_POINT ( 'NONE',  ( -68.99615306438072082, 130.8153103381302742, 15.00000000000006928 ) ) ;
#6163=CARTESIAN_POINT ( 'NONE',  ( -68.99615306438074924, 121.3905323881302962, 15.00000000000006928 ) ) ;
#6164=ORIENTED_EDGE ( 'NONE', *, *, #11353, .F. ) ;
#6166=EDGE_CURVE ( 'NONE', #15968, #9281, #17654, .T. ) ;
#6170=CARTESIAN_POINT ( 'NONE',  ( -68.99615306438111872, 10.81993378166265529, -15.00000000000001421 ) ) ;
#6173=ORIENTED_EDGE ( 'NONE', *, *, #1176, .F. ) ;
#6174=LINE ( 'NONE', #6463, #13482 ) ;
#6175=EDGE_LOOP ( 'NONE', ( #9524, #4043, #495, #463 ) ) ;
#6179=LINE ( 'NONE', #224, #16804 ) ;
#6183=CARTESIAN_POINT ( 'NONE',  ( -71.24615306438070661, 141.0590213152292449, -167.1454815528550739 ) ) ;
#6184=VERTEX_POINT ( 'NONE', #15987 ) ;
#6185=DIRECTION ( 'NONE',  ( -0.9396926207859097602, 0.3420201433256649937, 1.086737899652991371E-16 ) ) ;
#6187=ORIENTED_EDGE ( 'NONE', *, *, #8118, .T. ) ;
#6190=DIRECTION ( 'NONE',  ( 0.000000000000000000, 1.000000000000000000, 0.000000000000000000 ) ) ;
#6193=VERTEX_POINT ( 'NONE', #9242 ) ;
#6194=CARTESIAN_POINT ( 'NONE',  ( -71.24615306438103346, 46.81124181522922356, -167.1454815528550739 ) ) ;
#6197=DIRECTION ( 'NONE',  ( 0.3420201433256649937, 0.9396926207859097602, -0.000000000000000000 ) ) ;
#6203=VECTOR ( 'NONE', #14409, 999.9999999999998863 ) ;
#6205=ORIENTED_EDGE ( 'NONE', *, *, #9770, .F. ) ;
#6206=ORIENTED_EDGE ( 'NONE', *, *, #15548, .T. ) ;
#6208=ORIENTED_EDGE ( 'NONE', *, *, #17853, .T. ) ;
#6211=CARTESIAN_POINT ( 'NONE',  ( -71.24615306438089135, 81.36876096522922808, -167.1454815528550739 ) ) ;
#6214=DIRECTION ( 'NONE',  ( 0.000000000000000000, 0.000000000000000000, 1.000000000000000000 ) ) ;
#6219=VERTEX_POINT ( 'NONE', #17475 ) ;
#6223=LINE ( 'NONE', #531, #13924 ) ;
#6225=DIRECTION ( 'NONE',  ( 0.000000000000000000, 1.000000000000000000, 0.000000000000000000 ) ) ;
#6227=CARTESIAN_POINT ( 'NONE',  ( -68.99615306438111872, 20.24471173166267235, 15.00000000000006928 ) ) ;
#6233=ORIENTED_EDGE ( 'NONE', *, *, #5821, .F. ) ;
#6234=VECTOR ( 'NONE', #14380, 1000.000000000000000 ) ;
#6236=ORIENTED_EDGE ( 'NONE', *, *, #13469, .T. ) ;
#6238=DIRECTION ( 'NONE',  ( 0.9396926207859171987, 0.3420201433256444545, 0.000000000000000000 ) ) ;
#6248=VECTOR ( 'NONE', #4876, 1000.000000000000000 ) ;
#6249=DIRECTION ( 'NONE',  ( -0.9396926207859084279, 0.3420201433256686574, 0.000000000000000000 ) ) ;
#6256=ORIENTED_EDGE ( 'NONE', *, *, #4083, .F. ) ;
#6265=CARTESIAN_POINT ( 'NONE',  ( -71.24615306438110451, 6.859408104563811115, 15.00000000000006928 ) ) ;
#6266=DIRECTION ( 'NONE',  ( 0.3420201433256686574, 0.9396926207859084279, -0.000000000000000000 ) ) ;
#6268=EDGE_CURVE ( 'NONE', #4518, #13839, #8676, .T. ) ;
#6269=PLANE ( 'NONE',  #12900 ) ;
#6272=VECTOR ( 'NONE', #5774, 1000.000000000000000 ) ;
#6274=CARTESIAN_POINT ( 'NONE',  ( -71.24615306438077766, 97.96559495456378386, 15.00000000000006928 ) ) ;
#6277=CARTESIAN_POINT ( 'NONE',  ( -68.99615306438109030, 17.71797493813028268, -15.00000000000001421 ) ) ;
#6279=VECTOR ( 'NONE', #8208, 1000.000000000000000 ) ;
#6280=LINE ( 'NONE', #14894, #14874 ) ;
#6284=EDGE_CURVE ( 'NONE', #2737, #10339, #2970, .T. ) ;
#6293=DIRECTION ( 'NONE',  ( 1.000000000000000000, 0.000000000000000000, 0.000000000000000000 ) ) ;
#6294=ORIENTED_EDGE ( 'NONE', *, *, #3204, .T. ) ;
#6295=EDGE_CURVE ( 'NONE', #9316, #3236, #11313, .T. ) ;
#6297=ORIENTED_EDGE ( 'NONE', *, *, #4577, .F. ) ;
#6299=DIRECTION ( 'NONE',  ( -0.9396926207859097602, 0.3420201433256649381, -4.890320548438455808E-16 ) ) ;
#6303=CARTESIAN_POINT ( 'NONE',  ( -68.99615306438117557, 2.010011688130281193, -15.00000000000001421 ) ) ;
#6312=VERTEX_POINT ( 'NONE', #10003 ) ;
#6314=PLANE ( 'NONE',  #12053 ) ;
#6330=( NAMED_UNIT ( * ) PLANE_ANGLE_UNIT ( ) SI_UNIT ( $, .RADIAN. ) );
#6331=ORIENTED_EDGE ( 'NONE', *, *, #7773, .F. ) ;
#6336=ORIENTED_EDGE ( 'NONE', *, *, #7229, .T. ) ;
#6337=CARTESIAN_POINT ( 'NONE',  ( -68.99615306438074924, 120.7756765316626542, -167.1454815528550739 ) ) ;
#6338=CARTESIAN_POINT ( 'NONE',  ( -71.24615306438114715, 10.00100075456375492, -167.1454815528550739 ) ) ;
#6340=AXIS2_PLACEMENT_3D ( 'NONE', #9551, #5335, #1144 ) ;
#6341=DIRECTION ( 'NONE',  ( 1.000000000000000000, 0.000000000000000000, 0.000000000000000000 ) ) ;
#6342=LINE ( 'NONE', #16075, #17191 ) ;
#6346=VECTOR ( 'NONE', #11534, 1000.000000000000000 ) ;
#6349=DIRECTION ( 'NONE',  ( -1.000000000000000000, 0.000000000000000000, -5.204170427930409450E-16 ) ) ;
#6355=ADVANCED_FACE ( 'NONE', ( #7100 ), #16917, .T. ) ;
#6358=AXIS2_PLACEMENT_3D ( 'NONE', #6775, #15176, #12401 ) ;
#6359=CARTESIAN_POINT ( 'NONE',  ( -68.99615306438109030, 17.10311908166270456, -167.1454815528550739 ) ) ;
#6365=DIRECTION ( 'NONE',  ( 0.000000000000000000, 0.000000000000000000, 1.000000000000000000 ) ) ;
#6366=ORIENTED_EDGE ( 'NONE', *, *, #3796, .F. ) ;
#6372=EDGE_CURVE ( 'NONE', #10372, #4288, #18334, .T. ) ;
#6373=DIRECTION ( 'NONE',  ( 1.000000000000000000, 0.000000000000000000, 0.000000000000000000 ) ) ;
#6375=EDGE_CURVE ( 'NONE', #11376, #18033, #5504, .T. ) ;
#6376=VECTOR ( 'NONE', #18219, 1000.000000000000000 ) ;
#6378=AXIS2_PLACEMENT_3D ( 'NONE', #4418, #1533, #11365 ) ;
#6381=ORIENTED_EDGE ( 'NONE', *, *, #13161, .T. ) ;
#6384=EDGE_CURVE ( 'NONE', #7201, #13332, #14121, .T. ) ;
#6387=VECTOR ( 'NONE', #912, 1000.000000000000000 ) ;
#6391=PLANE ( 'NONE',  #7028 ) ;
#6392=ORIENTED_EDGE ( 'NONE', *, *, #4904, .T. ) ;
#6395=ORIENTED_EDGE ( 'NONE', *, *, #10334, .T. ) ;
#6399=ORIENTED_EDGE ( 'NONE', *, *, #2892, .T. ) ;
#6400=EDGE_CURVE ( 'NONE', #12790, #5784, #983, .T. ) ;
#6405=AXIS2_PLACEMENT_3D ( 'NONE', #8508, #5676, #7097 ) ;
#6406=CARTESIAN_POINT ( 'NONE',  ( -94.45685920050698314, -47.21335801510345220, 15.00000000000006928 ) ) ;
#6407=VECTOR ( 'NONE', #11877, 1000.000000000000000 ) ;
#6408=ORIENTED_EDGE ( 'NONE', *, *, #15877, .F. ) ;
#6411=EDGE_CURVE ( 'NONE', #1616, #5307, #12592, .T. ) ;
#6413=EDGE_LOOP ( 'NONE', ( #8226, #9205, #6208, #11206 ) ) ;
#6419=CARTESIAN_POINT ( 'NONE',  ( -71.24615306438086293, 93.93513156522925556, -167.1454815528550739 ) ) ;
#6421=VECTOR ( 'NONE', #2541, 1000.000000000000000 ) ;
#6424=PLANE ( 'NONE',  #4063 ) ;
#6425=DIRECTION ( 'NONE',  ( 0.3420201433256407353, -0.9396926207859186420, 0.000000000000000000 ) ) ;
#6430=DIRECTION ( 'NONE',  ( -0.9396926207859145341, 0.3420201433256519485, -4.890320548438481446E-16 ) ) ;
#6434=PLANE ( 'NONE',  #17915 ) ;
#6436=ORIENTED_EDGE ( 'NONE', *, *, #3008, .F. ) ;
#6439=CARTESIAN_POINT ( 'NONE',  ( -93.73308511844572877, 147.7866419848965052, -15.00000000000001421 ) ) ;
#6444=CARTESIAN_POINT ( 'NONE',  ( -71.24615306438086293, 93.93513156522925556, 15.00000000000006928 ) ) ;
#6446=LINE ( 'NONE', #10383, #2856 ) ;
#6447=CARTESIAN_POINT ( 'NONE',  ( -71.24615306438079188, 107.3903729045637192, -15.00000000000001421 ) ) ;
#6448=ORIENTED_EDGE ( 'NONE', *, *, #2895, .T. ) ;
#6451=ORIENTED_EDGE ( 'NONE', *, *, #17272, .F. ) ;
#6452=CARTESIAN_POINT ( 'NONE',  ( -71.24615306438089135, 84.51035361522924916, -15.00000000000001421 ) ) ;
#6455=VERTEX_POINT ( 'NONE', #11187 ) ;
#6460=DIRECTION ( 'NONE',  ( 0.000000000000000000, 0.000000000000000000, -1.000000000000000000 ) ) ;
#6461=VERTEX_POINT ( 'NONE', #1174 ) ;
#6463=CARTESIAN_POINT ( 'NONE',  ( -68.99615306438072082, 130.8153103381302742, -167.1454815528550739 ) ) ;
#6464=ORIENTED_EDGE ( 'NONE', *, *, #12027, .T. ) ;
#6465=CARTESIAN_POINT ( 'NONE',  ( -71.24615306438114715, 16.28418605456380419, -15.00000000000001421 ) ) ;
#6471=ORIENTED_EDGE ( 'NONE', *, *, #786, .T. ) ;
#6472=CARTESIAN_POINT ( 'NONE',  ( -71.24615306438091977, 72.83285375456371469, -15.00000000000001421 ) ) ;
#6473=ORIENTED_EDGE ( 'NONE', *, *, #5346, .T. ) ;
#6475=PLANE ( 'NONE',  #11198 ) ;
#6478=EDGE_CURVE ( 'NONE', #10978, #12641, #13796, .T. ) ;
#6479=LINE ( 'NONE', #12117, #17946 ) ;
#6482=CARTESIAN_POINT ( 'NONE',  ( -68.99615306438106188, 30.28434553813027108, -167.1454815528550739 ) ) ;
#6484=ORIENTED_EDGE ( 'NONE', *, *, #18207, .T. ) ;
#6485=DIRECTION ( 'NONE',  ( 0.9396926207859097602, 0.3420201433256649381, 4.890320548438455808E-16 ) ) ;
#6487=VERTEX_POINT ( 'NONE', #6685 ) ;
#6488=EDGE_CURVE ( 'NONE', #4573, #5742, #9484, .T. ) ;
#6492=EDGE_LOOP ( 'NONE', ( #9883, #1281, #7302, #438 ) ) ;
#6494=EDGE_LOOP ( 'NONE', ( #3430, #338, #10917, #14213 ) ) ;
#6497=CARTESIAN_POINT ( 'NONE',  ( -68.99615306438097662, 57.94382353166266597, -167.1454815528550739 ) ) ;
#6500=DIRECTION ( 'NONE',  ( 1.000000000000000000, 0.000000000000000000, 0.000000000000000000 ) ) ;
#6503=DIRECTION ( 'NONE',  ( 0.000000000000000000, 0.000000000000000000, 1.000000000000000000 ) ) ;
#6506=CARTESIAN_POINT ( 'NONE',  ( -71.24615306438076345, 131.6342433652292243, 15.00000000000006928 ) ) ;
#6508=FACE_OUTER_BOUND ( 'NONE', #15516, .T. ) ;
#6516=DIRECTION ( 'NONE',  ( 0.3420201433256444545, 0.9396926207859171987, -0.000000000000000000 ) ) ;
#6519=CARTESIAN_POINT ( 'NONE',  ( -68.99615306438094819, 64.22700883166265839, 15.00000000000006928 ) ) ;
#6521=VERTEX_POINT ( 'NONE', #8745 ) ;
#6522=ORIENTED_EDGE ( 'NONE', *, *, #11119, .F. ) ;
#6525=DIRECTION ( 'NONE',  ( 0.000000000000000000, 0.000000000000000000, 1.000000000000000000 ) ) ;
#6526=EDGE_LOOP ( 'NONE', ( #133, #16452, #9469, #2745 ) ) ;
#6529=LINE ( 'NONE', #12352, #7268 ) ;
#6530=EDGE_CURVE ( 'NONE', #455, #7544, #5834, .T. ) ;
#6533=LINE ( 'NONE', #12543, #12104 ) ;
#6536=ORIENTED_EDGE ( 'NONE', *, *, #10666, .T. ) ;
#6537=EDGE_CURVE ( 'NONE', #11339, #14706, #12784, .T. ) ;
#6540=VECTOR ( 'NONE', #1292, 1000.000000000000000 ) ;
#6544=ORIENTED_EDGE ( 'NONE', *, *, #4682, .T. ) ;
#6550=CARTESIAN_POINT ( 'NONE',  ( -68.99615306438106188, 35.95267498166268894, 15.00000000000006928 ) ) ;
#6554=DIRECTION ( 'NONE',  ( 0.000000000000000000, 0.000000000000000000, 1.000000000000000000 ) ) ;
#6555=ORIENTED_EDGE ( 'NONE', *, *, #5433, .F. ) ;
#6556=ADVANCED_BREP_SHAPE_REPRESENTATION ( '', ( #6144, #16217 ), #11478 ) ;
#6560=EDGE_LOOP ( 'NONE', ( #14615, #17110, #3075, #1028 ) ) ;
#6561=DIRECTION ( 'NONE',  ( 0.000000000000000000, 0.000000000000000000, 1.000000000000000000 ) ) ;
#6562=VERTEX_POINT ( 'NONE', #7341 ) ;
#6565=LINE ( 'NONE', #6853, #12816 ) ;
#6566=ORIENTED_EDGE ( 'NONE', *, *, #16938, .T. ) ;
#6567=VECTOR ( 'NONE', #13973, 1000.000000000000000 ) ;
#6571=VERTEX_POINT ( 'NONE', #5909 ) ;
#6572=DIRECTION ( 'NONE',  ( 1.000000000000000000, 0.000000000000000000, 0.000000000000000000 ) ) ;
#6573=FACE_OUTER_BOUND ( 'NONE', #17607, .T. ) ;
#6574=ORIENTED_EDGE ( 'NONE', *, *, #5471, .F. ) ;
#6580=ORIENTED_EDGE ( 'NONE', *, *, #18180, .T. ) ;
#6581=DIRECTION ( 'NONE',  ( 0.000000000000000000, 0.000000000000000000, 1.000000000000000000 ) ) ;
#6583=VECTOR ( 'NONE', #18025, 1000.000000000000000 ) ;
#6584=ORIENTED_EDGE ( 'NONE', *, *, #242, .F. ) ;
#6587=LINE ( 'NONE', #13620, #8435 ) ;
#6589=CARTESIAN_POINT ( 'NONE',  ( -68.99615306438072082, 127.0588618316627105, -15.00000000000001421 ) ) ;
#6592=EDGE_LOOP ( 'NONE', ( #16858, #7700, #1919, #1706 ) ) ;
#6595=ORIENTED_EDGE ( 'NONE', *, *, #4566, .F. ) ;
#6602=DIRECTION ( 'NONE',  ( 1.000000000000000000, 0.000000000000000000, 0.000000000000000000 ) ) ;
#6603=LINE ( 'NONE', #6419, #9686 ) ;
#6604=ORIENTED_EDGE ( 'NONE', *, *, #7953, .T. ) ;
#6607=FACE_OUTER_BOUND ( 'NONE', #15814, .T. ) ;
#6608=CARTESIAN_POINT ( 'NONE',  ( -71.24615306438083451, 97.96559495456375544, -15.00000000000001421 ) ) ;
#6614=CARTESIAN_POINT ( 'NONE',  ( -71.24615306438103346, 40.52805651522925245, 15.00000000000006928 ) ) ;
#6615=LINE ( 'NONE', #10730, #1233 ) ;
#6621=ORIENTED_EDGE ( 'NONE', *, *, #10655, .F. ) ;
#6622=VECTOR ( 'NONE', #12124, 1000.000000000000000 ) ;
#6624=EDGE_CURVE ( 'NONE', #5917, #10712, #1449, .T. ) ;
#6625=ORIENTED_EDGE ( 'NONE', *, *, #8889, .F. ) ;
#6626=EDGE_CURVE ( 'NONE', #10960, #9281, #6970, .T. ) ;
#6629=DIRECTION ( 'NONE',  ( -0.9396926207859084279, 0.3420201433256687684, -4.890320548438449892E-16 ) ) ;
#6632=DIRECTION ( 'NONE',  ( 0.3420201433256686574, -0.9396926207859084279, 0.000000000000000000 ) ) ;
#6634=PLANE ( 'NONE',  #1645 ) ;
#6636=ORIENTED_EDGE ( 'NONE', *, *, #7284, .F. ) ;
#6641=EDGE_CURVE ( 'NONE', #10712, #18436, #12869, .T. ) ;
#6647=ADVANCED_FACE ( 'NONE', ( #10056 ), #4161, .T. ) ;
#6648=VERTEX_POINT ( 'NONE', #17067 ) ;
#6650=VERTEX_POINT ( 'NONE', #9967 ) ;
#6653=ADVANCED_FACE ( 'NONE', ( #10137 ), #6269, .T. ) ;
#6656=DIRECTION ( 'NONE',  ( 0.000000000000000000, 1.000000000000000000, 0.000000000000000000 ) ) ;
#6664=CARTESIAN_POINT ( 'NONE',  ( -71.24615306438080609, 109.6430948152292189, -15.00000000000001421 ) ) ;
#6665=CARTESIAN_POINT ( 'NONE',  ( -68.99615306438077766, 115.1073470881302541, -167.1454815528550739 ) ) ;
#6668=CARTESIAN_POINT ( 'NONE',  ( -71.24615306438091977, 75.97444640456376419, -15.00000000000001421 ) ) ;
#6669=EDGE_LOOP ( 'NONE', ( #11604, #9846, #16670, #8571 ) ) ;
#6671=LINE ( 'NONE', #9853, #2648 ) ;
#6673=EDGE_CURVE ( 'NONE', #17240, #16781, #3205, .T. ) ;
#6675=VECTOR ( 'NONE', #12640, 1000.000000000000114 ) ;
#6677=FACE_OUTER_BOUND ( 'NONE', #11850, .T. ) ;
#6682=DIRECTION ( 'NONE',  ( 0.000000000000000000, 1.000000000000000000, 0.000000000000000000 ) ) ;
#6684=ORIENTED_EDGE ( 'NONE', *, *, #10304, .F. ) ;
#6685=CARTESIAN_POINT ( 'NONE',  ( -68.99615306438077766, 123.9172691816626610, -15.00000000000001421 ) ) ;
#6693=VECTOR ( 'NONE', #6106, 1000.000000000000000 ) ;
#6694=LINE ( 'NONE', #2590, #4895 ) ;
#6700=ORIENTED_EDGE ( 'NONE', *, *, #8492, .T. ) ;
#6702=CARTESIAN_POINT ( 'NONE',  ( -71.24615306438083451, 97.96559495456375544, -167.1454815528550739 ) ) ;
#6703=ORIENTED_EDGE ( 'NONE', *, *, #13922, .T. ) ;
#6706=CARTESIAN_POINT ( 'NONE',  ( -68.99615306438111872, 7.678341131662685726, -167.1454815528550739 ) ) ;
#6712=DIRECTION ( 'NONE',  ( 0.000000000000000000, 1.000000000000000000, 0.000000000000000000 ) ) ;
#6713=CARTESIAN_POINT ( 'NONE',  ( -68.99615306438077766, 111.3508985816626335, 15.00000000000006928 ) ) ;
#6716=ORIENTED_EDGE ( 'NONE', *, *, #8992, .F. ) ;
#6717=VECTOR ( 'NONE', #4451, 1000.000000000000000 ) ;
#6720=CARTESIAN_POINT ( 'NONE',  ( -68.99615306438117557, 4.536748481662661980, -15.00000000000001421 ) ) ;
#6721=DIRECTION ( 'NONE',  ( 0.9396926207859078728, 0.3420201433256701007, -1.086737899652989152E-16 ) ) ;
#6722=ORIENTED_EDGE ( 'NONE', *, *, #8492, .F. ) ;
#6728=VERTEX_POINT ( 'NONE', #16191 ) ;
#6738=EDGE_LOOP ( 'NONE', ( #2454, #2015, #6381, #6161 ) ) ;
#6739=DIRECTION ( 'NONE',  ( -0.9396926207859097602, 0.3420201433256649937, 0.000000000000000000 ) ) ;
#6754=FACE_OUTER_BOUND ( 'NONE', #6592, .T. ) ;
#6755=CARTESIAN_POINT ( 'NONE',  ( -68.99615306438086293, 93.11619853813030545, -167.1454815528550739 ) ) ;
#6758=LINE ( 'NONE', #1146, #9015 ) ;
#6759=ORIENTED_EDGE ( 'NONE', *, *, #1176, .T. ) ;
#6760=DIRECTION ( 'NONE',  ( 0.000000000000000000, 0.000000000000000000, -1.000000000000000000 ) ) ;
#6761=CARTESIAN_POINT ( 'NONE',  ( -68.99615306438100504, 48.51904558166270220, -15.00000000000001421 ) ) ;
#6765=DIRECTION ( 'NONE',  ( 0.9396926207859084279, 0.3420201433256686574, 0.000000000000000000 ) ) ;
#6767=EDGE_CURVE ( 'NONE', #4422, #16032, #13400, .T. ) ;
#6771=ORIENTED_EDGE ( 'NONE', *, *, #14973, .T. ) ;
#6772=EDGE_CURVE ( 'NONE', #2297, #10978, #10329, .T. ) ;
#6773=ORIENTED_EDGE ( 'NONE', *, *, #3691, .F. ) ;
#6775=CARTESIAN_POINT ( 'NONE',  ( -71.24615306438097662, 63.40807580456375803, -167.1454815528550739 ) ) ;
#6784=DIRECTION ( 'NONE',  ( 0.000000000000000000, 0.000000000000000000, -1.000000000000000000 ) ) ;
#6785=DIRECTION ( 'NONE',  ( 0.000000000000000000, 0.000000000000000000, -1.000000000000000000 ) ) ;
#6794=ORIENTED_EDGE ( 'NONE', *, *, #18024, .T. ) ;
#6798=DIRECTION ( 'NONE',  ( 0.000000000000000000, 1.000000000000000000, 0.000000000000000000 ) ) ;
#6802=ORIENTED_EDGE ( 'NONE', *, *, #5511, .F. ) ;
#6803=DIRECTION ( 'NONE',  ( 0.000000000000000000, 1.000000000000000000, 0.000000000000000000 ) ) ;
#6805=FACE_OUTER_BOUND ( 'NONE', #13102, .T. ) ;
#6807=DIRECTION ( 'NONE',  ( 0.3420201433256649937, -0.9396926207859097602, 0.000000000000000000 ) ) ;
#6809=DIRECTION ( 'NONE',  ( -0.9396926207859158664, 0.3420201433256481738, 0.000000000000000000 ) ) ;
#6815=EDGE_LOOP ( 'NONE', ( #10062, #14543, #6399, #14736 ) ) ;
#6819=CARTESIAN_POINT ( 'NONE',  ( -68.99615306438110451, 2.010011688130255436, 15.00000000000006928 ) ) ;
#6821=AXIS2_PLACEMENT_3D ( 'NONE', #17800, #13233, #12192 ) ;
#6822=LINE ( 'NONE', #1031, #15035 ) ;
#6835=ORIENTED_EDGE ( 'NONE', *, *, #7739, .F. ) ;
#6836=EDGE_LOOP ( 'NONE', ( #1013, #10120, #4164, #5118 ) ) ;
#6837=CARTESIAN_POINT ( 'NONE',  ( -68.99615306438067819, 143.3816809381303585, -167.1454815528550739 ) ) ;
#6838=CARTESIAN_POINT ( 'NONE',  ( -71.24615306438109030, 31.99214930456376038, -15.00000000000001421 ) ) ;
#6839=FACE_OUTER_BOUND ( 'NONE', #7942, .T. ) ;
#6846=CARTESIAN_POINT ( 'NONE',  ( -71.24615306438091977, 78.22716831522920700, 15.00000000000006928 ) ) ;
#6849=ORIENTED_EDGE ( 'NONE', *, *, #15471, .T. ) ;
#6850=DIRECTION ( 'NONE',  ( -0.000000000000000000, 0.000000000000000000, 1.000000000000000000 ) ) ;
#6852=VERTEX_POINT ( 'NONE', #13968 ) ;
#6853=CARTESIAN_POINT ( 'NONE',  ( -68.99615306438111872, 8.293196988130274505, -167.1454815528550739 ) ) ;
#6855=ADVANCED_FACE ( 'NONE', ( #13875 ), #11166, .T. ) ;
#6856=EDGE_CURVE ( 'NONE', #16652, #2059, #2346, .T. ) ;
#6857=AXIS2_PLACEMENT_3D ( 'NONE', #7791, #6373, #3386 ) ;
#6858=ORIENTED_EDGE ( 'NONE', *, *, #3868, .F. ) ;
#6859=VECTOR ( 'NONE', #13074, 1000.000000000000114 ) ;
#6861=FACE_OUTER_BOUND ( 'NONE', #4067, .T. ) ;
#6863=EDGE_CURVE ( 'NONE', #13855, #14048, #3762, .T. ) ;
#6864=ORIENTED_EDGE ( 'NONE', *, *, #7898, .T. ) ;
#6867=VERTEX_POINT ( 'NONE', #7967 ) ;
#6870=VERTEX_POINT ( 'NONE', #15162 ) ;
#6871=DIRECTION ( 'NONE',  ( 0.000000000000000000, 0.000000000000000000, 1.000000000000000000 ) ) ;
#6875=VECTOR ( 'NONE', #16277, 1000.000000000000000 ) ;
#6888=DIRECTION ( 'NONE',  ( 0.000000000000000000, 0.000000000000000000, 1.000000000000000000 ) ) ;
#6891=VECTOR ( 'NONE', #2241, 1000.000000000000000 ) ;
#6892=DIRECTION ( 'NONE',  ( 0.9396926207859084279, 0.3420201433256686574, 4.890320548438448905E-16 ) ) ;
#6895=DIRECTION ( 'NONE',  ( 0.000000000000000000, 1.000000000000000000, 0.000000000000000000 ) ) ;
#6896=VERTEX_POINT ( 'NONE', #15262 ) ;
#6897=DIRECTION ( 'NONE',  ( 1.000000000000000000, 0.000000000000000000, 0.000000000000000000 ) ) ;
#6898=PLANE ( 'NONE',  #13039 ) ;
#6900=PLANE ( 'NONE',  #3941 ) ;
#6902=VERTEX_POINT ( 'NONE', #6465 ) ;
#6903=MECHANICAL_DESIGN_GEOMETRIC_PRESENTATION_REPRESENTATION('',(#15852),#8691);
#6906=VECTOR ( 'NONE', #18424, 1000.000000000000000 ) ;
#6907=CARTESIAN_POINT ( 'NONE',  ( -68.99615306438077766, 114.4924912316626688, 15.00000000000006928 ) ) ;
#6909=CARTESIAN_POINT ( 'NONE',  ( -71.24615306438089135, 82.25763170456374951, -167.1454815528550739 ) ) ;
#6911=VERTEX_POINT ( 'NONE', #17876 ) ;
#6917=LINE ( 'NONE', #1576, #6081 ) ;
#6918=ORIENTED_EDGE ( 'NONE', *, *, #3317, .T. ) ;
#6919=LINE ( 'NONE', #4206, #7772 ) ;
#6925=ORIENTED_EDGE ( 'NONE', *, *, #1499, .T. ) ;
#6928=VERTEX_POINT ( 'NONE', #6846 ) ;
#6930=DIRECTION ( 'NONE',  ( 1.000000000000000000, 0.000000000000000000, 0.000000000000000000 ) ) ;
#6934=VERTEX_POINT ( 'NONE', #12385 ) ;
#6936=AXIS2_PLACEMENT_3D ( 'NONE', #14153, #12765, #5628 ) ;
#6938=CARTESIAN_POINT ( 'NONE',  ( -70.27900850916093134, -2.213358015103445098, -15.00000000000001599 ) ) ;
#6940=FACE_OUTER_BOUND ( 'NONE', #12701, .T. ) ;
#6943=DIRECTION ( 'NONE',  ( 0.000000000000000000, 1.000000000000000000, 0.000000000000000000 ) ) ;
#6945=ORIENTED_EDGE ( 'NONE', *, *, #7574, .F. ) ;
#6946=ADVANCED_FACE ( 'NONE', ( #15368 ), #12281, .T. ) ;
#6950=VECTOR ( 'NONE', #13448, 1000.000000000000000 ) ;
#6951=AXIS2_PLACEMENT_3D ( 'NONE', #1491, #3171, #11681 ) ;
#6955=VERTEX_POINT ( 'NONE', #2263 ) ;
#6956=VECTOR ( 'NONE', #16766, 1000.000000000000114 ) ;
#6957=EDGE_CURVE ( 'NONE', #14359, #17240, #5339, .T. ) ;
#6961=LINE ( 'NONE', #7144, #10893 ) ;
#6962=LINE ( 'NONE', #3960, #9991 ) ;
#6964=ORIENTED_EDGE ( 'NONE', *, *, #10196, .T. ) ;
#6966=CARTESIAN_POINT ( 'NONE',  ( -71.24615306438067819, 144.2006139652292518, -15.00000000000001421 ) ) ;
#6970=LINE ( 'NONE', #5650, #10790 ) ;
#6972=PLANE ( 'NONE',  #10525 ) ;
#6977=AXIS2_PLACEMENT_3D ( 'NONE', #2140, #12246, #10567 ) ;
#6978=VECTOR ( 'NONE', #2245, 1000.000000000000000 ) ;
#6984=VERTEX_POINT ( 'NONE', #16954 ) ;
#6986=EDGE_LOOP ( 'NONE', ( #7391, #15536, #1783, #34 ) ) ;
#6988=DIRECTION ( 'NONE',  ( 1.000000000000000000, 0.000000000000000000, 0.000000000000000000 ) ) ;
#6989=VERTEX_POINT ( 'NONE', #4408 ) ;
#6993=CARTESIAN_POINT ( 'NONE',  ( -71.24615306438080609, 115.9262801152292042, -167.1454815528550739 ) ) ;
#6995=VECTOR ( 'NONE', #9570, 1000.000000000000114 ) ;
#6996=DIRECTION ( 'NONE',  ( 0.9396926207859171987, 0.3420201433256444545, -1.086737899652999999E-16 ) ) ;
#6998=LINE ( 'NONE', #12620, #7609 ) ;
#7001=LINE ( 'NONE', #8400, #1806 ) ;
#7002=DIRECTION ( 'NONE',  ( 0.9396926207859102043, 0.3420201433256637724, 0.000000000000000000 ) ) ;
#7003=EDGE_CURVE ( 'NONE', #16011, #15896, #15823, .T. ) ;
#7005=CARTESIAN_POINT ( 'NONE',  ( -71.24615306438107609, 31.99214930456376749, -15.00000000000001421 ) ) ;
#7007=VECTOR ( 'NONE', #7083, 1000.000000000000000 ) ;
#7008=DIRECTION ( 'NONE',  ( 0.000000000000000000, 0.000000000000000000, 1.000000000000000000 ) ) ;
#7015=DIRECTION ( 'NONE',  ( 0.000000000000000000, 1.000000000000000000, 0.000000000000000000 ) ) ;
#7018=ORIENTED_EDGE ( 'NONE', *, *, #5025, .F. ) ;
#7019=EDGE_CURVE ( 'NONE', #1167, #18033, #8347, .T. ) ;
#7020=PLANE ( 'NONE',  #13852 ) ;
#7021=ORIENTED_EDGE ( 'NONE', *, *, #16353, .F. ) ;
#7023=CARTESIAN_POINT ( 'NONE',  ( -68.99615306438111872, 14.57638228813026871, -167.1454815528550739 ) ) ;
#7024=PLANE ( 'NONE',  #16230 ) ;
#7028=AXIS2_PLACEMENT_3D ( 'NONE', #12119, #793, #12201 ) ;
#7034=VERTEX_POINT ( 'NONE', #11349 ) ;
#7035=EDGE_CURVE ( 'NONE', #16976, #4613, #14059, .T. ) ;
#7037=ORIENTED_EDGE ( 'NONE', *, *, #3280, .F. ) ;
#7040=LINE ( 'NONE', #12832, #8930 ) ;
#7051=DIRECTION ( 'NONE',  ( 0.000000000000000000, 0.000000000000000000, 1.000000000000000000 ) ) ;
#7052=CARTESIAN_POINT ( 'NONE',  ( -71.24615306438106188, 34.24487121522926003, -167.1454815528550739 ) ) ;
#7053=ORIENTED_EDGE ( 'NONE', *, *, #14696, .F. ) ;
#7054=DIRECTION ( 'NONE',  ( -0.9396926207859084279, 0.3420201433256686574, 0.000000000000000000 ) ) ;
#7055=ORIENTED_EDGE ( 'NONE', *, *, #6488, .F. ) ;
#7058=FACE_OUTER_BOUND ( 'NONE', #1696, .T. ) ;
#7065=CARTESIAN_POINT ( 'NONE',  ( -71.24615306438114715, 16.28418605456380419, -167.1454815528550739 ) ) ;
#7066=FACE_OUTER_BOUND ( 'NONE', #14131, .T. ) ;
#7067=ORIENTED_EDGE ( 'NONE', *, *, #16132, .F. ) ;
#7072=DIRECTION ( 'NONE',  ( 0.9396926207859134239, 0.3420201433256546686, 4.890320548438474543E-16 ) ) ;
#7076=DIRECTION ( 'NONE',  ( 1.000000000000000000, 0.000000000000000000, 0.000000000000000000 ) ) ;
#7082=EDGE_CURVE ( 'NONE', #3118, #12199, #9942, .T. ) ;
#7083=DIRECTION ( 'NONE',  ( 0.9396926207859097602, 0.3420201433256649937, -1.086737899652991371E-16 ) ) ;
#7084=FACE_OUTER_BOUND ( 'NONE', #12266, .T. ) ;
#7087=FACE_OUTER_BOUND ( 'NONE', #2437, .T. ) ;
#7090=CARTESIAN_POINT ( 'NONE',  ( -71.24615306438097662, 62.51920506522922949, 15.00000000000006928 ) ) ;
#7092=ADVANCED_FACE ( 'NONE', ( #8445 ), #14156, .T. ) ;
#7095=PLANE ( 'NONE',  #11722 ) ;
#7097=DIRECTION ( 'NONE',  ( -0.9396926207859069846, 0.3420201433256723766, 0.000000000000000000 ) ) ;
#7100=FACE_OUTER_BOUND ( 'NONE', #14223, .T. ) ;
#7103=ORIENTED_EDGE ( 'NONE', *, *, #6863, .F. ) ;
#7104=EDGE_CURVE ( 'NONE', #14076, #12606, #2925, .T. ) ;
#7106=ORIENTED_EDGE ( 'NONE', *, *, #5247, .T. ) ;
#7110=ADVANCED_FACE ( 'NONE', ( #3104 ), #4673, .T. ) ;
#7118=CARTESIAN_POINT ( 'NONE',  ( -68.99615306438106188, 26.52789703166272162, -167.1454815528550739 ) ) ;
#7120=EDGE_CURVE ( 'NONE', #16262, #14197, #555, .T. ) ;
#7121=CARTESIAN_POINT ( 'NONE',  ( -68.99615306438070661, 127.6737176881302958, -15.00000000000001421 ) ) ;
#7122=LINE ( 'NONE', #5614, #1751 ) ;
#7127=ORIENTED_EDGE ( 'NONE', *, *, #13514, .T. ) ;
#7128=FACE_OUTER_BOUND ( 'NONE', #6986, .T. ) ;
#7137=LINE ( 'NONE', #16657, #14713 ) ;
#7138=DIRECTION ( 'NONE',  ( 0.3420201433256444545, -0.9396926207859171987, 0.000000000000000000 ) ) ;
#7140=ORIENTED_EDGE ( 'NONE', *, *, #7236, .F. ) ;
#7142=VERTEX_POINT ( 'NONE', #13114 ) ;
#7144=CARTESIAN_POINT ( 'NONE',  ( -71.24615306438109030, 31.10327856522923540, -167.1454815528550739 ) ) ;
#7146=DIRECTION ( 'NONE',  ( 0.000000000000000000, 0.000000000000000000, 1.000000000000000000 ) ) ;
#7147=LINE ( 'NONE', #1793, #17680 ) ;
#7148=ORIENTED_EDGE ( 'NONE', *, *, #6051, .F. ) ;
#7149=ORIENTED_EDGE ( 'NONE', *, *, #7406, .T. ) ;
#7151=VERTEX_POINT ( 'NONE', #14779 ) ;
#7152=DIRECTION ( 'NONE',  ( 0.000000000000000000, 0.000000000000000000, 1.000000000000000000 ) ) ;
#7154=DIRECTION ( 'NONE',  ( -0.000000000000000000, 1.000000000000000000, -0.000000000000000000 ) ) ;
#7157=ORIENTED_EDGE ( 'NONE', *, *, #4770, .F. ) ;
#7162=ORIENTED_EDGE ( 'NONE', *, *, #560, .T. ) ;
#7165=LINE ( 'NONE', #235, #3098 ) ;
#7166=VERTEX_POINT ( 'NONE', #2055 ) ;
#7169=DIRECTION ( 'NONE',  ( 0.000000000000000000, 0.000000000000000000, 1.000000000000000000 ) ) ;
#7172=PLANE ( 'NONE',  #1337 ) ;
#7173=EDGE_LOOP ( 'NONE', ( #11564, #3286, #8573, #13760 ) ) ;
#7175=AXIS2_PLACEMENT_3D ( 'NONE', #5253, #13589, #15158 ) ;
#7177=FACE_OUTER_BOUND ( 'NONE', #17570, .T. ) ;
#7181=DIRECTION ( 'NONE',  ( 0.000000000000000000, 0.000000000000000000, -1.000000000000000000 ) ) ;
#7185=VECTOR ( 'NONE', #9848, 1000.000000000000000 ) ;
#7186=VERTEX_POINT ( 'NONE', #4856 ) ;
#7187=EDGE_CURVE ( 'NONE', #17297, #794, #4495, .T. ) ;
#7193=FACE_OUTER_BOUND ( 'NONE', #9419, .T. ) ;
#7196=VECTOR ( 'NONE', #15393, 1000.000000000000000 ) ;
#7201=VERTEX_POINT ( 'NONE', #7757 ) ;
#7204=CARTESIAN_POINT ( 'NONE',  ( -68.99615306438110451, 14.57638228813026338, -15.00000000000001421 ) ) ;
#7207=ORIENTED_EDGE ( 'NONE', *, *, #7035, .T. ) ;
#7210=VERTEX_POINT ( 'NONE', #10208 ) ;
#7211=ORIENTED_EDGE ( 'NONE', *, *, #232, .F. ) ;
#7212=ADVANCED_FACE ( 'NONE', ( #10306 ), #14515, .T. ) ;
#7216=VECTOR ( 'NONE', #2664, 1000.000000000000000 ) ;
#7221=CARTESIAN_POINT ( 'NONE',  ( -68.99615306438073503, 108.8241617881302261, 15.00000000000006928 ) ) ;
#7222=ORIENTED_EDGE ( 'NONE', *, *, #13285, .F. ) ;
#7225=VERTEX_POINT ( 'NONE', #11120 ) ;
#7226=VECTOR ( 'NONE', #1243, 1000.000000000000000 ) ;
#7229=EDGE_CURVE ( 'NONE', #13353, #15968, #12439, .T. ) ;
#7231=ORIENTED_EDGE ( 'NONE', *, *, #7120, .T. ) ;
#7233=VECTOR ( 'NONE', #17569, 1000.000000000000000 ) ;
#7236=EDGE_CURVE ( 'NONE', #6571, #7186, #9606, .T. ) ;
#7238=ORIENTED_EDGE ( 'NONE', *, *, #8238, .F. ) ;
#7240=DIRECTION ( 'NONE',  ( 0.9396926207859084279, 0.3420201433256686574, -1.086737899652989892E-16 ) ) ;
#7246=ORIENTED_EDGE ( 'NONE', *, *, #8810, .F. ) ;
#7248=CARTESIAN_POINT ( 'NONE',  ( -94.45685920050698314, -47.21335801510345220, 15.00000000000006928 ) ) ;
#7253=ORIENTED_EDGE ( 'NONE', *, *, #15718, .T. ) ;
#7254=ORIENTED_EDGE ( 'NONE', *, *, #13983, .T. ) ;
#7256=ORIENTED_EDGE ( 'NONE', *, *, #3112, .T. ) ;
#7257=LINE ( 'NONE', #7427, #6693 ) ;
#7258=LINE ( 'NONE', #160, #13258 ) ;
#7264=CARTESIAN_POINT ( 'NONE',  ( -68.99615306438094819, 52.27549408813023746, 15.00000000000006928 ) ) ;
#7268=VECTOR ( 'NONE', #3631, 1000.000000000000000 ) ;
#7275=CARTESIAN_POINT ( 'NONE',  ( -68.99615306438077766, 118.2489397381302751, 15.00000000000006928 ) ) ;
#7278=CARTESIAN_POINT ( 'NONE',  ( -71.24615306438096241, 60.26648315456373695, -15.00000000000001421 ) ) ;
#7279=ORIENTED_EDGE ( 'NONE', *, *, #12315, .F. ) ;
#7283=LINE ( 'NONE', #3064, #15021 ) ;
#7284=EDGE_CURVE ( 'NONE', #8311, #5735, #1201, .T. ) ;
#7294=ORIENTED_EDGE ( 'NONE', *, *, #16212, .F. ) ;
#7297=AXIS2_PLACEMENT_3D ( 'NONE', #4134, #9839, #2444 ) ;
#7298=LINE ( 'NONE', #10106, #9271 ) ;
#7299=ORIENTED_EDGE ( 'NONE', *, *, #16354, .F. ) ;
#7302=ORIENTED_EDGE ( 'NONE', *, *, #10534, .T. ) ;
#7305=ORIENTED_EDGE ( 'NONE', *, *, #8130, .F. ) ;
#7307=AXIS2_PLACEMENT_3D ( 'NONE', #9198, #3484, #10687 ) ;
#7311=LINE ( 'NONE', #1687, #2793 ) ;
#7313=CARTESIAN_POINT ( 'NONE',  ( -68.99615306438089135, 86.21815738166266385, -15.00000000000001421 ) ) ;
#7314=DIRECTION ( 'NONE',  ( -0.9396926207859158664, 0.3420201433256481738, 0.000000000000000000 ) ) ;
#7315=ORIENTED_EDGE ( 'NONE', *, *, #903, .T. ) ;
#7316=VECTOR ( 'NONE', #4623, 1000.000000000000000 ) ;
#7319=EDGE_CURVE ( 'NONE', #14830, #7990, #10933, .T. ) ;
#7324=PLANE ( 'NONE',  #2249 ) ;
#7326=AXIS2_PLACEMENT_3D ( 'NONE', #16325, #5004, #2116 ) ;
#7328=ADVANCED_FACE ( 'NONE', ( #3811 ), #9513, .T. ) ;
#7329=ADVANCED_FACE ( 'NONE', ( #2397 ), #6900, .T. ) ;
#7330=ORIENTED_EDGE ( 'NONE', *, *, #2492, .T. ) ;
#7332=LINE ( 'NONE', #14605, #4039 ) ;
#7334=CARTESIAN_POINT ( 'NONE',  ( -68.99615306438106188, 36.56753083813027416, -167.1454815528550739 ) ) ;
#7337=AXIS2_PLACEMENT_3D ( 'NONE', #13642, #6425, #13926 ) ;
#7340=EDGE_CURVE ( 'NONE', #12366, #15968, #14557, .T. ) ;
#7341=CARTESIAN_POINT ( 'NONE',  ( -71.24615306438109030, 24.82009326522924297, -15.00000000000001421 ) ) ;
#7345=CARTESIAN_POINT ( 'NONE',  ( -68.99615306438083451, 98.78452798166264870, -15.00000000000001421 ) ) ;
#7346=EDGE_CURVE ( 'NONE', #5470, #2933, #1470, .T. ) ;
#7352=EDGE_CURVE ( 'NONE', #5195, #6193, #15705, .T. ) ;
#7362=DIRECTION ( 'NONE',  ( 0.000000000000000000, 1.000000000000000000, 0.000000000000000000 ) ) ;
#7365=DIRECTION ( 'NONE',  ( 0.3420201433256649937, -0.9396926207859097602, 0.000000000000000000 ) ) ;
#7366=CARTESIAN_POINT ( 'NONE',  ( -71.24615306438076345, 122.2094654152292037, 15.00000000000006928 ) ) ;
#7368=ORIENTED_EDGE ( 'NONE', *, *, #4667, .T. ) ;
#7371=ORIENTED_EDGE ( 'NONE', *, *, #10526, .T. ) ;
#7375=CARTESIAN_POINT ( 'NONE',  ( -71.24615306438089135, 81.36876096522922808, -15.00000000000001421 ) ) ;
#7383=CARTESIAN_POINT ( 'NONE',  ( -71.24615306438086293, 100.2183168652291982, -167.1454815528550739 ) ) ;
#7384=EDGE_LOOP ( 'NONE', ( #2601, #1212, #8871, #14257 ) ) ;
#7388=ORIENTED_EDGE ( 'NONE', *, *, #9753, .T. ) ;
#7390=ADVANCED_FACE ( 'NONE', ( #11399 ), #5768, .T. ) ;
#7391=ORIENTED_EDGE ( 'NONE', *, *, #7082, .F. ) ;
#7392=LINE ( 'NONE', #3261, #12709 ) ;
#7396=CARTESIAN_POINT ( 'NONE',  ( -71.24615306438101925, 44.55851990456372391, -15.00000000000001421 ) ) ;
#7398=CARTESIAN_POINT ( 'NONE',  ( -68.99615306438100504, 45.37745293166267402, 15.00000000000006928 ) ) ;
#7399=DIRECTION ( 'NONE',  ( 0.3420201433256520596, -0.9396926207859145341, 0.000000000000000000 ) ) ;
#7400=CARTESIAN_POINT ( 'NONE',  ( -71.24615306438107609, 25.70896400456377506, -15.00000000000001421 ) ) ;
#7401=ORIENTED_EDGE ( 'NONE', *, *, #4891, .T. ) ;
#7402=DIRECTION ( 'NONE',  ( -1.000000000000000000, 0.000000000000000000, 0.000000000000000000 ) ) ;
#7406=EDGE_CURVE ( 'NONE', #10257, #15993, #2887, .T. ) ;
#7410=ORIENTED_EDGE ( 'NONE', *, *, #14416, .F. ) ;
#7411=ORIENTED_EDGE ( 'NONE', *, *, #10304, .T. ) ;
#7421=EDGE_CURVE ( 'NONE', #8426, #18002, #12803, .T. ) ;
#7422=ORIENTED_EDGE ( 'NONE', *, *, #8952, .F. ) ;
#7426=ADVANCED_FACE ( 'NONE', ( #7177 ), #10159, .T. ) ;
#7427=CARTESIAN_POINT ( 'NONE',  ( -71.24615306438083451, 97.07672421522921979, 15.00000000000006928 ) ) ;
#7430=VERTEX_POINT ( 'NONE', #4373 ) ;
#7433=LINE ( 'NONE', #11745, #935 ) ;
#7436=EDGE_CURVE ( 'NONE', #6896, #13777, #15864, .T. ) ;
#7437=LINE ( 'NONE', #13246, #13468 ) ;
#7444=PLANE ( 'NONE',  #11808 ) ;
#7447=ORIENTED_EDGE ( 'NONE', *, *, #8710, .F. ) ;
#7449=EDGE_CURVE ( 'NONE', #7663, #13644, #16314, .T. ) ;
#7452=CARTESIAN_POINT ( 'NONE',  ( -71.24615306438091977, 75.08557566522922855, -15.00000000000001421 ) ) ;
#7453=ORIENTED_EDGE ( 'NONE', *, *, #17392, .T. ) ;
#7465=CARTESIAN_POINT ( 'NONE',  ( -71.24615306438109030, 27.96168591522921076, -15.00000000000001421 ) ) ;
#7467=EDGE_LOOP ( 'NONE', ( #213, #10589, #6918, #500 ) ) ;
#7469=VECTOR ( 'NONE', #8720, 1000.000000000000000 ) ;
#7471=ORIENTED_EDGE ( 'NONE', *, *, #7664, .T. ) ;
#7472=VECTOR ( 'NONE', #639, 1000.000000000000000 ) ;
#7473=ORIENTED_EDGE ( 'NONE', *, *, #8822, .T. ) ;
#7478=VECTOR ( 'NONE', #8326, 1000.000000000000000 ) ;
#7480=FACE_OUTER_BOUND ( 'NONE', #13878, .T. ) ;
#7483=EDGE_CURVE ( 'NONE', #4400, #2613, #10706, .T. ) ;
#7489=LINE ( 'NONE', #13206, #8479 ) ;
#7490=DIRECTION ( 'NONE',  ( 1.000000000000000000, 0.000000000000000000, 0.000000000000000000 ) ) ;
#7491=ORIENTED_EDGE ( 'NONE', *, *, #9376, .F. ) ;
#7493=LINE ( 'NONE', #1697, #4340 ) ;
#7494=CARTESIAN_POINT ( 'NONE',  ( -71.24615306438103346, 47.70011255456374499, -15.00000000000001421 ) ) ;
#7496=VECTOR ( 'NONE', #4372, 1000.000000000000000 ) ;
#7498=ORIENTED_EDGE ( 'NONE', *, *, #2640, .F. ) ;
#7501=EDGE_CURVE ( 'NONE', #11410, #10310, #12207, .T. ) ;
#7503=VERTEX_POINT ( 'NONE', #13423 ) ;
#7511=VECTOR ( 'NONE', #2642, 1000.000000000000000 ) ;
#7512=VERTEX_POINT ( 'NONE', #2198 ) ;
#7513=CARTESIAN_POINT ( 'NONE',  ( -68.99615306438089135, 83.69142058813029905, 15.00000000000006928 ) ) ;
#7514=ORIENTED_EDGE ( 'NONE', *, *, #17064, .F. ) ;
#7517=VECTOR ( 'NONE', #9410, 1000.000000000000000 ) ;
#7523=CARTESIAN_POINT ( 'NONE',  ( -68.99615306438094819, 54.80223088166269463, -15.00000000000001421 ) ) ;
#7525=EDGE_CURVE ( 'NONE', #17396, #16262, #7632, .T. ) ;
#7531=DIRECTION ( 'NONE',  ( 0.9396926207859097602, 0.3420201433256649937, 0.000000000000000000 ) ) ;
#7542=VECTOR ( 'NONE', #13050, 1000.000000000000000 ) ;
#7544=VERTEX_POINT ( 'NONE', #4712 ) ;
#7548=VECTOR ( 'NONE', #10296, 1000.000000000000000 ) ;
#7549=DIRECTION ( 'NONE',  ( 0.3420201433256686574, 0.9396926207859084279, -0.000000000000000000 ) ) ;
#7551=LINE ( 'NONE', #14487, #17117 ) ;
#7552=EDGE_CURVE ( 'NONE', #1261, #5560, #13249, .T. ) ;
#7553=CARTESIAN_POINT ( 'NONE',  ( -68.99615306438111872, 10.81993378166265529, -167.1454815528550739 ) ) ;
#7560=EDGE_CURVE ( 'NONE', #3332, #5163, #17724, .T. ) ;
#7563=ADVANCED_FACE ( 'NONE', ( #9215 ), #3313, .T. ) ;
#7564=DIRECTION ( 'NONE',  ( -0.9396926207859084279, 0.3420201433256686574, 1.086737899652989892E-16 ) ) ;
#7565=ORIENTED_EDGE ( 'NONE', *, *, #17888, .F. ) ;
#7571=ORIENTED_EDGE ( 'NONE', *, *, #15339, .T. ) ;
#7574=EDGE_CURVE ( 'NONE', #2512, #4254, #2001, .T. ) ;
#7577=ADVANCED_FACE ( 'NONE', ( #6573 ), #10896, .T. ) ;
#7579=PLANE ( 'NONE',  #4947 ) ;
#7581=DIRECTION ( 'NONE',  ( -0.004825104377941397994, -0.9999883591161159435, 0.000000000000000000 ) ) ;
#7582=AXIS2_PLACEMENT_3D ( 'NONE', #18212, #6988, #1189 ) ;
#7583=CARTESIAN_POINT ( 'NONE',  ( -68.99615306438080609, 108.2093059316626693, 15.00000000000006928 ) ) ;
#7587=CARTESIAN_POINT ( 'NONE',  ( -71.24615306438076345, 119.0678727652292253, -167.1454815528550739 ) ) ;
#7591=CARTESIAN_POINT ( 'NONE',  ( -70.27900850916093134, -47.21335801510345220, 15.00000000000008171 ) ) ;
#7592=CARTESIAN_POINT ( 'NONE',  ( -71.24615306438074924, 110.5319655545637687, 15.00000000000006928 ) ) ;
#7595=ORIENTED_EDGE ( 'NONE', *, *, #7806, .T. ) ;
#7599=CARTESIAN_POINT ( 'NONE',  ( -68.99615306438111872, 20.85956758813031797, -167.1454815528550739 ) ) ;
#7609=VECTOR ( 'NONE', #8666, 1000.000000000000000 ) ;
#7611=VECTOR ( 'NONE', #7666, 1000.000000000000000 ) ;
#7612=PLANE ( 'NONE',  #1777 ) ;
#7613=VERTEX_POINT ( 'NONE', #5179 ) ;
#7615=ORIENTED_EDGE ( 'NONE', *, *, #17064, .T. ) ;
#7616=EDGE_CURVE ( 'NONE', #3179, #5307, #3580, .T. ) ;
#7620=EDGE_CURVE ( 'NONE', #1345, #6650, #2094, .T. ) ;
#7628=CARTESIAN_POINT ( 'NONE',  ( -68.99615306438083451, 96.25779118813026969, -167.1454815528550739 ) ) ;
#7631=EDGE_LOOP ( 'NONE', ( #3962, #14623, #15735, #5842 ) ) ;
#7632=LINE ( 'NONE', #14820, #7517 ) ;
#7642=CARTESIAN_POINT ( 'NONE',  ( -71.24615306438117557, 5.970537365229261262, -15.00000000000001421 ) ) ;
#7644=LINE ( 'NONE', #10641, #17192 ) ;
#7648=DIRECTION ( 'NONE',  ( 0.9396926207859171987, 0.3420201433256444545, -1.086737899652999999E-16 ) ) ;
#7649=CARTESIAN_POINT ( 'NONE',  ( -71.24615306438091977, 71.94398301522919326, -167.1454815528550739 ) ) ;
#7653=ORIENTED_EDGE ( 'NONE', *, *, #15515, .F. ) ;
#7656=ORIENTED_EDGE ( 'NONE', *, *, #15545, .F. ) ;
#7661=ORIENTED_EDGE ( 'NONE', *, *, #14516, .T. ) ;
#7663=VERTEX_POINT ( 'NONE', #3396 ) ;
#7664=EDGE_CURVE ( 'NONE', #8569, #12366, #10512, .T. ) ;
#7666=DIRECTION ( 'NONE',  ( 0.000000000000000000, 0.000000000000000000, 1.000000000000000000 ) ) ;
#7670=CARTESIAN_POINT ( 'NONE',  ( -71.24615306438087714, 69.69126110456377887, 15.00000000000006928 ) ) ;
#7674=CARTESIAN_POINT ( 'NONE',  ( -68.99615306438080609, 108.2093059316626693, -167.1454815528550739 ) ) ;
#7676=CARTESIAN_POINT ( 'NONE',  ( -68.99615306438072082, 127.6737176881302958, -167.1454815528550739 ) ) ;
#7679=DIRECTION ( 'NONE',  ( 0.9396926207859171987, 0.3420201433256445100, 4.890320548438495251E-16 ) ) ;
#7680=EDGE_CURVE ( 'NONE', #16077, #3860, #16491, .T. ) ;
#7684=EDGE_CURVE ( 'NONE', #9812, #8044, #2274, .T. ) ;
#7686=CARTESIAN_POINT ( 'NONE',  ( -71.24615306438089135, 84.51035361522924916, -167.1454815528550739 ) ) ;
#7687=CARTESIAN_POINT ( 'NONE',  ( -68.99615306438094819, 54.80223088166269463, -167.1454815528550739 ) ) ;
#7690=ORIENTED_EDGE ( 'NONE', *, *, #17836, .F. ) ;
#7700=ORIENTED_EDGE ( 'NONE', *, *, #7891, .T. ) ;
#7701=ORIENTED_EDGE ( 'NONE', *, *, #4788, .F. ) ;
#7706=DIRECTION ( 'NONE',  ( 0.000000000000000000, 0.000000000000000000, 1.000000000000000000 ) ) ;
#7707=DIRECTION ( 'NONE',  ( 0.000000000000000000, 1.000000000000000000, 0.000000000000000000 ) ) ;
#7712=CARTESIAN_POINT ( 'NONE',  ( -68.99615306438117557, 5.151604338130305827, 15.00000000000006928 ) ) ;
#7713=VERTEX_POINT ( 'NONE', #4155 ) ;
#7720=ORIENTED_EDGE ( 'NONE', *, *, #11353, .T. ) ;
#7721=DIRECTION ( 'NONE',  ( 0.9396926207859092051, 0.3420201433256663259, 0.000000000000000000 ) ) ;
#7727=VECTOR ( 'NONE', #16989, 1000.000000000000000 ) ;
#7739=EDGE_CURVE ( 'NONE', #12217, #13329, #12495, .T. ) ;
#7742=ORIENTED_EDGE ( 'NONE', *, *, #10405, .F. ) ;
#7745=VECTOR ( 'NONE', #15195, 1000.000000000000114 ) ;
#7746=CARTESIAN_POINT ( 'NONE',  ( -68.99615306438067819, 146.5232735881302801, -167.1454815528550739 ) ) ;
#7747=ORIENTED_EDGE ( 'NONE', *, *, #16977, .T. ) ;
#7749=DIRECTION ( 'NONE',  ( 0.000000000000000000, 0.000000000000000000, 1.000000000000000000 ) ) ;
#7751=CARTESIAN_POINT ( 'NONE',  ( -68.99615306438099083, 45.99230878813025925, -15.00000000000001421 ) ) ;
#7754=DIRECTION ( 'NONE',  ( 0.000000000000000000, 1.000000000000000000, 0.000000000000000000 ) ) ;
#7756=AXIS2_PLACEMENT_3D ( 'NONE', #7676, #2057, #6249 ) ;
#7757=CARTESIAN_POINT ( 'NONE',  ( -71.24615306438086293, 87.65194626522927024, -15.00000000000001421 ) ) ;
#7760=APPLICATION_CONTEXT ( 'automotive_design' ) ;
#7766=FACE_OUTER_BOUND ( 'NONE', #6738, .T. ) ;
#7770=VECTOR ( 'NONE', #5880, 1000.000000000000114 ) ;
#7772=VECTOR ( 'NONE', #8608, 1000.000000000000000 ) ;
#7773=EDGE_CURVE ( 'NONE', #16605, #17396, #3776, .T. ) ;
#7777=ADVANCED_FACE ( 'NONE', ( #7066 ), #18385, .T. ) ;
#7779=PLANE ( 'NONE',  #16198 ) ;
#7782=PLANE ( 'NONE',  #7175 ) ;
#7783=ADVANCED_FACE ( 'NONE', ( #977 ), #11366, .T. ) ;
#7790=AXIS2_PLACEMENT_3D ( 'NONE', #15129, #17840, #8016 ) ;
#7791=CARTESIAN_POINT ( 'NONE',  ( -68.99615306438106188, 23.38630438166269698, -167.1454815528550739 ) ) ;
#7794=EDGE_CURVE ( 'NONE', #11906, #2577, #15177, .T. ) ;
#7795=AXIS2_PLACEMENT_3D ( 'NONE', #1559, #1653, #17442 ) ;
#7796=LINE ( 'NONE', #16661, #16365 ) ;
#7797=ORIENTED_EDGE ( 'NONE', *, *, #4361, .T. ) ;
#7799=VECTOR ( 'NONE', #7072, 1000.000000000000114 ) ;
#7806=EDGE_CURVE ( 'NONE', #1716, #17497, #5644, .T. ) ;
#7808=EDGE_LOOP ( 'NONE', ( #633, #11879, #866, #17954 ) ) ;
#7810=VERTEX_POINT ( 'NONE', #3961 ) ;
#7811=DIRECTION ( 'NONE',  ( -0.9396926207859022107, 0.3420201433256853663, 0.000000000000000000 ) ) ;
#7812=LINE ( 'NONE', #7989, #3951 ) ;
#7813=LINE ( 'NONE', #10708, #15386 ) ;
#7816=EDGE_LOOP ( 'NONE', ( #6555, #8062, #17672, #17105 ) ) ;
#7818=LINE ( 'NONE', #13533, #2197 ) ;
#7820=EDGE_CURVE ( 'NONE', #4896, #13281, #13789, .T. ) ;
#7822=ORIENTED_EDGE ( 'NONE', *, *, #6068, .F. ) ;
#7826=ORIENTED_EDGE ( 'NONE', *, *, #16457, .F. ) ;
#7827=DIRECTION ( 'NONE',  ( -0.9396926207859097602, 0.3420201433256649937, 1.086737899652991371E-16 ) ) ;
#7829=VECTOR ( 'NONE', #17645, 1000.000000000000000 ) ;
#7830=DIRECTION ( 'NONE',  ( 0.000000000000000000, 0.000000000000000000, 1.000000000000000000 ) ) ;
#7831=CARTESIAN_POINT ( 'NONE',  ( -68.99615306438086293, 92.50134268166266338, -15.00000000000001421 ) ) ;
#7836=ORIENTED_EDGE ( 'NONE', *, *, #15548, .F. ) ;
#7838=CARTESIAN_POINT ( 'NONE',  ( -68.99615306438080609, 105.6825691381303045, -167.1454815528550739 ) ) ;
#7839=( NAMED_UNIT ( * ) SI_UNIT ( $, .STERADIAN. ) SOLID_ANGLE_UNIT ( ) );
#7840=ORIENTED_EDGE ( 'NONE', *, *, #18366, .T. ) ;
#7844=VECTOR ( 'NONE', #13596, 1000.000000000000227 ) ;
#7846=ORIENTED_EDGE ( 'NONE', *, *, #18140, .F. ) ;
#7847=DIRECTION ( 'NONE',  ( 0.000000000000000000, 0.000000000000000000, 1.000000000000000000 ) ) ;
#7848=DIRECTION ( 'NONE',  ( 0.3420201433256444545, -0.9396926207859171987, 0.000000000000000000 ) ) ;
#7849=CARTESIAN_POINT ( 'NONE',  ( -68.99615306438087714, 86.83301323813024908, -15.00000000000001421 ) ) ;
#7852=DIRECTION ( 'NONE',  ( 0.9396926207859171987, 0.3420201433256444545, -1.086737899652999999E-16 ) ) ;
#7854=ORIENTED_EDGE ( 'NONE', *, *, #16225, .T. ) ;
#7859=ORIENTED_EDGE ( 'NONE', *, *, #8822, .F. ) ;
#7861=DIRECTION ( 'NONE',  ( 0.000000000000000000, 1.000000000000000000, 0.000000000000000000 ) ) ;
#7862=ORIENTED_EDGE ( 'NONE', *, *, #11873, .F. ) ;
#7869=LINE ( 'NONE', #3475, #17988 ) ;
#7871=CARTESIAN_POINT ( 'NONE',  ( -68.99615306438120399, -1.746436818337276931, 15.00000000000006928 ) ) ;
#7873=EDGE_CURVE ( 'NONE', #773, #15101, #16871, .T. ) ;
#7874=DIRECTION ( 'NONE',  ( 0.000000000000000000, 1.000000000000000000, 0.000000000000000000 ) ) ;
#7882=ORIENTED_EDGE ( 'NONE', *, *, #16573, .T. ) ;
#7884=ORIENTED_EDGE ( 'NONE', *, *, #9260, .T. ) ;
#7885=EDGE_CURVE ( 'NONE', #16082, #8820, #298, .T. ) ;
#7886=VECTOR ( 'NONE', #14835, 1000.000000000000000 ) ;
#7887=CARTESIAN_POINT ( 'NONE',  ( -68.99615306438097662, 57.94382353166266597, 15.00000000000006928 ) ) ;
#7891=EDGE_CURVE ( 'NONE', #12615, #11278, #17057, .T. ) ;
#7892=EDGE_LOOP ( 'NONE', ( #13127, #12312, #18356, #11192 ) ) ;
#7893=LINE ( 'NONE', #3684, #2215 ) ;
#7894=CARTESIAN_POINT ( 'NONE',  ( -68.99615306438083451, 101.9261206316626698, -167.1454815528550739 ) ) ;
#7897=EDGE_LOOP ( 'NONE', ( #5192, #11869, #9662, #13652 ) ) ;
#7898=EDGE_CURVE ( 'NONE', #2089, #18486, #7147, .T. ) ;
#7902=CARTESIAN_POINT ( 'NONE',  ( -71.24615306438084872, 79.11603905456375685, 15.00000000000006928 ) ) ;
#7903=ORIENTED_EDGE ( 'NONE', *, *, #16690, .T. ) ;
#7908=DIRECTION ( 'NONE',  ( 0.000000000000000000, 1.000000000000000000, 0.000000000000000000 ) ) ;
#7909=EDGE_CURVE ( 'NONE', #10207, #10372, #13219, .T. ) ;
#7911=FACE_OUTER_BOUND ( 'NONE', #8506, .T. ) ;
#7916=EDGE_CURVE ( 'NONE', #7225, #14192, #10223, .T. ) ;
#7921=DIRECTION ( 'NONE',  ( -0.9396926207859084279, 0.3420201433256687684, 1.086737899652989769E-16 ) ) ;
#7926=EDGE_CURVE ( 'NONE', #6312, #17387, #4605, .T. ) ;
#7934=VECTOR ( 'NONE', #9059, 1000.000000000000000 ) ;
#7935=CARTESIAN_POINT ( 'NONE',  ( -71.24615306438097662, 59.37761241522920841, -15.00000000000001421 ) ) ;
#7940=CARTESIAN_POINT ( 'NONE',  ( -68.99615306438097662, 58.55867938813025830, -15.00000000000001421 ) ) ;
#7942=EDGE_LOOP ( 'NONE', ( #10784, #17136, #1158, #10473 ) ) ;
#7943=EDGE_LOOP ( 'NONE', ( #6625, #8273, #4843, #15400 ) ) ;
#7944=LINE ( 'NONE', #7746, #15928 ) ;
#7947=CARTESIAN_POINT ( 'NONE',  ( -68.99615306438060713, 143.3816809381303301, 15.00000000000006928 ) ) ;
#7953=EDGE_CURVE ( 'NONE', #2278, #11754, #3121, .T. ) ;
#7955=CARTESIAN_POINT ( 'NONE',  ( -68.99615306438072082, 140.2400882881302948, -15.00000000000001421 ) ) ;
#7961=LINE ( 'NONE', #6359, #15354 ) ;
#7962=CARTESIAN_POINT ( 'NONE',  ( -68.99615306438089135, 67.36860148166267948, -15.00000000000001421 ) ) ;
#7963=DIRECTION ( 'NONE',  ( 0.000000000000000000, 0.000000000000000000, -1.000000000000000000 ) ) ;
#7967=CARTESIAN_POINT ( 'NONE',  ( -71.24615306438070661, 147.3422066152292871, -15.00000000000001421 ) ) ;
#7971=ORIENTED_EDGE ( 'NONE', *, *, #16116, .F. ) ;
#7972=CARTESIAN_POINT ( 'NONE',  ( -71.24615306438103346, 41.41692725456378099, -167.1454815528550739 ) ) ;
#7974=DIRECTION ( 'NONE',  ( -0.9396926207859167546, 0.3420201433256455648, -4.890320548438493279E-16 ) ) ;
#7976=EDGE_CURVE ( 'NONE', #18067, #1261, #14265, .T. ) ;
#7977=ORIENTED_EDGE ( 'NONE', *, *, #11005, .T. ) ;
#7981=CARTESIAN_POINT ( 'NONE',  ( -68.99615306438110451, 11.43478963813029381, -15.00000000000001421 ) ) ;
#7987=ORIENTED_EDGE ( 'NONE', *, *, #13606, .T. ) ;
#7989=CARTESIAN_POINT ( 'NONE',  ( -71.24615306438114715, 15.39531531522927921, 15.00000000000006928 ) ) ;
#7990=VERTEX_POINT ( 'NONE', #1704 ) ;
#7993=ADVANCED_FACE ( 'NONE', ( #8740 ), #2936, .T. ) ;
#7998=DIRECTION ( 'NONE',  ( 0.9396926207859185309, 0.3420201433256406798, 4.890320548438501168E-16 ) ) ;
#7999=DIRECTION ( 'NONE',  ( 0.000000000000000000, 0.000000000000000000, 1.000000000000000000 ) ) ;
#8000=EDGE_CURVE ( 'NONE', #1867, #4994, #12963, .T. ) ;
#8004=EDGE_CURVE ( 'NONE', #11612, #13941, #1624, .T. ) ;
#8007=DIRECTION ( 'NONE',  ( 0.000000000000000000, 0.000000000000000000, -1.000000000000000000 ) ) ;
#8008=DIRECTION ( 'NONE',  ( 0.3420201433256686574, -0.9396926207859084279, 0.000000000000000000 ) ) ;
#8010=CARTESIAN_POINT ( 'NONE',  ( -68.99615306438091977, 77.40823528813029952, -167.1454815528550739 ) ) ;
#8011=EDGE_CURVE ( 'NONE', #15821, #15944, #15070, .T. ) ;
#8014=ORIENTED_EDGE ( 'NONE', *, *, #8358, .T. ) ;
#8015=LINE ( 'NONE', #3726, #16291 ) ;
#8016=DIRECTION ( 'NONE',  ( -0.9396926207859097602, 0.3420201433256649937, 0.000000000000000000 ) ) ;
#8018=ADVANCED_FACE ( 'NONE', ( #11820 ), #14697, .T. ) ;
#8022=ORIENTED_EDGE ( 'NONE', *, *, #14579, .T. ) ;
#8025=EDGE_LOOP ( 'NONE', ( #7836, #13504, #14531, #17415 ) ) ;
#8027=CARTESIAN_POINT ( 'NONE',  ( -68.99615306438077766, 111.9657544381302330, -167.1454815528550739 ) ) ;
#8032=DIRECTION ( 'NONE',  ( 0.000000000000000000, 1.000000000000000000, 0.000000000000000000 ) ) ;
#8039=FACE_OUTER_BOUND ( 'NONE', #17196, .T. ) ;
#8044=VERTEX_POINT ( 'NONE', #11895 ) ;
#8046=LINE ( 'NONE', #16561, #4844 ) ;
#8050=CARTESIAN_POINT ( 'NONE',  ( -71.24615306438067819, 144.2006139652292518, 15.00000000000006928 ) ) ;
#8052=DIRECTION ( 'NONE',  ( 0.000000000000000000, 1.000000000000000000, 0.000000000000000000 ) ) ;
#8057=ORIENTED_EDGE ( 'NONE', *, *, #14385, .F. ) ;
#8059=DIRECTION ( 'NONE',  ( 0.000000000000000000, 1.000000000000000000, 0.000000000000000000 ) ) ;
#8060=ORIENTED_EDGE ( 'NONE', *, *, #5994, .F. ) ;
#8062=ORIENTED_EDGE ( 'NONE', *, *, #12747, .T. ) ;
#8065=VECTOR ( 'NONE', #5019, 1000.000000000000000 ) ;
#8066=EDGE_CURVE ( 'NONE', #18486, #8399, #3284, .T. ) ;
#8069=DIRECTION ( 'NONE',  ( 0.000000000000000000, 0.000000000000000000, -1.000000000000000000 ) ) ;
#8074=VECTOR ( 'NONE', #11523, 1000.000000000000000 ) ;
#8075=LINE ( 'NONE', #12019, #15377 ) ;
#8076=ORIENTED_EDGE ( 'NONE', *, *, #7684, .F. ) ;
#8078=LINE ( 'NONE', #16775, #5093 ) ;
#8080=AXIS2_PLACEMENT_3D ( 'NONE', #628, #17831, #8007 ) ;
#8081=ORIENTED_EDGE ( 'NONE', *, *, #14440, .T. ) ;
#8084=CARTESIAN_POINT ( 'NONE',  ( -71.24615306438097662, 59.37761241522920841, 15.00000000000006928 ) ) ;
#8085=VERTEX_POINT ( 'NONE', #16372 ) ;
#8087=CARTESIAN_POINT ( 'NONE',  ( -68.99615306438111872, 20.85956758813031797, 15.00000000000006928 ) ) ;
#8091=VECTOR ( 'NONE', #15099, 1000.000000000000000 ) ;
#8092=CARTESIAN_POINT ( 'NONE',  ( -68.99615306438103346, 33.42593818813029571, -167.1454815528550739 ) ) ;
#8100=EDGE_CURVE ( 'NONE', #5068, #10635, #10772, .T. ) ;
#8101=CARTESIAN_POINT ( 'NONE',  ( -68.99615306438099083, 36.56753083813024574, 15.00000000000006928 ) ) ;
#8105=DIRECTION ( 'NONE',  ( 0.3420201433256635504, 0.9396926207859103153, -0.000000000000000000 ) ) ;
#8107=ORIENTED_EDGE ( 'NONE', *, *, #9260, .F. ) ;
#8110=VECTOR ( 'NONE', #11898, 1000.000000000000000 ) ;
#8112=LINE ( 'NONE', #16526, #16131 ) ;
#8118=EDGE_CURVE ( 'NONE', #4518, #6934, #3377, .T. ) ;
#8120=ADVANCED_FACE ( 'NONE', ( #3657 ), #7779, .T. ) ;
#8123=ORIENTED_EDGE ( 'NONE', *, *, #10634, .T. ) ;
#8126=DIRECTION ( 'NONE',  ( 0.000000000000000000, 1.000000000000000000, 0.000000000000000000 ) ) ;
#8130=EDGE_CURVE ( 'NONE', #18088, #3227, #17685, .T. ) ;
#8131=FACE_OUTER_BOUND ( 'NONE', #15757, .T. ) ;
#8132=EDGE_CURVE ( 'NONE', #10671, #3670, #1986, .T. ) ;
#8136=AXIS2_PLACEMENT_3D ( 'NONE', #7599, #12091, #10681 ) ;
#8137=ADVANCED_FACE ( 'NONE', ( #4874 ), #10594, .T. ) ;
#8139=DIRECTION ( 'NONE',  ( 1.000000000000000000, 0.000000000000000000, 0.000000000000000000 ) ) ;
#8143=VECTOR ( 'NONE', #14255, 1000.000000000000000 ) ;
#8147=ADVANCED_FACE ( 'NONE', ( #2072 ), #15258, .T. ) ;
#8150=VECTOR ( 'NONE', #1486, 1000.000000000000000 ) ;
#8152=FACE_OUTER_BOUND ( 'NONE', #6494, .T. ) ;
#8153=LINE ( 'NONE', #12276, #4012 ) ;
#8154=LINE ( 'NONE', #16852, #11453 ) ;
#8161=CARTESIAN_POINT ( 'NONE',  ( -71.24615306438100504, 49.95283446522918780, -167.1454815528550739 ) ) ;
#8162=LINE ( 'NONE', #10876, #13194 ) ;
#8164=VERTEX_POINT ( 'NONE', #87 ) ;
#8166=LINE ( 'NONE', #5446, #6567 ) ;
#8167=EDGE_LOOP ( 'NONE', ( #15943, #8123, #3773, #4420 ) ) ;
#8169=ORIENTED_EDGE ( 'NONE', *, *, #4143, .T. ) ;
#8170=EDGE_CURVE ( 'NONE', #15520, #6455, #2556, .T. ) ;
#8175=PLANE ( 'NONE',  #6358 ) ;
#8179=LINE ( 'NONE', #14080, #16759 ) ;
#8181=ORIENTED_EDGE ( 'NONE', *, *, #2539, .T. ) ;
#8183=FACE_OUTER_BOUND ( 'NONE', #1887, .T. ) ;
#8191=FACE_OUTER_BOUND ( 'NONE', #14525, .T. ) ;
#8192=EDGE_CURVE ( 'NONE', #18188, #10024, #12561, .T. ) ;
#8193=DIRECTION ( 'NONE',  ( 0.000000000000000000, 1.000000000000000000, 0.000000000000000000 ) ) ;
#8204=FACE_OUTER_BOUND ( 'NONE', #13611, .T. ) ;
#8206=ORIENTED_EDGE ( 'NONE', *, *, #12829, .F. ) ;
#8208=DIRECTION ( 'NONE',  ( 0.000000000000000000, 1.000000000000000000, 0.000000000000000000 ) ) ;
#8210=LINE ( 'NONE', #8010, #464 ) ;
#8212=DIRECTION ( 'NONE',  ( -0.9396926207859084279, 0.3420201433256686574, 0.000000000000000000 ) ) ;
#8213=ORIENTED_EDGE ( 'NONE', *, *, #600, .T. ) ;
#8216=AXIS2_PLACEMENT_3D ( 'NONE', #18458, #14147, #5623 ) ;
#8221=ORIENTED_EDGE ( 'NONE', *, *, #6400, .F. ) ;
#8222=ORIENTED_EDGE ( 'NONE', *, *, #15334, .T. ) ;
#8226=ORIENTED_EDGE ( 'NONE', *, *, #4222, .F. ) ;
#8228=VECTOR ( 'NONE', #9227, 1000.000000000000000 ) ;
#8229=LINE ( 'NONE', #14032, #15981 ) ;
#8232=ORIENTED_EDGE ( 'NONE', *, *, #4450, .T. ) ;
#8235=CARTESIAN_POINT ( 'NONE',  ( -68.99615306438094819, 55.41708673813027985, -15.00000000000001421 ) ) ;
#8237=ORIENTED_EDGE ( 'NONE', *, *, #4310, .F. ) ;
#8238=EDGE_CURVE ( 'NONE', #12144, #4238, #3940, .T. ) ;
#8240=FACE_OUTER_BOUND ( 'NONE', #7631, .T. ) ;
#8241=DIRECTION ( 'NONE',  ( -0.9396926207859171987, 0.3420201433256444545, 1.086737899652999999E-16 ) ) ;
#8242=ORIENTED_EDGE ( 'NONE', *, *, #7449, .F. ) ;
#8246=VECTOR ( 'NONE', #14923, 1000.000000000000114 ) ;
#8247=ORIENTED_EDGE ( 'NONE', *, *, #5033, .F. ) ;
#8248=ORIENTED_EDGE ( 'NONE', *, *, #1188, .T. ) ;
#8249=ADVANCED_FACE ( 'NONE', ( #7193 ), #2639, .T. ) ;
#8252=PLANE ( 'NONE',  #4030 ) ;
#8254=CARTESIAN_POINT ( 'NONE',  ( -68.99615306438097662, 61.08541618166268705, -15.00000000000001421 ) ) ;
#8256=EDGE_CURVE ( 'NONE', #11278, #3670, #12913, .T. ) ;
#8257=LINE ( 'NONE', #8628, #8361 ) ;
#8258=DIRECTION ( 'NONE',  ( 0.000000000000000000, 1.000000000000000000, 0.000000000000000000 ) ) ;
#8259=ORIENTED_EDGE ( 'NONE', *, *, #14956, .T. ) ;
#8266=EDGE_CURVE ( 'NONE', #9970, #15423, #8154, .T. ) ;
#8267=ADVANCED_FACE ( 'NONE', ( #16744 ), #5252, .T. ) ;
#8270=LINE ( 'NONE', #9473, #9496 ) ;
#8273=ORIENTED_EDGE ( 'NONE', *, *, #12939, .T. ) ;
#8276=CARTESIAN_POINT ( 'NONE',  ( -71.24615306438093398, 66.54966845456371516, -15.00000000000001421 ) ) ;
#8281=CARTESIAN_POINT ( 'NONE',  ( -71.24615306438070661, 134.7758360152292312, -167.1454815528550739 ) ) ;
#8287=LINE ( 'NONE', #18296, #1194 ) ;
#8291=VERTEX_POINT ( 'NONE', #9759 ) ;
#8293=CARTESIAN_POINT ( 'NONE',  ( -68.99615306438093398, 71.12504998813029999, -15.00000000000001421 ) ) ;
#8295=ORIENTED_EDGE ( 'NONE', *, *, #3090, .F. ) ;
#8300=ORIENTED_EDGE ( 'NONE', *, *, #4266, .T. ) ;
#8301=DIRECTION ( 'NONE',  ( 0.000000000000000000, 1.000000000000000000, 0.000000000000000000 ) ) ;
#8302=DIRECTION ( 'NONE',  ( 0.000000000000000000, 1.000000000000000000, 0.000000000000000000 ) ) ;
#8307=DIRECTION ( 'NONE',  ( 1.000000000000000000, 0.000000000000000000, 0.000000000000000000 ) ) ;
#8308=DIRECTION ( 'NONE',  ( 0.000000000000000000, 0.000000000000000000, -1.000000000000000000 ) ) ;
#8309=DIRECTION ( 'NONE',  ( -0.9396926207859068736, 0.3420201433256726542, 1.086737899652988043E-16 ) ) ;
#8311=VERTEX_POINT ( 'NONE', #14392 ) ;
#8313=CARTESIAN_POINT ( 'NONE',  ( -71.24615306438084872, 101.1071876045637055, -15.00000000000001421 ) ) ;
#8314=EDGE_CURVE ( 'NONE', #8559, #794, #12277, .T. ) ;
#8323=CARTESIAN_POINT ( 'NONE',  ( -68.99615306438091977, 77.40823528813029952, 15.00000000000006928 ) ) ;
#8324=EDGE_LOOP ( 'NONE', ( #16142, #14046, #1455, #4664 ) ) ;
#8326=DIRECTION ( 'NONE',  ( 0.000000000000000000, 0.000000000000000000, 1.000000000000000000 ) ) ;
#8327=ORIENTED_EDGE ( 'NONE', *, *, #11685, .F. ) ;
#8333=ORIENTED_EDGE ( 'NONE', *, *, #2621, .F. ) ;
#8339=PLANE ( 'NONE',  #9357 ) ;
#8342=DIRECTION ( 'NONE',  ( 0.000000000000000000, 1.000000000000000000, 0.000000000000000000 ) ) ;
#8344=ORIENTED_EDGE ( 'NONE', *, *, #2054, .F. ) ;
#8345=VECTOR ( 'NONE', #1818, 1000.000000000000000 ) ;
#8347=LINE ( 'NONE', #8631, #15876 ) ;
#8348=ORIENTED_EDGE ( 'NONE', *, *, #17719, .F. ) ;
#8351=CARTESIAN_POINT ( 'NONE',  ( -68.99615306438083451, 99.39938383813029077, 15.00000000000006928 ) ) ;
#8358=EDGE_CURVE ( 'NONE', #2873, #11376, #9055, .T. ) ;
#8361=VECTOR ( 'NONE', #6943, 1000.000000000000000 ) ;
#8366=ORIENTED_EDGE ( 'NONE', *, *, #15471, .F. ) ;
#8371=ORIENTED_EDGE ( 'NONE', *, *, #6268, .F. ) ;
#8375=FACE_OUTER_BOUND ( 'NONE', #13627, .T. ) ;
#8376=EDGE_CURVE ( 'NONE', #13839, #14227, #7551, .T. ) ;
#8379=DIRECTION ( 'NONE',  ( 0.000000000000000000, 1.000000000000000000, 0.000000000000000000 ) ) ;
#8380=DIRECTION ( 'NONE',  ( 0.000000000000000000, 1.000000000000000000, 0.000000000000000000 ) ) ;
#8383=CARTESIAN_POINT ( 'NONE',  ( -68.99615306438100504, 39.09426763166271002, 15.00000000000006928 ) ) ;
#8385=ORIENTED_EDGE ( 'NONE', *, *, #5835, .T. ) ;
#8387=ADVANCED_FACE ( 'NONE', ( #8876 ), #17280, .T. ) ;
#8390=EDGE_CURVE ( 'NONE', #5168, #9316, #14743, .T. ) ;
#8392=EDGE_LOOP ( 'NONE', ( #14782, #15002, #9104, #743 ) ) ;
#8396=VECTOR ( 'NONE', #9437, 1000.000000000000000 ) ;
#8398=DIRECTION ( 'NONE',  ( 1.000000000000000000, 0.000000000000000000, 0.000000000000000000 ) ) ;
#8399=VERTEX_POINT ( 'NONE', #3428 ) ;
#8400=CARTESIAN_POINT ( 'NONE',  ( -71.24615306438082030, 97.96559495456375544, -15.00000000000001421 ) ) ;
#8401=FACE_OUTER_BOUND ( 'NONE', #12541, .T. ) ;
#8403=FACE_OUTER_BOUND ( 'NONE', #9265, .T. ) ;
#8406=DIRECTION ( 'NONE',  ( 1.000000000000000000, 0.000000000000000000, 0.000000000000000000 ) ) ;
#8407=CARTESIAN_POINT ( 'NONE',  ( -71.24615306438097662, 63.40807580456375803, -167.1454815528550739 ) ) ;
#8408=VECTOR ( 'NONE', #17098, 1000.000000000000000 ) ;
#8410=AXIS2_PLACEMENT_3D ( 'NONE', #10622, #6197, #11923 ) ;
#8423=DIRECTION ( 'NONE',  ( 0.000000000000000000, 0.000000000000000000, 1.000000000000000000 ) ) ;
#8426=VERTEX_POINT ( 'NONE', #8962 ) ;
#8435=VECTOR ( 'NONE', #16222, 1000.000000000000000 ) ;
#8438=PLANE ( 'NONE',  #8216 ) ;
#8439=DIRECTION ( 'NONE',  ( -0.9396926207859092051, 0.3420201433256663259, 0.000000000000000000 ) ) ;
#8441=VECTOR ( 'NONE', #11494, 1000.000000000000000 ) ;
#8444=ORIENTED_EDGE ( 'NONE', *, *, #5526, .F. ) ;
#8445=FACE_OUTER_BOUND ( 'NONE', #1545, .T. ) ;
#8446=ORIENTED_EDGE ( 'NONE', *, *, #16130, .F. ) ;
#8450=CARTESIAN_POINT ( 'NONE',  ( -68.99615306438094819, 70.51019413166270056, -167.1454815528550739 ) ) ;
#8455=AXIS2_PLACEMENT_3D ( 'NONE', #18099, #15475, #11277 ) ;
#8456=ORIENTED_EDGE ( 'NONE', *, *, #16606, .F. ) ;
#8457=ADVANCED_FACE ( 'NONE', ( #11767 ), #444, .T. ) ;
#8458=VECTOR ( 'NONE', #9837, 1000.000000000000114 ) ;
#8460=DIRECTION ( 'NONE',  ( 0.000000000000000000, 1.000000000000000000, 0.000000000000000000 ) ) ;
#8464=VERTEX_POINT ( 'NONE', #14657 ) ;
#8468=AXIS2_PLACEMENT_3D ( 'NONE', #17462, #4649, #10363 ) ;
#8474=PLANE ( 'NONE',  #11360 ) ;
#8478=VECTOR ( 'NONE', #8809, 1000.000000000000114 ) ;
#8479=VECTOR ( 'NONE', #5895, 1000.000000000000000 ) ;
#8483=CARTESIAN_POINT ( 'NONE',  ( -71.24615306438076345, 125.3510580652292248, -167.1454815528550739 ) ) ;
#8484=ORIENTED_EDGE ( 'NONE', *, *, #7873, .F. ) ;
#8487=EDGE_CURVE ( 'NONE', #13457, #8085, #2023, .T. ) ;
#8492=EDGE_CURVE ( 'NONE', #773, #16082, #5203, .T. ) ;
#8494=VECTOR ( 'NONE', #15493, 1000.000000000000000 ) ;
#8495=CARTESIAN_POINT ( 'NONE',  ( -68.99615306438091977, 73.65178678166269322, 15.00000000000006928 ) ) ;
#8496=CARTESIAN_POINT ( 'NONE',  ( -68.99615306438086293, 93.11619853813030545, 15.00000000000006928 ) ) ;
#8498=LINE ( 'NONE', #18497, #5772 ) ;
#8500=VERTEX_POINT ( 'NONE', #9507 ) ;
#8501=EDGE_CURVE ( 'NONE', #11612, #8311, #10818, .T. ) ;
#8502=LINE ( 'NONE', #2394, #14069 ) ;
#8505=DIRECTION ( 'NONE',  ( 0.3420201433256456203, 0.9396926207859168656, -0.000000000000000000 ) ) ;
#8506=EDGE_LOOP ( 'NONE', ( #3113, #13277, #2711, #5296 ) ) ;
#8508=CARTESIAN_POINT ( 'NONE',  ( -68.99615306438077766, 124.5321250381302747, -167.1454815528550739 ) ) ;
#8509=DIRECTION ( 'NONE',  ( 0.000000000000000000, 1.000000000000000000, 0.000000000000000000 ) ) ;
#8512=VECTOR ( 'NONE', #1555, 1000.000000000000000 ) ;
#8516=ORIENTED_EDGE ( 'NONE', *, *, #7436, .T. ) ;
#8528=CARTESIAN_POINT ( 'NONE',  ( -68.99615306438111872, 10.81993378166265529, -15.00000000000001421 ) ) ;
#8531=DIRECTION ( 'NONE',  ( 0.000000000000000000, 0.000000000000000000, 1.000000000000000000 ) ) ;
#8533=PLANE ( 'NONE',  #8983 ) ;
#8535=CARTESIAN_POINT ( 'NONE',  ( -71.24615306438073503, 128.4926507152292459, -167.1454815528550739 ) ) ;
#8538=ORIENTED_EDGE ( 'NONE', *, *, #8132, .T. ) ;
#8539=AXIS2_PLACEMENT_3D ( 'NONE', #4004, #15424, #6809 ) ;
#8540=VECTOR ( 'NONE', #5692, 1000.000000000000000 ) ;
#8542=ORIENTED_EDGE ( 'NONE', *, *, #7926, .F. ) ;
#8543=FACE_OUTER_BOUND ( 'NONE', #364, .T. ) ;
#8546=DIRECTION ( 'NONE',  ( 0.000000000000000000, 0.000000000000000000, 1.000000000000000000 ) ) ;
#8549=DIRECTION ( 'NONE',  ( 0.000000000000000000, 0.000000000000000000, 1.000000000000000000 ) ) ;
#8551=ADVANCED_FACE ( 'NONE', ( #1006 ), #6314, .T. ) ;
#8552=CARTESIAN_POINT ( 'NONE',  ( -71.24615306438067819, 145.0894847045637732, 15.00000000000006928 ) ) ;
#8555=LINE ( 'NONE', #18468, #13431 ) ;
#8558=ORIENTED_EDGE ( 'NONE', *, *, #226, .F. ) ;
#8559=VERTEX_POINT ( 'NONE', #16326 ) ;
#8564=PLANE ( 'NONE',  #3433 ) ;
#8569=VERTEX_POINT ( 'NONE', #16697 ) ;
#8571=ORIENTED_EDGE ( 'NONE', *, *, #1076, .F. ) ;
#8573=ORIENTED_EDGE ( 'NONE', *, *, #366, .T. ) ;
#8574=LINE ( 'NONE', #15404, #136 ) ;
#8575=ORIENTED_EDGE ( 'NONE', *, *, #18428, .T. ) ;
#8577=EDGE_CURVE ( 'NONE', #8399, #7810, #17743, .T. ) ;
#8581=PLANE ( 'NONE',  #17024 ) ;
#8582=LINE ( 'NONE', #14287, #4170 ) ;
#8583=CARTESIAN_POINT ( 'NONE',  ( -71.24615306438097662, 56.23601976522923707, -15.00000000000001421 ) ) ;
#8584=CARTESIAN_POINT ( 'NONE',  ( -68.99615306438120399, -1.746436818337276931, -167.1454815528550739 ) ) ;
#8585=ORIENTED_EDGE ( 'NONE', *, *, #11454, .F. ) ;
#8586=DIRECTION ( 'NONE',  ( 0.000000000000000000, 1.000000000000000000, 0.000000000000000000 ) ) ;
#8588=FACE_OUTER_BOUND ( 'NONE', #2649, .T. ) ;
#8593=CARTESIAN_POINT ( 'NONE',  ( -71.24615306438089135, 81.36876096522922808, -15.00000000000001421 ) ) ;
#8597=VERTEX_POINT ( 'NONE', #8583 ) ;
#8598=VERTEX_POINT ( 'NONE', #2685 ) ;
#8599=EDGE_CURVE ( 'NONE', #13376, #8923, #2789, .T. ) ;
#8600=EDGE_CURVE ( 'NONE', #5572, #16527, #8498, .T. ) ;
#8606=PLANE ( 'NONE',  #14464 ) ;
#8608=DIRECTION ( 'NONE',  ( 0.9396926207859084279, 0.3420201433256686574, 4.890320548438448905E-16 ) ) ;
#8609=CARTESIAN_POINT ( 'NONE',  ( -68.99615306438089135, 67.36860148166267948, -167.1454815528550739 ) ) ;
#8612=ORIENTED_EDGE ( 'NONE', *, *, #3795, .F. ) ;
#8613=DIRECTION ( 'NONE',  ( -0.9396926207859022107, 0.3420201433256853663, 1.086737899652982620E-16 ) ) ;
#8616=LINE ( 'NONE', #5527, #7478 ) ;
#8619=LINE ( 'NONE', #10109, #316 ) ;
#8620=ORIENTED_EDGE ( 'NONE', *, *, #18213, .F. ) ;
#8625=CARTESIAN_POINT ( 'NONE',  ( -71.24615306438087714, 82.25763170456374951, -15.00000000000001421 ) ) ;
#8626=EDGE_CURVE ( 'NONE', #409, #10136, #17087, .T. ) ;
#8628=CARTESIAN_POINT ( 'NONE',  ( -68.99615306438070661, 136.4836397816626743, -15.00000000000001421 ) ) ;
#8631=CARTESIAN_POINT ( 'NONE',  ( -68.99615306438103346, 33.42593818813029571, -167.1454815528550739 ) ) ;
#8639=EDGE_LOOP ( 'NONE', ( #7103, #15672, #824, #12774 ) ) ;
#8641=AXIS2_PLACEMENT_3D ( 'NONE', #13030, #17390, #5711 ) ;
#8647=CARTESIAN_POINT ( 'NONE',  ( -71.24615306438074924, 104.2487802545637692, 15.00000000000006928 ) ) ;
#8651=DIRECTION ( 'NONE',  ( 0.000000000000000000, 0.000000000000000000, -1.000000000000000000 ) ) ;
#8655=ADVANCED_FACE ( 'NONE', ( #18414 ), #11302, .T. ) ;
#8656=CARTESIAN_POINT ( 'NONE',  ( -68.99615306438111872, 11.43478963813029914, 15.00000000000006928 ) ) ;
#8659=ORIENTED_EDGE ( 'NONE', *, *, #10884, .T. ) ;
#8661=ORIENTED_EDGE ( 'NONE', *, *, #907, .F. ) ;
#8664=CARTESIAN_POINT ( 'NONE',  ( -71.24615306438089135, 81.36876096522922808, -167.1454815528550739 ) ) ;
#8666=DIRECTION ( 'NONE',  ( 0.000000000000000000, 1.000000000000000000, 0.000000000000000000 ) ) ;
#8670=DIRECTION ( 'NONE',  ( 0.000000000000000000, 1.000000000000000000, 0.000000000000000000 ) ) ;
#8671=CARTESIAN_POINT ( 'NONE',  ( -71.24615306438099083, 38.27533460456378123, 15.00000000000006928 ) ) ;
#8676=LINE ( 'NONE', #76, #15555 ) ;
#8682=DIRECTION ( 'NONE',  ( 1.000000000000000000, 0.000000000000000000, 0.000000000000000000 ) ) ;
#8683=ADVANCED_FACE ( 'NONE', ( #8204 ), #4279, .T. ) ;
#8686=PLANE ( 'NONE',  #11749 ) ;
#8687=DIRECTION ( 'NONE',  ( 0.3420201433256481738, -0.9396926207859158664, 0.000000000000000000 ) ) ;
#8688=DIRECTION ( 'NONE',  ( 0.000000000000000000, 1.000000000000000000, 0.000000000000000000 ) ) ;
#8689=ADVANCED_FACE ( 'NONE', ( #9706 ), #1193, .T. ) ;
#8691=( GEOMETRIC_REPRESENTATION_CONTEXT ( 3 ) GLOBAL_UNCERTAINTY_ASSIGNED_CONTEXT ( ( #13957 ) ) GLOBAL_UNIT_ASSIGNED_CONTEXT ( ( #368, #6330, #7839 ) ) REPRESENTATION_CONTEXT ( 'NONE', 'WORKASPACE' ) );
#8692=LINE ( 'NONE', #13178, #10754 ) ;
#8693=PLANE ( 'NONE',  #1658 ) ;
#8699=VECTOR ( 'NONE', #3896, 1000.000000000000227 ) ;
#8702=EDGE_CURVE ( 'NONE', #13724, #2315, #10426, .T. ) ;
#8707=EDGE_LOOP ( 'NONE', ( #16599, #8385, #135, #1684 ) ) ;
#8708=VERTEX_POINT ( 'NONE', #8939 ) ;
#8710=EDGE_CURVE ( 'NONE', #2059, #2407, #1917, .T. ) ;
#8712=EDGE_CURVE ( 'NONE', #15993, #8797, #3225, .T. ) ;
#8714=EDGE_CURVE ( 'NONE', #5859, #9827, #16118, .T. ) ;
#8716=LINE ( 'NONE', #14418, #1637 ) ;
#8720=DIRECTION ( 'NONE',  ( 0.000000000000000000, 0.000000000000000000, 1.000000000000000000 ) ) ;
#8721=PLANE ( 'NONE',  #14674 ) ;
#8729=ORIENTED_EDGE ( 'NONE', *, *, #13086, .F. ) ;
#8734=ADVANCED_FACE ( 'NONE', ( #324 ), #423, .T. ) ;
#8739=LINE ( 'NONE', #3120, #422 ) ;
#8740=FACE_OUTER_BOUND ( 'NONE', #1088, .T. ) ;
#8741=VERTEX_POINT ( 'NONE', #10152 ) ;
#8743=AXIS2_PLACEMENT_3D ( 'NONE', #8968, #17470, #4655 ) ;
#8745=CARTESIAN_POINT ( 'NONE',  ( -93.54007869656273044, 187.7866419848965052, 15.00000000000006928 ) ) ;
#8749=ORIENTED_EDGE ( 'NONE', *, *, #5699, .F. ) ;
#8756=EDGE_LOOP ( 'NONE', ( #3966, #4250, #10711, #14692 ) ) ;
#8759=CARTESIAN_POINT ( 'NONE',  ( -71.24615306438111872, 19.42577870456376132, -15.00000000000001421 ) ) ;
#8760=VECTOR ( 'NONE', #17969, 1000.000000000000114 ) ;
#8761=ORIENTED_EDGE ( 'NONE', *, *, #1943, .T. ) ;
#8762=LINE ( 'NONE', #14465, #10738 ) ;
#8763=LINE ( 'NONE', #10425, #5042 ) ;
#8764=CARTESIAN_POINT ( 'NONE',  ( -68.99615306438111872, 7.678341131662685726, 15.00000000000006928 ) ) ;
#8766=ORIENTED_EDGE ( 'NONE', *, *, #1968, .T. ) ;
#8767=EDGE_CURVE ( 'NONE', #3371, #9665, #509, .T. ) ;
#8768=LINE ( 'NONE', #4534, #14086 ) ;
#8770=VECTOR ( 'NONE', #6850, 1000.000000000000000 ) ;
#8777=LINE ( 'NONE', #3235, #4743 ) ;
#8785=PLANE ( 'NONE',  #4599 ) ;
#8789=DIRECTION ( 'NONE',  ( 0.000000000000000000, 0.000000000000000000, -1.000000000000000000 ) ) ;
#8792=ORIENTED_EDGE ( 'NONE', *, *, #13221, .F. ) ;
#8796=FACE_OUTER_BOUND ( 'NONE', #8756, .T. ) ;
#8797=VERTEX_POINT ( 'NONE', #7264 ) ;
#8798=EDGE_CURVE ( 'NONE', #10024, #18464, #17342, .T. ) ;
#8800=DIRECTION ( 'NONE',  ( -0.004825104377941397994, -0.9999883591161159435, -2.511066551536017787E-18 ) ) ;
#8805=ORIENTED_EDGE ( 'NONE', *, *, #18102, .T. ) ;
#8809=DIRECTION ( 'NONE',  ( 0.9396926207859084279, 0.3420201433256686574, -1.086737899652989892E-16 ) ) ;
#8810=EDGE_CURVE ( 'NONE', #16126, #4629, #3148, .T. ) ;
#8815=ORIENTED_EDGE ( 'NONE', *, *, #11893, .T. ) ;
#8819=CARTESIAN_POINT ( 'NONE',  ( -71.24615306438109030, 28.85055665456373575, 15.00000000000006928 ) ) ;
#8820=VERTEX_POINT ( 'NONE', #1731 ) ;
#8822=EDGE_CURVE ( 'NONE', #2315, #14578, #7433, .T. ) ;
#8824=DIRECTION ( 'NONE',  ( 0.9396926207859069846, 0.3420201433256723766, 4.890320548438442003E-16 ) ) ;
#8829=ORIENTED_EDGE ( 'NONE', *, *, #7552, .T. ) ;
#8830=EDGE_CURVE ( 'NONE', #18243, #5195, #4800, .T. ) ;
#8831=LINE ( 'NONE', #5824, #5206 ) ;
#8833=DIRECTION ( 'NONE',  ( 0.000000000000000000, 1.000000000000000000, 0.000000000000000000 ) ) ;
#8834=DIRECTION ( 'NONE',  ( 0.000000000000000000, 1.000000000000000000, 0.000000000000000000 ) ) ;
#8836=ORIENTED_EDGE ( 'NONE', *, *, #18428, .F. ) ;
#8838=EDGE_CURVE ( 'NONE', #2538, #881, #3690, .T. ) ;
#8845=CARTESIAN_POINT ( 'NONE',  ( -71.24615306438089135, 84.51035361522924916, 15.00000000000006928 ) ) ;
#8846=DIRECTION ( 'NONE',  ( -0.9396926207859097602, 0.3420201433256649381, -4.890320548438455808E-16 ) ) ;
#8858=DIRECTION ( 'NONE',  ( 0.000000000000000000, 1.000000000000000000, 0.000000000000000000 ) ) ;
#8871=ORIENTED_EDGE ( 'NONE', *, *, #13499, .T. ) ;
#8873=EDGE_CURVE ( 'NONE', #10695, #6984, #6479, .T. ) ;
#8876=FACE_OUTER_BOUND ( 'NONE', #9169, .T. ) ;
#8877=DIRECTION ( 'NONE',  ( 0.3420201433256686574, -0.9396926207859084279, 0.000000000000000000 ) ) ;
#8880=CARTESIAN_POINT ( 'NONE',  ( -68.99615306438097662, 57.94382353166266597, -15.00000000000001421 ) ) ;
#8884=LINE ( 'NONE', #8970, #12575 ) ;
#8885=ORIENTED_EDGE ( 'NONE', *, *, #5048, .F. ) ;
#8886=CARTESIAN_POINT ( 'NONE',  ( -68.99615306438072082, 127.0588618316627105, -15.00000000000001421 ) ) ;
#8888=EDGE_LOOP ( 'NONE', ( #7822, #407, #3285, #13904 ) ) ;
#8889=EDGE_CURVE ( 'NONE', #689, #7503, #4900, .T. ) ;
#8890=EDGE_LOOP ( 'NONE', ( #11692, #4537, #16558, #16554 ) ) ;
#8891=EDGE_LOOP ( 'NONE', ( #13679, #9863, #2380, #11636 ) ) ;
#8893=LINE ( 'NONE', #16163, #6346 ) ;
#8895=DIRECTION ( 'NONE',  ( 0.9396926207859084279, 0.3420201433256686574, 0.000000000000000000 ) ) ;
#8896=EDGE_CURVE ( 'NONE', #14192, #15440, #4986, .T. ) ;
#8899=EDGE_LOOP ( 'NONE', ( #11476, #4923, #16594, #17102 ) ) ;
#8903=EDGE_LOOP ( 'NONE', ( #16683, #2654, #4193, #15832 ) ) ;
#8906=ORIENTED_EDGE ( 'NONE', *, *, #7187, .T. ) ;
#8908=EDGE_LOOP ( 'NONE', ( #4968, #5809, #12597, #5528 ) ) ;
#8909=CARTESIAN_POINT ( 'NONE',  ( -71.24615306438070661, 134.7758360152292312, -15.00000000000001421 ) ) ;
#8916=VECTOR ( 'NONE', #9203, 1000.000000000000000 ) ;
#8923=VERTEX_POINT ( 'NONE', #13417 ) ;
#8925=FACE_OUTER_BOUND ( 'NONE', #1909, .T. ) ;
#8926=EDGE_LOOP ( 'NONE', ( #8348, #12080, #17538, #4221 ) ) ;
#8928=EDGE_CURVE ( 'NONE', #10355, #5064, #10619, .T. ) ;
#8930=VECTOR ( 'NONE', #15533, 1000.000000000000000 ) ;
#8931=VERTEX_POINT ( 'NONE', #13612 ) ;
#8932=CARTESIAN_POINT ( 'NONE',  ( -71.24615306438103346, 44.55851990456372391, -15.00000000000001421 ) ) ;
#8936=EDGE_CURVE ( 'NONE', #14282, #13644, #8179, .T. ) ;
#8937=EDGE_CURVE ( 'NONE', #14417, #4127, #1366, .T. ) ;
#8939=CARTESIAN_POINT ( 'NONE',  ( -68.99615306438089135, 80.54982793813027797, -15.00000000000001421 ) ) ;
#8941=ORIENTED_EDGE ( 'NONE', *, *, #786, .F. ) ;
#8945=DIRECTION ( 'NONE',  ( -5.204170427930409450E-16, 0.000000000000000000, 1.000000000000000000 ) ) ;
#8950=CARTESIAN_POINT ( 'NONE',  ( -68.99615306438111872, 8.293196988130274505, -15.00000000000001421 ) ) ;
#8951=ORIENTED_EDGE ( 'NONE', *, *, #12248, .F. ) ;
#8952=EDGE_CURVE ( 'NONE', #17521, #7151, #12408, .T. ) ;
#8961=DIRECTION ( 'NONE',  ( 1.000000000000000000, 0.000000000000000000, 0.000000000000000000 ) ) ;
#8962=CARTESIAN_POINT ( 'NONE',  ( -68.99615306438083451, 102.5409764881302692, -15.00000000000001421 ) ) ;
#8963=PLANE ( 'NONE',  #2204 ) ;
#8965=CARTESIAN_POINT ( 'NONE',  ( -71.24615306438089135, 84.51035361522924916, 15.00000000000006928 ) ) ;
#8968=CARTESIAN_POINT ( 'NONE',  ( -68.99615306438106188, 35.95267498166268894, -167.1454815528550739 ) ) ;
#8970=CARTESIAN_POINT ( 'NONE',  ( -68.99615306438079188, 108.8241617881302545, -15.00000000000001421 ) ) ;
#8971=VECTOR ( 'NONE', #8059, 1000.000000000000000 ) ;
#8976=ORIENTED_EDGE ( 'NONE', *, *, #3658, .F. ) ;
#8978=ORIENTED_EDGE ( 'NONE', *, *, #15689, .F. ) ;
#8979=AXIS2_PLACEMENT_3D ( 'NONE', #10088, #18426, #2896 ) ;
#8982=LINE ( 'NONE', #10114, #991 ) ;
#8983=AXIS2_PLACEMENT_3D ( 'NONE', #4123, #14240, #4308 ) ;
#8985=CARTESIAN_POINT ( 'NONE',  ( -71.24615306438079188, 113.6735582045637045, -167.1454815528550739 ) ) ;
#8986=LINE ( 'NONE', #17394, #3888 ) ;
#8989=DIRECTION ( 'NONE',  ( 1.000000000000000000, 0.000000000000000000, 0.000000000000000000 ) ) ;
#8992=EDGE_CURVE ( 'NONE', #12749, #7713, #12588, .T. ) ;
#8994=LINE ( 'NONE', #1878, #12959 ) ;
#8995=LINE ( 'NONE', #4757, #16408 ) ;
#8996=VERTEX_POINT ( 'NONE', #9963 ) ;
#8999=PLANE ( 'NONE',  #13909 ) ;
#9002=VECTOR ( 'NONE', #4804, 1000.000000000000000 ) ;
#9003=VECTOR ( 'NONE', #10247, 1000.000000000000227 ) ;
#9007=DIRECTION ( 'NONE',  ( 0.000000000000000000, 0.000000000000000000, 1.000000000000000000 ) ) ;
#9014=VECTOR ( 'NONE', #12282, 1000.000000000000000 ) ;
#9015=VECTOR ( 'NONE', #2558, 1000.000000000000114 ) ;
#9016=ORIENTED_EDGE ( 'NONE', *, *, #17728, .F. ) ;
#9018=VERTEX_POINT ( 'NONE', #12690 ) ;
#9019=CARTESIAN_POINT ( 'NONE',  ( -71.24615306438072082, 113.6735582045637329, 15.00000000000006928 ) ) ;
#9020=VERTEX_POINT ( 'NONE', #15670 ) ;
#9022=EDGE_CURVE ( 'NONE', #1535, #17780, #4075, .T. ) ;
#9024=ORIENTED_EDGE ( 'NONE', *, *, #8702, .F. ) ;
#9027=DIRECTION ( 'NONE',  ( 0.9396926207859069846, 0.3420201433256723766, 0.000000000000000000 ) ) ;
#9032=LINE ( 'NONE', #10427, #10293 ) ;
#9035=VECTOR ( 'NONE', #12583, 1000.000000000000000 ) ;
#9036=FACE_OUTER_BOUND ( 'NONE', #16364, .T. ) ;
#9037=CARTESIAN_POINT ( 'NONE',  ( -68.99615306438067819, 146.5232735881302801, -167.1454815528550739 ) ) ;
#9039=ORIENTED_EDGE ( 'NONE', *, *, #13367, .F. ) ;
#9040=VECTOR ( 'NONE', #6561, 1000.000000000000000 ) ;
#9043=EDGE_CURVE ( 'NONE', #7186, #13900, #6174, .T. ) ;
#9045=EDGE_CURVE ( 'NONE', #18127, #14885, #494, .T. ) ;
#9055=LINE ( 'NONE', #16053, #12663 ) ;
#9059=DIRECTION ( 'NONE',  ( 0.000000000000000000, 1.000000000000000000, 0.000000000000000000 ) ) ;
#9060=ADVANCED_FACE ( 'NONE', ( #13397 ), #10775, .T. ) ;
#9065=VERTEX_POINT ( 'NONE', #3379 ) ;
#9070=CARTESIAN_POINT ( 'NONE',  ( -68.99615306438106188, 35.95267498166268894, 15.00000000000006928 ) ) ;
#9074=ORIENTED_EDGE ( 'NONE', *, *, #792, .F. ) ;
#9079=CARTESIAN_POINT ( 'NONE',  ( -68.99615306438094819, 52.27549408813023746, -167.1454815528550739 ) ) ;
#9080=DIRECTION ( 'NONE',  ( 0.000000000000000000, 1.000000000000000000, 0.000000000000000000 ) ) ;
#9088=FACE_OUTER_BOUND ( 'NONE', #1492, .T. ) ;
#9092=DIRECTION ( 'NONE',  ( 0.000000000000000000, 1.000000000000000000, 0.000000000000000000 ) ) ;
#9093=ORIENTED_EDGE ( 'NONE', *, *, #13392, .T. ) ;
#9094=VECTOR ( 'NONE', #10298, 1000.000000000000114 ) ;
#9102=VERTEX_POINT ( 'NONE', #5158 ) ;
#9104=ORIENTED_EDGE ( 'NONE', *, *, #3658, .T. ) ;
#9107=PLANE ( 'NONE',  #17368 ) ;
#9108=LINE ( 'NONE', #2265, #1890 ) ;
#9112=VECTOR ( 'NONE', #1339, 1000.000000000000000 ) ;
#9115=DIRECTION ( 'NONE',  ( 0.9396926207859084279, 0.3420201433256686574, 4.890320548438448905E-16 ) ) ;
#9116=ORIENTED_EDGE ( 'NONE', *, *, #15181, .T. ) ;
#9121=DIRECTION ( 'NONE',  ( 0.000000000000000000, 1.000000000000000000, 0.000000000000000000 ) ) ;
#9126=EDGE_CURVE ( 'NONE', #12063, #17707, #9194, .T. ) ;
#9131=ORIENTED_EDGE ( 'NONE', *, *, #5268, .F. ) ;
#9137=ADVANCED_FACE ( 'NONE', ( #13493 ), #16565, .T. ) ;
#9138=EDGE_CURVE ( 'NONE', #17987, #593, #16375, .T. ) ;
#9143=PRODUCT_CONTEXT ( 'NONE', #7760, 'mechanical' ) ;
#9146=FACE_OUTER_BOUND ( 'NONE', #3870, .T. ) ;
#9147=ORIENTED_EDGE ( 'NONE', *, *, #3525, .T. ) ;
#9151=PLANE ( 'NONE',  #10327 ) ;
#9157=CARTESIAN_POINT ( 'NONE',  ( -71.24615306438070661, 138.8062994045637311, -15.00000000000001421 ) ) ;
#9158=CARTESIAN_POINT ( 'NONE',  ( -68.99615306438111872, 10.81993378166265529, 15.00000000000006928 ) ) ;
#9160=DIRECTION ( 'NONE',  ( -0.9396926207859158664, 0.3420201433256481738, 0.000000000000000000 ) ) ;
#9166=ADVANCED_FACE ( 'NONE', ( #11060 ), #15365, .T. ) ;
#9167=EDGE_CURVE ( 'NONE', #12615, #10671, #18077, .T. ) ;
#9168=FACE_OUTER_BOUND ( 'NONE', #1295, .T. ) ;
#9169=EDGE_LOOP ( 'NONE', ( #5751, #4172, #4744, #7067 ) ) ;
#9173=ADVANCED_FACE ( 'NONE', ( #16747 ), #11264, .T. ) ;
#9174=EDGE_CURVE ( 'NONE', #6461, #1535, #6758, .T. ) ;
#9176=DIRECTION ( 'NONE',  ( 0.9396926207859110924, 0.3420201433256612189, -1.086737899652992973E-16 ) ) ;
#9179=CARTESIAN_POINT ( 'NONE',  ( -68.99615306438106188, 26.52789703166272162, -167.1454815528550739 ) ) ;
#9181=FACE_OUTER_BOUND ( 'NONE', #3015, .T. ) ;
#9186=EDGE_CURVE ( 'NONE', #9018, #11293, #12564, .T. ) ;
#9188=DIRECTION ( 'NONE',  ( 0.000000000000000000, 0.000000000000000000, 1.000000000000000000 ) ) ;
#9191=DIRECTION ( 'NONE',  ( 0.3420201433256724322, -0.9396926207859070956, 0.000000000000000000 ) ) ;
#9194=LINE ( 'NONE', #14884, #8110 ) ;
#9197=CARTESIAN_POINT ( 'NONE',  ( -71.24615306438120399, -0.3126479347707321610, -15.00000000000001421 ) ) ;
#9198=CARTESIAN_POINT ( 'NONE',  ( -68.99615306438120399, -1.131580961869733448, -167.1454815528550739 ) ) ;
#9199=CARTESIAN_POINT ( 'NONE',  ( -71.24615306438120399, -0.3126479347707321610, 15.00000000000006928 ) ) ;
#9201=DIRECTION ( 'NONE',  ( 0.000000000000000000, 0.000000000000000000, -1.000000000000000000 ) ) ;
#9203=DIRECTION ( 'NONE',  ( 0.000000000000000000, 0.000000000000000000, 1.000000000000000000 ) ) ;
#9205=ORIENTED_EDGE ( 'NONE', *, *, #2166, .T. ) ;
#9207=VECTOR ( 'NONE', #9295, 1000.000000000000000 ) ;
#9210=CARTESIAN_POINT ( 'NONE',  ( -68.99615306438080609, 105.0677132816627051, -15.00000000000001421 ) ) ;
#9213=DIRECTION ( 'NONE',  ( 0.000000000000000000, 0.000000000000000000, 1.000000000000000000 ) ) ;
#9214=EDGE_LOOP ( 'NONE', ( #2386, #3508, #2345, #17801 ) ) ;
#9215=FACE_OUTER_BOUND ( 'NONE', #9214, .T. ) ;
#9217=EDGE_CURVE ( 'NONE', #18436, #2297, #4137, .T. ) ;
#9219=PLANE ( 'NONE',  #13010 ) ;
#9221=DIRECTION ( 'NONE',  ( 0.000000000000000000, 0.000000000000000000, -1.000000000000000000 ) ) ;
#9227=DIRECTION ( 'NONE',  ( 0.000000000000000000, 1.000000000000000000, 0.000000000000000000 ) ) ;
#9233=CARTESIAN_POINT ( 'NONE',  ( -71.24615306438087714, 85.39922435456371375, -15.00000000000001421 ) ) ;
#9235=LINE ( 'NONE', #16249, #14126 ) ;
#9238=CARTESIAN_POINT ( 'NONE',  ( -68.99615306438094819, 51.66063823166267355, -15.00000000000001421 ) ) ;
#9242=CARTESIAN_POINT ( 'NONE',  ( -71.24615306438114715, 12.25372266522925457, 15.00000000000006928 ) ) ;
#9247=EDGE_CURVE ( 'NONE', #7512, #1261, #16854, .T. ) ;
#9248=VECTOR ( 'NONE', #7874, 1000.000000000000000 ) ;
#9252=DIRECTION ( 'NONE',  ( 0.000000000000000000, 0.000000000000000000, 1.000000000000000000 ) ) ;
#9253=PLANE ( 'NONE',  #15721 ) ;
#9254=DIRECTION ( 'NONE',  ( 0.000000000000000000, 0.000000000000000000, -1.000000000000000000 ) ) ;
#9258=EDGE_LOOP ( 'NONE', ( #7305, #18042, #12374, #8060 ) ) ;
#9260=EDGE_CURVE ( 'NONE', #9888, #3544, #11164, .T. ) ;
#9264=LINE ( 'NONE', #7400, #6875 ) ;
#9265=EDGE_LOOP ( 'NONE', ( #14340, #5702, #1335, #13912 ) ) ;
#9267=ORIENTED_EDGE ( 'NONE', *, *, #8896, .F. ) ;
#9269=ADVANCED_FACE ( 'NONE', ( #6072 ), #12942, .T. ) ;
#9270=EDGE_CURVE ( 'NONE', #103, #11183, #5891, .T. ) ;
#9271=VECTOR ( 'NONE', #13018, 1000.000000000000000 ) ;
#9274=VECTOR ( 'NONE', #13720, 1000.000000000000000 ) ;
#9277=DIRECTION ( 'NONE',  ( 0.000000000000000000, 0.000000000000000000, 1.000000000000000000 ) ) ;
#9280=EDGE_CURVE ( 'NONE', #11545, #4878, #3186, .T. ) ;
#9281=VERTEX_POINT ( 'NONE', #10301 ) ;
#9295=DIRECTION ( 'NONE',  ( 0.000000000000000000, 0.000000000000000000, 1.000000000000000000 ) ) ;
#9300=ORIENTED_EDGE ( 'NONE', *, *, #9, .T. ) ;
#9301=VECTOR ( 'NONE', #3206, 1000.000000000000000 ) ;
#9306=CARTESIAN_POINT ( 'NONE',  ( -71.24615306438103346, 46.81124181522922356, 15.00000000000006928 ) ) ;
#9310=ORIENTED_EDGE ( 'NONE', *, *, #18311, .T. ) ;
#9312=CARTESIAN_POINT ( 'NONE',  ( -68.99615306438083451, 101.9261206316626698, 15.00000000000006928 ) ) ;
#9316=VERTEX_POINT ( 'NONE', #17222 ) ;
#9321=DIRECTION ( 'NONE',  ( 0.3420201433256407353, -0.9396926207859186420, 0.000000000000000000 ) ) ;
#9323=CARTESIAN_POINT ( 'NONE',  ( -94.45685920050698314, -47.21335801510345220, 15.00000000000006928 ) ) ;
#9326=LINE ( 'NONE', #12521, #6376 ) ;
#9328=EDGE_CURVE ( 'NONE', #16319, #9465, #1775, .T. ) ;
#9330=VECTOR ( 'NONE', #10350, 1000.000000000000114 ) ;
#9334=ORIENTED_EDGE ( 'NONE', *, *, #6673, .T. ) ;
#9339=LINE ( 'NONE', #9521, #8396 ) ;
#9351=LINE ( 'NONE', #3540, #10459 ) ;
#9353=LINE ( 'NONE', #10384, #7233 ) ;
#9357=AXIS2_PLACEMENT_3D ( 'NONE', #14148, #18364, #18459 ) ;
#9368=VECTOR ( 'NONE', #7998, 1000.000000000000114 ) ;
#9369=CARTESIAN_POINT ( 'NONE',  ( -71.24615306438106188, 35.13374195456378146, -167.1454815528550739 ) ) ;
#9370=DIRECTION ( 'NONE',  ( 0.000000000000000000, 0.000000000000000000, 1.000000000000000000 ) ) ;
#9376=EDGE_CURVE ( 'NONE', #7034, #7430, #2923, .T. ) ;
#9380=ADVANCED_FACE ( 'NONE', ( #3011 ), #8721, .T. ) ;
#9382=ORIENTED_EDGE ( 'NONE', *, *, #10507, .T. ) ;
#9383=CARTESIAN_POINT ( 'NONE',  ( -71.24615306438074924, 107.3903729045637476, 15.00000000000006928 ) ) ;
#9384=ORIENTED_EDGE ( 'NONE', *, *, #7616, .T. ) ;
#9389=ORIENTED_EDGE ( 'NONE', *, *, #2073, .F. ) ;
#9394=EDGE_CURVE ( 'NONE', #4629, #17860, #6154, .T. ) ;
#9399=VECTOR ( 'NONE', #6430, 999.9999999999998863 ) ;
#9407=CARTESIAN_POINT ( 'NONE',  ( -71.24615306438080609, 106.5015021652292404, 15.00000000000006928 ) ) ;
#9409=ORIENTED_EDGE ( 'NONE', *, *, #13045, .F. ) ;
#9410=DIRECTION ( 'NONE',  ( 0.000000000000000000, 1.000000000000000000, 0.000000000000000000 ) ) ;
#9413=LINE ( 'NONE', #17816, #1361 ) ;
#9414=AXIS2_PLACEMENT_3D ( 'NONE', #5399, #8406, #4289 ) ;
#9416=VECTOR ( 'NONE', #13374, 1000.000000000000000 ) ;
#9419=EDGE_LOOP ( 'NONE', ( #8344, #6101, #7401, #13229 ) ) ;
#9422=DIRECTION ( 'NONE',  ( 0.000000000000000000, 0.000000000000000000, 1.000000000000000000 ) ) ;
#9426=DIRECTION ( 'NONE',  ( 0.000000000000000000, 0.000000000000000000, 1.000000000000000000 ) ) ;
#9431=VECTOR ( 'NONE', #11117, 1000.000000000000114 ) ;
#9434=CARTESIAN_POINT ( 'NONE',  ( -68.99615306438094819, 51.66063823166267355, -15.00000000000001421 ) ) ;
#9435=CARTESIAN_POINT ( 'NONE',  ( -68.99615306438083451, 99.39938383813029077, -167.1454815528550739 ) ) ;
#9437=DIRECTION ( 'NONE',  ( 0.000000000000000000, 0.000000000000000000, 1.000000000000000000 ) ) ;
#9445=DIRECTION ( 'NONE',  ( -0.9396926207859157554, 0.3420201433256481738, -4.890320548438487362E-16 ) ) ;
#9451=LINE ( 'NONE', #3466, #16821 ) ;
#9452=DIRECTION ( 'NONE',  ( 0.000000000000000000, 0.000000000000000000, 1.000000000000000000 ) ) ;
#9456=CARTESIAN_POINT ( 'NONE',  ( -71.24615306438097662, 56.23601976522923707, 15.00000000000006928 ) ) ;
#9463=CARTESIAN_POINT ( 'NONE',  ( -71.24615306438101925, 25.70896400456379283, 15.00000000000006928 ) ) ;
#9465=VERTEX_POINT ( 'NONE', #12254 ) ;
#9467=DIRECTION ( 'NONE',  ( -0.000000000000000000, 1.000000000000000000, -0.000000000000000000 ) ) ;
#9469=ORIENTED_EDGE ( 'NONE', *, *, #586, .T. ) ;
#9471=PLANE ( 'NONE',  #14631 ) ;
#9473=CARTESIAN_POINT ( 'NONE',  ( -68.99615306438086293, 89.97460588813027016, -167.1454815528550739 ) ) ;
#9475=ORIENTED_EDGE ( 'NONE', *, *, #15355, .T. ) ;
#9478=CARTESIAN_POINT ( 'NONE',  ( -71.24615306438117557, 5.970537365229261262, -167.1454815528550739 ) ) ;
#9483=ORIENTED_EDGE ( 'NONE', *, *, #7082, .T. ) ;
#9484=LINE ( 'NONE', #6482, #17938 ) ;
#9487=EDGE_CURVE ( 'NONE', #17232, #9825, #9353, .T. ) ;
#9492=EDGE_CURVE ( 'NONE', #8164, #6219, #653, .T. ) ;
#9494=FACE_OUTER_BOUND ( 'NONE', #8392, .T. ) ;
#9496=VECTOR ( 'NONE', #12573, 1000.000000000000000 ) ;
#9497=ADVANCED_FACE ( 'NONE', ( #4956 ), #10749, .T. ) ;
#9507=CARTESIAN_POINT ( 'NONE',  ( -68.99615306438106188, 24.00116023813026445, -15.00000000000001421 ) ) ;
#9509=ORIENTED_EDGE ( 'NONE', *, *, #4458, .T. ) ;
#9513=PLANE ( 'NONE',  #16486 ) ;
#9517=CARTESIAN_POINT ( 'NONE',  ( -71.24615306438091977, 75.97444640456376419, -167.1454815528550739 ) ) ;
#9521=CARTESIAN_POINT ( 'NONE',  ( -68.99615306438077766, 114.4924912316626688, -167.1454815528550739 ) ) ;
#9523=ORIENTED_EDGE ( 'NONE', *, *, #2535, .F. ) ;
#9524=ORIENTED_EDGE ( 'NONE', *, *, #7229, .F. ) ;
#9536=ORIENTED_EDGE ( 'NONE', *, *, #2732, .T. ) ;
#9538=CARTESIAN_POINT ( 'NONE',  ( -68.99615306438111872, 11.43478963813029914, -167.1454815528550739 ) ) ;
#9539=CARTESIAN_POINT ( 'NONE',  ( -71.24615306438097662, 63.40807580456375803, 15.00000000000006928 ) ) ;
#9540=VECTOR ( 'NONE', #108, 1000.000000000000114 ) ;
#9542=CARTESIAN_POINT ( 'NONE',  ( -68.99615306438070661, 133.9569029881302811, -15.00000000000001421 ) ) ;
#9549=LINE ( 'NONE', #6550, #15359 ) ;
#9551=CARTESIAN_POINT ( 'NONE',  ( -71.24615306438100504, 53.98329785456373742, -167.1454815528550739 ) ) ;
#9558=LINE ( 'NONE', #6665, #5767 ) ;
#9560=EDGE_CURVE ( 'NONE', #3211, #3179, #2428, .T. ) ;
#9562=DIRECTION ( 'NONE',  ( 0.3420201433256546686, -0.9396926207859135349, 0.000000000000000000 ) ) ;
#9563=ORIENTED_EDGE ( 'NONE', *, *, #7909, .F. ) ;
#9567=AXIS2_PLACEMENT_3D ( 'NONE', #15894, #17378, #10284 ) ;
#9570=DIRECTION ( 'NONE',  ( 0.9396926207859185309, 0.3420201433256406798, -1.086737899653001478E-16 ) ) ;
#9575=AXIS2_PLACEMENT_3D ( 'NONE', #18055, #8139, #844 ) ;
#9576=CARTESIAN_POINT ( 'NONE',  ( -71.24615306438080609, 103.3599095152292193, -167.1454815528550739 ) ) ;
#9579=CARTESIAN_POINT ( 'NONE',  ( -68.99615306438093398, 64.84186468813030046, -15.00000000000001421 ) ) ;
#9581=VECTOR ( 'NONE', #14013, 1000.000000000000114 ) ;
#9586=EDGE_CURVE ( 'NONE', #11230, #5649, #12456, .T. ) ;
#9587=CARTESIAN_POINT ( 'NONE',  ( -71.24615306438101925, 47.70011255456375210, -15.00000000000001421 ) ) ;
#9588=VECTOR ( 'NONE', #403, 1000.000000000000114 ) ;
#9589=DIRECTION ( 'NONE',  ( 0.000000000000000000, 1.000000000000000000, 0.000000000000000000 ) ) ;
#9593=EDGE_CURVE ( 'NONE', #10434, #13327, #5523, .T. ) ;
#9597=ORIENTED_EDGE ( 'NONE', *, *, #1721, .F. ) ;
#9604=LINE ( 'NONE', #12523, #17631 ) ;
#9606=LINE ( 'NONE', #15504, #2446 ) ;
#9608=EDGE_LOOP ( 'NONE', ( #5049, #12393, #18117, #7447 ) ) ;
#9610=EDGE_CURVE ( 'NONE', #6984, #425, #12357, .T. ) ;
#9613=DIRECTION ( 'NONE',  ( 0.3420201433256724322, 0.9396926207859070956, -0.000000000000000000 ) ) ;
#9628=PLANE ( 'NONE',  #4567 ) ;
#9629=EDGE_CURVE ( 'NONE', #15808, #103, #13848, .T. ) ;
#9630=DIRECTION ( 'NONE',  ( -0.9396926207858995461, 0.3420201433256928603, 1.086737899652979538E-16 ) ) ;
#9631=ORIENTED_EDGE ( 'NONE', *, *, #10945, .F. ) ;
#9639=LINE ( 'NONE', #16638, #4211 ) ;
#9642=PLANE ( 'NONE',  #17777 ) ;
#9645=ORIENTED_EDGE ( 'NONE', *, *, #795, .F. ) ;
#9650=CARTESIAN_POINT ( 'NONE',  ( -71.24615306438101925, 41.41692725456378810, -15.00000000000001421 ) ) ;
#9653=VECTOR ( 'NONE', #2420, 1000.000000000000000 ) ;
#9662=ORIENTED_EDGE ( 'NONE', *, *, #9560, .T. ) ;
#9663=LINE ( 'NONE', #2842, #4569 ) ;
#9664=DIRECTION ( 'NONE',  ( 0.000000000000000000, 0.000000000000000000, 1.000000000000000000 ) ) ;
#9665=VERTEX_POINT ( 'NONE', #8323 ) ;
#9666=VECTOR ( 'NONE', #3514, 1000.000000000000000 ) ;
#9671=VECTOR ( 'NONE', #10637, 1000.000000000000000 ) ;
#9674=DIRECTION ( 'NONE',  ( 0.000000000000000000, 1.000000000000000000, 0.000000000000000000 ) ) ;
#9676=VECTOR ( 'NONE', #57, 1000.000000000000000 ) ;
#9681=DIRECTION ( 'NONE',  ( 0.000000000000000000, 0.000000000000000000, -1.000000000000000000 ) ) ;
#9682=ORIENTED_EDGE ( 'NONE', *, *, #8992, .T. ) ;
#9684=DIRECTION ( 'NONE',  ( 1.000000000000000000, 0.000000000000000000, 0.000000000000000000 ) ) ;
#9686=VECTOR ( 'NONE', #9426, 1000.000000000000000 ) ;
#9688=VECTOR ( 'NONE', #15930, 1000.000000000000114 ) ;
#9690=LINE ( 'NONE', #5566, #3958 ) ;
#9699=VECTOR ( 'NONE', #15815, 1000.000000000000000 ) ;
#9701=CARTESIAN_POINT ( 'NONE',  ( -71.24615306438076345, 125.3510580652292248, -15.00000000000001421 ) ) ;
#9702=ORIENTED_EDGE ( 'NONE', *, *, #9487, .T. ) ;
#9706=FACE_OUTER_BOUND ( 'NONE', #8025, .T. ) ;
#9707=FACE_OUTER_BOUND ( 'NONE', #13787, .T. ) ;
#9708=ORIENTED_EDGE ( 'NONE', *, *, #4359, .F. ) ;
#9709=VECTOR ( 'NONE', #10894, 1000.000000000000000 ) ;
#9711=FACE_OUTER_BOUND ( 'NONE', #17656, .T. ) ;
#9714=ORIENTED_EDGE ( 'NONE', *, *, #14729, .F. ) ;
#9715=VECTOR ( 'NONE', #2201, 1000.000000000000000 ) ;
#9718=DIRECTION ( 'NONE',  ( 0.000000000000000000, 1.000000000000000000, 0.000000000000000000 ) ) ;
#9719=DIRECTION ( 'NONE',  ( 1.000000000000000000, 0.000000000000000000, 0.000000000000000000 ) ) ;
#9724=ORIENTED_EDGE ( 'NONE', *, *, #9328, .F. ) ;
#9726=CARTESIAN_POINT ( 'NONE',  ( -71.24615306438086293, 101.1071876045637055, -167.1454815528550739 ) ) ;
#9730=VECTOR ( 'NONE', #11859, 1000.000000000000114 ) ;
#9733=CARTESIAN_POINT ( 'NONE',  ( -71.24615306438079188, 112.7846874652292399, 15.00000000000006928 ) ) ;
#9734=ORIENTED_EDGE ( 'NONE', *, *, #8118, .F. ) ;
#9743=ORIENTED_EDGE ( 'NONE', *, *, #12747, .F. ) ;
#9744=ADVANCED_FACE ( 'NONE', ( #15802 ), #1581, .T. ) ;
#9746=VECTOR ( 'NONE', #5475, 1000.000000000000227 ) ;
#9747=DIRECTION ( 'NONE',  ( 0.9396926207859171987, 0.3420201433256444545, 0.000000000000000000 ) ) ;
#9751=VERTEX_POINT ( 'NONE', #17114 ) ;
#9753=EDGE_CURVE ( 'NONE', #16693, #13576, #12921, .T. ) ;
#9759=CARTESIAN_POINT ( 'NONE',  ( -68.99615306438091977, 76.79337943166271430, -15.00000000000001421 ) ) ;
#9760=CARTESIAN_POINT ( 'NONE',  ( -71.24615306438076345, 122.2094654152292037, -15.00000000000001421 ) ) ;
#9761=CARTESIAN_POINT ( 'NONE',  ( -68.99615306438099083, 49.13390143813028743, -15.00000000000001421 ) ) ;
#9764=EDGE_LOOP ( 'NONE', ( #462, #6473, #6700, #18122 ) ) ;
#9770=EDGE_CURVE ( 'NONE', #10136, #7810, #5787, .T. ) ;
#9772=DIRECTION ( 'NONE',  ( 0.3420201433256686574, 0.9396926207859084279, -0.000000000000000000 ) ) ;
#9782=ORIENTED_EDGE ( 'NONE', *, *, #7794, .T. ) ;
#9786=EDGE_CURVE ( 'NONE', #13041, #115, #15629, .T. ) ;
#9787=CARTESIAN_POINT ( 'NONE',  ( -71.24615306438080609, 116.8151508545637114, -167.1454815528550739 ) ) ;
#9789=VERTEX_POINT ( 'NONE', #4393 ) ;
#9794=CARTESIAN_POINT ( 'NONE',  ( -71.24615306438110451, 3.717815454563776711, 15.00000000000006928 ) ) ;
#9795=CARTESIAN_POINT ( 'NONE',  ( -71.24615306438086293, 91.68240965456375591, -167.1454815528550739 ) ) ;
#9797=CARTESIAN_POINT ( 'NONE',  ( -68.99615306438067819, 145.9084177316626949, -167.1454815528550739 ) ) ;
#9805=CARTESIAN_POINT ( 'NONE',  ( -68.99615306438106188, 26.52789703166272517, -15.00000000000001421 ) ) ;
#9806=VERTEX_POINT ( 'NONE', #11421 ) ;
#9808=LINE ( 'NONE', #17001, #17337 ) ;
#9812=VERTEX_POINT ( 'NONE', #17017 ) ;
#9814=ORIENTED_EDGE ( 'NONE', *, *, #4577, .T. ) ;
#9817=AXIS2_PLACEMENT_3D ( 'NONE', #5170, #11273, #18178 ) ;
#9820=EDGE_CURVE ( 'NONE', #1460, #13724, #4303, .T. ) ;
#9825=VERTEX_POINT ( 'NONE', #11520 ) ;
#9827=VERTEX_POINT ( 'NONE', #10020 ) ;
#9833=ORIENTED_EDGE ( 'NONE', *, *, #18165, .F. ) ;
#9837=DIRECTION ( 'NONE',  ( 0.9396926207859171987, 0.3420201433256444545, -1.086737899652999999E-16 ) ) ;
#9838=EDGE_CURVE ( 'NONE', #10339, #2433, #13798, .T. ) ;
#9839=DIRECTION ( 'NONE',  ( 1.000000000000000000, 0.000000000000000000, 0.000000000000000000 ) ) ;
#9841=CARTESIAN_POINT ( 'NONE',  ( -68.99615306438100504, 42.23586028166270978, -167.1454815528550739 ) ) ;
#9843=VERTEX_POINT ( 'NONE', #12413 ) ;
#9846=ORIENTED_EDGE ( 'NONE', *, *, #15795, .T. ) ;
#9848=DIRECTION ( 'NONE',  ( 0.000000000000000000, 1.000000000000000000, 0.000000000000000000 ) ) ;
#9850=ADVANCED_FACE ( 'NONE', ( #10452 ), #13447, .T. ) ;
#9853=CARTESIAN_POINT ( 'NONE',  ( -68.99615306438093398, 49.13390143813026611, 15.00000000000006928 ) ) ;
#9859=VECTOR ( 'NONE', #5926, 1000.000000000000000 ) ;
#9861=DIRECTION ( 'NONE',  ( 1.000000000000000000, 0.000000000000000000, 0.000000000000000000 ) ) ;
#9862=DIRECTION ( 'NONE',  ( 1.000000000000000000, 0.000000000000000000, 0.000000000000000000 ) ) ;
#9863=ORIENTED_EDGE ( 'NONE', *, *, #18187, .T. ) ;
#9867=EDGE_CURVE ( 'NONE', #2737, #15821, #14662, .T. ) ;
#9868=CARTESIAN_POINT ( 'NONE',  ( -68.99615306438067819, 143.3816809381303585, 15.00000000000006928 ) ) ;
#9869=ORIENTED_EDGE ( 'NONE', *, *, #8066, .F. ) ;
#9874=DIRECTION ( 'NONE',  ( -0.9396926207859158664, 0.3420201433256481738, 1.086737899652998397E-16 ) ) ;
#9876=ORIENTED_EDGE ( 'NONE', *, *, #5526, .T. ) ;
#9879=DIRECTION ( 'NONE',  ( 1.000000000000000000, 0.000000000000000000, 0.000000000000000000 ) ) ;
#9883=ORIENTED_EDGE ( 'NONE', *, *, #8937, .F. ) ;
#9888=VERTEX_POINT ( 'NONE', #16677 ) ;
#9889=VECTOR ( 'NONE', #15605, 1000.000000000000227 ) ;
#9892=VECTOR ( 'NONE', #16604, 1000.000000000000000 ) ;
#9896=LINE ( 'NONE', #2689, #9889 ) ;
#9898=CARTESIAN_POINT ( 'NONE',  ( -71.24615306438067819, 144.2006139652292518, -167.1454815528550739 ) ) ;
#9899=CARTESIAN_POINT ( 'NONE',  ( -68.99615306438100504, 49.13390143813029454, -167.1454815528550739 ) ) ;
#9900=ORIENTED_EDGE ( 'NONE', *, *, #10884, .F. ) ;
#9902=PLANE ( 'NONE',  #8539 ) ;
#9905=AXIS2_PLACEMENT_3D ( 'NONE', #2368, #13902, #6784 ) ;
#9910=CARTESIAN_POINT ( 'NONE',  ( -68.99615306438067819, 145.9084177316626949, 15.00000000000006928 ) ) ;
#9913=ORIENTED_EDGE ( 'NONE', *, *, #14054, .F. ) ;
#9914=CARTESIAN_POINT ( 'NONE',  ( -71.24615306438086293, 91.68240965456375591, -15.00000000000001421 ) ) ;
#9915=CARTESIAN_POINT ( 'NONE',  ( -68.99615306438066398, 127.6737176881302673, 15.00000000000006928 ) ) ;
#9921=CARTESIAN_POINT ( 'NONE',  ( -71.24615306438091977, 72.83285375456371469, -167.1454815528550739 ) ) ;
#9925=CARTESIAN_POINT ( 'NONE',  ( -71.24615306438103346, 44.55851990456372391, -167.1454815528550739 ) ) ;
#9928=PLANE ( 'NONE',  #2718 ) ;
#9930=ORIENTED_EDGE ( 'NONE', *, *, #17937, .T. ) ;
#9936=CARTESIAN_POINT ( 'NONE',  ( -71.24615306438093398, 53.98329785456376584, 15.00000000000006928 ) ) ;
#9938=ADVANCED_FACE ( 'NONE', ( #4732 ), #14750, .T. ) ;
#9941=ORIENTED_EDGE ( 'NONE', *, *, #13067, .F. ) ;
#9942=LINE ( 'NONE', #15654, #3039 ) ;
#9943=ORIENTED_EDGE ( 'NONE', *, *, #13854, .F. ) ;
#9944=PLANE ( 'NONE',  #11162 ) ;
#9951=EDGE_CURVE ( 'NONE', #663, #8598, #1949, .T. ) ;
#9958=DIRECTION ( 'NONE',  ( 0.000000000000000000, 1.000000000000000000, 0.000000000000000000 ) ) ;
#9963=CARTESIAN_POINT ( 'NONE',  ( -71.24615306438094819, 68.80239036522922902, 15.00000000000006928 ) ) ;
#9967=CARTESIAN_POINT ( 'NONE',  ( -71.24615306438109030, 27.96168591522921076, 15.00000000000006928 ) ) ;
#9969=DIRECTION ( 'NONE',  ( 0.000000000000000000, 0.000000000000000000, -1.000000000000000000 ) ) ;
#9970=VERTEX_POINT ( 'NONE', #1177 ) ;
#9971=DIRECTION ( 'NONE',  ( -0.9396926207859097602, 0.3420201433256649381, -4.890320548438455808E-16 ) ) ;
#9977=EDGE_CURVE ( 'NONE', #1662, #7503, #5652, .T. ) ;
#9980=ADVANCED_FACE ( 'NONE', ( #10058 ), #2864, .T. ) ;
#9985=ADVANCED_FACE ( 'NONE', ( #5563 ), #1268, .T. ) ;
#9988=VECTOR ( 'NONE', #15696, 1000.000000000000000 ) ;
#9990=DIRECTION ( 'NONE',  ( 0.3420201433256481738, -0.9396926207859158664, 0.000000000000000000 ) ) ;
#9991=VECTOR ( 'NONE', #9674, 1000.000000000000000 ) ;
#9993=PLANE ( 'NONE',  #1617 ) ;
#9997=DIRECTION ( 'NONE',  ( 0.9396926207859110924, 0.3420201433256612189, -1.086737899652992973E-16 ) ) ;
#9998=ORIENTED_EDGE ( 'NONE', *, *, #11126, .T. ) ;
#10000=CARTESIAN_POINT ( 'NONE',  ( -68.99615306438097662, 61.08541618166268705, -167.1454815528550739 ) ) ;
#10003=CARTESIAN_POINT ( 'NONE',  ( -68.99615306438070661, 137.0984956381303164, -15.00000000000001421 ) ) ;
#10009=VECTOR ( 'NONE', #3043, 1000.000000000000000 ) ;
#10013=CARTESIAN_POINT ( 'NONE',  ( -68.99615306438103346, 32.81108233166271759, 15.00000000000006928 ) ) ;
#10014=ORIENTED_EDGE ( 'NONE', *, *, #2516, .T. ) ;
#10020=CARTESIAN_POINT ( 'NONE',  ( -71.24615306438079188, 112.7846874652292399, -15.00000000000001421 ) ) ;
#10021=ORIENTED_EDGE ( 'NONE', *, *, #10334, .F. ) ;
#10022=CARTESIAN_POINT ( 'NONE',  ( -68.99615306438091977, 73.65178678166269322, -167.1454815528550739 ) ) ;
#10023=LINE ( 'NONE', #15731, #8074 ) ;
#10024=VERTEX_POINT ( 'NONE', #43 ) ;
#10025=CARTESIAN_POINT ( 'NONE',  ( -71.24615306438086293, 90.79353891522923448, -15.00000000000001421 ) ) ;
#10026=LINE ( 'NONE', #1333, #5329 ) ;
#10027=ORIENTED_EDGE ( 'NONE', *, *, #14855, .F. ) ;
#10028=ORIENTED_EDGE ( 'NONE', *, *, #699, .T. ) ;
#10029=VECTOR ( 'NONE', #483, 1000.000000000000000 ) ;
#10034=CARTESIAN_POINT ( 'NONE',  ( -71.24615306438080609, 109.6430948152292189, -167.1454815528550739 ) ) ;
#10036=ORIENTED_EDGE ( 'NONE', *, *, #13051, .F. ) ;
#10041=AXIS2_PLACEMENT_3D ( 'NONE', #15213, #2396, #5210 ) ;
#10042=VECTOR ( 'NONE', #14704, 1000.000000000000000 ) ;
#10044=ORIENTED_EDGE ( 'NONE', *, *, #8599, .F. ) ;
#10047=ORIENTED_EDGE ( 'NONE', *, *, #4576, .F. ) ;
#10049=PLANE ( 'NONE',  #6378 ) ;
#10050=DIRECTION ( 'NONE',  ( 0.000000000000000000, 1.000000000000000000, 0.000000000000000000 ) ) ;
#10051=ORIENTED_EDGE ( 'NONE', *, *, #16225, .F. ) ;
#10056=FACE_OUTER_BOUND ( 'NONE', #15029, .T. ) ;
#10058=FACE_OUTER_BOUND ( 'NONE', #11422, .T. ) ;
#10062=ORIENTED_EDGE ( 'NONE', *, *, #10065, .F. ) ;
#10065=EDGE_CURVE ( 'NONE', #1178, #7613, #1371, .T. ) ;
#10066=ORIENTED_EDGE ( 'NONE', *, *, #3641, .T. ) ;
#10067=CARTESIAN_POINT ( 'NONE',  ( -71.24615306438074924, 132.5231141045637457, -15.00000000000001421 ) ) ;
#10069=DIRECTION ( 'NONE',  ( 0.000000000000000000, 1.000000000000000000, 0.000000000000000000 ) ) ;
#10070=ORIENTED_EDGE ( 'NONE', *, *, #7794, .F. ) ;
#10072=PLANE ( 'NONE',  #5949 ) ;
#10078=EDGE_CURVE ( 'NONE', #14184, #115, #1094, .T. ) ;
#10079=CARTESIAN_POINT ( 'NONE',  ( -71.24615306438109030, 25.70896400456376796, -167.1454815528550739 ) ) ;
#10082=EDGE_LOOP ( 'NONE', ( #11093, #18038, #3971, #9631 ) ) ;
#10088=CARTESIAN_POINT ( 'NONE',  ( -68.99615306438106188, 24.00116023813026445, -167.1454815528550739 ) ) ;
#10090=ORIENTED_EDGE ( 'NONE', *, *, #7684, .T. ) ;
#10091=ADVANCED_FACE ( 'NONE', ( #8375 ), #6972, .T. ) ;
#10100=EDGE_CURVE ( 'NONE', #3118, #17521, #6179, .T. ) ;
#10103=ORIENTED_EDGE ( 'NONE', *, *, #14221, .F. ) ;
#10106=CARTESIAN_POINT ( 'NONE',  ( -68.99615306438094819, 54.80223088166269463, -167.1454815528550739 ) ) ;
#10109=CARTESIAN_POINT ( 'NONE',  ( -71.24615306438086293, 87.65194626522927024, -167.1454815528550739 ) ) ;
#10112=VECTOR ( 'NONE', #7008, 1000.000000000000000 ) ;
#10113=CARTESIAN_POINT ( 'NONE',  ( -68.99615306438096241, 61.70027203813027938, -15.00000000000001421 ) ) ;
#10114=CARTESIAN_POINT ( 'NONE',  ( -71.24615306438086293, 101.1071876045637055, -167.1454815528550739 ) ) ;
#10116=LINE ( 'NONE', #10205, #14916 ) ;
#10117=DIRECTION ( 'NONE',  ( 0.000000000000000000, 1.000000000000000000, 0.000000000000000000 ) ) ;
#10120=ORIENTED_EDGE ( 'NONE', *, *, #10626, .T. ) ;
#10121=LINE ( 'NONE', #16079, #15018 ) ;
#10133=ORIENTED_EDGE ( 'NONE', *, *, #12225, .T. ) ;
#10136=VERTEX_POINT ( 'NONE', #3290 ) ;
#10137=FACE_OUTER_BOUND ( 'NONE', #9608, .T. ) ;
#10139=LINE ( 'NONE', #10410, #10838 ) ;
#10142=ORIENTED_EDGE ( 'NONE', *, *, #4582, .T. ) ;
#10143=ORIENTED_EDGE ( 'NONE', *, *, #14068, .T. ) ;
#10144=VECTOR ( 'NONE', #8858, 1000.000000000000000 ) ;
#10146=ORIENTED_EDGE ( 'NONE', *, *, #137, .F. ) ;
#10147=CARTESIAN_POINT ( 'NONE',  ( -68.99615306438091977, 73.65178678166269322, -15.00000000000001421 ) ) ;
#10151=LINE ( 'NONE', #15859, #17898 ) ;
#10152=CARTESIAN_POINT ( 'NONE',  ( -71.24615306438097662, 63.40807580456375803, -15.00000000000001421 ) ) ;
#10154=DIRECTION ( 'NONE',  ( -0.9396926207859088720, 0.3420201433256675472, 1.086737899652990385E-16 ) ) ;
#10155=EDGE_LOOP ( 'NONE', ( #5324, #2901, #18268, #17624 ) ) ;
#10159=PLANE ( 'NONE',  #18299 ) ;
#10161=VERTEX_POINT ( 'NONE', #142 ) ;
#10162=CARTESIAN_POINT ( 'NONE',  ( -71.24615306438114715, 9.112130015229229940, 15.00000000000006928 ) ) ;
#10166=EDGE_CURVE ( 'NONE', #10924, #3445, #10139, .T. ) ;
#10173=DIRECTION ( 'NONE',  ( 0.3420201433256649937, 0.9396926207859097602, -0.000000000000000000 ) ) ;
#10180=CARTESIAN_POINT ( 'NONE',  ( -71.24615306438097662, 56.23601976522923707, -167.1454815528550739 ) ) ;
#10181=DIRECTION ( 'NONE',  ( 1.000000000000000000, 0.000000000000000000, 0.000000000000000000 ) ) ;
#10184=ORIENTED_EDGE ( 'NONE', *, *, #4315, .F. ) ;
#10185=AXIS2_PLACEMENT_3D ( 'NONE', #9435, #6516, #12232 ) ;
#10192=CARTESIAN_POINT ( 'NONE',  ( -71.24615306438103346, 43.66964916522919538, -167.1454815528550739 ) ) ;
#10195=ORIENTED_EDGE ( 'NONE', *, *, #14773, .F. ) ;
#10196=EDGE_CURVE ( 'NONE', #11754, #15862, #5913, .T. ) ;
#10197=EDGE_CURVE ( 'NONE', #6984, #15061, #13322, .T. ) ;
#10203=CARTESIAN_POINT ( 'NONE',  ( -68.99615306438103346, 32.81108233166271759, -15.00000000000001421 ) ) ;
#10205=CARTESIAN_POINT ( 'NONE',  ( -71.24615306438073503, 129.3815214545637104, -167.1454815528550739 ) ) ;
#10206=DIRECTION ( 'NONE',  ( -0.9396926207859084279, 0.3420201433256686574, -4.890320548438448905E-16 ) ) ;
#10207=VERTEX_POINT ( 'NONE', #7345 ) ;
#10208=CARTESIAN_POINT ( 'NONE',  ( -68.99615306438111872, 20.85956758813031797, -15.00000000000001421 ) ) ;
#10210=DIRECTION ( 'NONE',  ( 0.9396926207859158664, 0.3420201433256481738, -1.086737899652998397E-16 ) ) ;
#10212=ORIENTED_EDGE ( 'NONE', *, *, #9838, .T. ) ;
#10214=DIRECTION ( 'NONE',  ( 0.000000000000000000, 0.000000000000000000, -1.000000000000000000 ) ) ;
#10218=ORIENTED_EDGE ( 'NONE', *, *, #7560, .T. ) ;
#10220=VECTOR ( 'NONE', #245, 1000.000000000000000 ) ;
#10222=LINE ( 'NONE', #14346, #5802 ) ;
#10223=LINE ( 'NONE', #33, #11145 ) ;
#10225=VECTOR ( 'NONE', #9997, 1000.000000000000000 ) ;
#10230=CARTESIAN_POINT ( 'NONE',  ( -71.24615306438091977, 71.94398301522919326, -15.00000000000001421 ) ) ;
#10231=CARTESIAN_POINT ( 'NONE',  ( -68.99615306438093398, 45.99230878813023793, 15.00000000000006928 ) ) ;
#10233=CARTESIAN_POINT ( 'NONE',  ( -68.99615306438067819, 145.9084177316626949, -167.1454815528550739 ) ) ;
#10242=DIRECTION ( 'NONE',  ( 0.000000000000000000, 1.000000000000000000, 0.000000000000000000 ) ) ;
#10245=CARTESIAN_POINT ( 'NONE',  ( -71.24615306438076345, 122.2094654152292037, -15.00000000000001421 ) ) ;
#10247=DIRECTION ( 'NONE',  ( 0.9396926207859157554, 0.3420201433256481738, 4.890320548438487362E-16 ) ) ;
#10248=LINE ( 'NONE', #13077, #15965 ) ;
#10254=DIRECTION ( 'NONE',  ( 0.000000000000000000, 0.000000000000000000, 1.000000000000000000 ) ) ;
#10256=EDGE_CURVE ( 'NONE', #12606, #9020, #17327, .T. ) ;
#10257=VERTEX_POINT ( 'NONE', #4612 ) ;
#10271=LINE ( 'NONE', #3244, #7886 ) ;
#10272=ORIENTED_EDGE ( 'NONE', *, *, #8376, .T. ) ;
#10275=CARTESIAN_POINT ( 'NONE',  ( -68.99615306438111872, 7.678341131662687502, -15.00000000000001421 ) ) ;
#10284=DIRECTION ( 'NONE',  ( -0.9396926207859084279, 0.3420201433256689905, 0.000000000000000000 ) ) ;
#10289=EDGE_CURVE ( 'NONE', #17556, #3227, #10495, .T. ) ;
#10293=VECTOR ( 'NONE', #1821, 1000.000000000000000 ) ;
#10296=DIRECTION ( 'NONE',  ( 0.000000000000000000, 1.000000000000000000, 0.000000000000000000 ) ) ;
#10298=DIRECTION ( 'NONE',  ( -0.9396926207859069846, 0.3420201433256723766, -4.890320548438442003E-16 ) ) ;
#10301=CARTESIAN_POINT ( 'NONE',  ( -68.99615306438077766, 117.6340838816626899, 15.00000000000006928 ) ) ;
#10303=EDGE_CURVE ( 'NONE', #12950, #6650, #17978, .T. ) ;
#10304=EDGE_CURVE ( 'NONE', #4587, #10505, #5063, .T. ) ;
#10305=VECTOR ( 'NONE', #12177, 999.9999999999998863 ) ;
#10306=FACE_OUTER_BOUND ( 'NONE', #2871, .T. ) ;
#10309=FACE_OUTER_BOUND ( 'NONE', #11017, .T. ) ;
#10310=VERTEX_POINT ( 'NONE', #16381 ) ;
#10311=VECTOR ( 'NONE', #4189, 1000.000000000000000 ) ;
#10314=LINE ( 'NONE', #1435, #15168 ) ;
#10319=EDGE_CURVE ( 'NONE', #7713, #10372, #15079, .T. ) ;
#10321=DIRECTION ( 'NONE',  ( 0.000000000000000000, 1.000000000000000000, 0.000000000000000000 ) ) ;
#10323=CARTESIAN_POINT ( 'NONE',  ( -68.99615306438089135, 83.69142058813029905, -167.1454815528550739 ) ) ;
#10324=VECTOR ( 'NONE', #1182, 1000.000000000000000 ) ;
#10325=ORIENTED_EDGE ( 'NONE', *, *, #17540, .T. ) ;
#10327=AXIS2_PLACEMENT_3D ( 'NONE', #7649, #4730, #10450 ) ;
#10328=ORIENTED_EDGE ( 'NONE', *, *, #14943, .T. ) ;
#10329=LINE ( 'NONE', #1709, #9588 ) ;
#10333=ORIENTED_EDGE ( 'NONE', *, *, #9138, .T. ) ;
#10334=EDGE_CURVE ( 'NONE', #16663, #9751, #17695, .T. ) ;
#10336=DIRECTION ( 'NONE',  ( 0.000000000000000000, 0.000000000000000000, 1.000000000000000000 ) ) ;
#10337=ORIENTED_EDGE ( 'NONE', *, *, #8100, .T. ) ;
#10339=VERTEX_POINT ( 'NONE', #12677 ) ;
#10344=LINE ( 'NONE', #17526, #13412 ) ;
#10348=LINE ( 'NONE', #15957, #14381 ) ;
#10350=DIRECTION ( 'NONE',  ( 0.9396926207859110924, 0.3420201433256612189, 4.890320548438462711E-16 ) ) ;
#10352=DIRECTION ( 'NONE',  ( 0.000000000000000000, 1.000000000000000000, 0.000000000000000000 ) ) ;
#10354=VERTEX_POINT ( 'NONE', #15267 ) ;
#10355=VERTEX_POINT ( 'NONE', #5262 ) ;
#10356=EDGE_LOOP ( 'NONE', ( #5552, #3295, #10090, #8446 ) ) ;
#10358=EDGE_CURVE ( 'NONE', #17780, #8931, #4061, .T. ) ;
#10363=DIRECTION ( 'NONE',  ( 0.000000000000000000, 0.000000000000000000, -1.000000000000000000 ) ) ;
#10372=VERTEX_POINT ( 'NONE', #11351 ) ;
#10380=LINE ( 'NONE', #3263, #1480 ) ;
#10381=DIRECTION ( 'NONE',  ( 0.9396926207859084279, 0.3420201433256686574, -1.086737899652989892E-16 ) ) ;
#10383=CARTESIAN_POINT ( 'NONE',  ( -68.99615306438072082, 127.6737176881302958, -167.1454815528550739 ) ) ;
#10384=CARTESIAN_POINT ( 'NONE',  ( -68.99615306438094819, 64.84186468813030046, -167.1454815528550739 ) ) ;
#10385=ORIENTED_EDGE ( 'NONE', *, *, #7552, .F. ) ;
#10390=CARTESIAN_POINT ( 'NONE',  ( -71.24615306438080609, 103.3599095152292193, 15.00000000000006928 ) ) ;
#10393=LINE ( 'NONE', #13212, #5919 ) ;
#10395=VECTOR ( 'NONE', #9188, 1000.000000000000000 ) ;
#10400=LINE ( 'NONE', #17684, #4888 ) ;
#10401=CARTESIAN_POINT ( 'NONE',  ( -68.99615306438100504, 39.70912348813028103, -167.1454815528550739 ) ) ;
#10402=ORIENTED_EDGE ( 'NONE', *, *, #6767, .T. ) ;
#10403=EDGE_LOOP ( 'NONE', ( #12778, #16656, #10599, #17802 ) ) ;
#10405=EDGE_CURVE ( 'NONE', #18141, #18474, #9663, .T. ) ;
#10406=CARTESIAN_POINT ( 'NONE',  ( -71.24615306438097662, 59.37761241522920841, -167.1454815528550739 ) ) ;
#10410=CARTESIAN_POINT ( 'NONE',  ( -71.24615306438076345, 125.3510580652292248, -15.00000000000001421 ) ) ;
#10420=EDGE_CURVE ( 'NONE', #1022, #8464, #1432, .T. ) ;
#10421=CARTESIAN_POINT ( 'NONE',  ( -68.99615306438096241, 33.42593818813026729, 15.00000000000006928 ) ) ;
#10422=ADVANCED_FACE ( 'NONE', ( #16956 ), #9944, .T. ) ;
#10425=CARTESIAN_POINT ( 'NONE',  ( -71.24615306438069240, 135.6647067545637242, -15.00000000000001421 ) ) ;
#10426=LINE ( 'NONE', #8764, #10796 ) ;
#10427=CARTESIAN_POINT ( 'NONE',  ( -71.24615306438103346, 44.55851990456372391, -167.1454815528550739 ) ) ;
#10428=VERTEX_POINT ( 'NONE', #10975 ) ;
#10433=DIRECTION ( 'NONE',  ( 0.000000000000000000, 0.000000000000000000, 1.000000000000000000 ) ) ;
#10434=VERTEX_POINT ( 'NONE', #11168 ) ;
#10436=DIRECTION ( 'NONE',  ( 0.000000000000000000, 1.000000000000000000, 0.000000000000000000 ) ) ;
#10437=LINE ( 'NONE', #1929, #6234 ) ;
#10443=VECTOR ( 'NONE', #11439, 1000.000000000000000 ) ;
#10445=FACE_OUTER_BOUND ( 'NONE', #3678, .T. ) ;
#10449=CARTESIAN_POINT ( 'NONE',  ( -71.24615306438109030, 31.99214930456376038, -167.1454815528550739 ) ) ;
#10450=DIRECTION ( 'NONE',  ( 0.000000000000000000, 0.000000000000000000, -1.000000000000000000 ) ) ;
#10452=FACE_OUTER_BOUND ( 'NONE', #12448, .T. ) ;
#10456=VECTOR ( 'NONE', #14434, 1000.000000000000000 ) ;
#10459=VECTOR ( 'NONE', #14946, 1000.000000000000114 ) ;
#10473=ORIENTED_EDGE ( 'NONE', *, *, #13183, .F. ) ;
#10476=CARTESIAN_POINT ( 'NONE',  ( -127.5926225674732279, 187.7866419848965052, 15.00000000000004263 ) ) ;
#10477=ORIENTED_EDGE ( 'NONE', *, *, #9560, .F. ) ;
#10478=VECTOR ( 'NONE', #11373, 1000.000000000000000 ) ;
#10483=VECTOR ( 'NONE', #3867, 1000.000000000000000 ) ;
#10484=VERTEX_POINT ( 'NONE', #12769 ) ;
#10485=EDGE_CURVE ( 'NONE', #8500, #6562, #18467, .T. ) ;
#10491=ORIENTED_EDGE ( 'NONE', *, *, #14729, .T. ) ;
#10493=DIRECTION ( 'NONE',  ( -1.156482317317869999E-16, 0.000000000000000000, -1.000000000000000000 ) ) ;
#10495=LINE ( 'NONE', #863, #14432 ) ;
#10500=FACE_OUTER_BOUND ( 'NONE', #13345, .T. ) ;
#10502=LINE ( 'NONE', #16200, #18176 ) ;
#10505=VERTEX_POINT ( 'NONE', #5545 ) ;
#10506=VERTEX_POINT ( 'NONE', #8552 ) ;
#10507=EDGE_CURVE ( 'NONE', #16077, #8426, #7137, .T. ) ;
#10508=EDGE_CURVE ( 'NONE', #1230, #9843, #11614, .T. ) ;
#10512=LINE ( 'NONE', #14813, #17393 ) ;
#10516=ORIENTED_EDGE ( 'NONE', *, *, #2899, .T. ) ;
#10520=EDGE_CURVE ( 'NONE', #13807, #7544, #10121, .T. ) ;
#10523=EDGE_LOOP ( 'NONE', ( #15477, #25, #9876, #8885 ) ) ;
#10525=AXIS2_PLACEMENT_3D ( 'NONE', #16972, #12695, #9969 ) ;
#10526=EDGE_CURVE ( 'NONE', #15988, #10428, #8994, .T. ) ;
#10533=VECTOR ( 'NONE', #15794, 1000.000000000000000 ) ;
#10534=EDGE_CURVE ( 'NONE', #5330, #18127, #7489, .T. ) ;
#10542=DIRECTION ( 'NONE',  ( -0.9396926207859084279, 0.3420201433256686574, 0.000000000000000000 ) ) ;
#10549=LINE ( 'NONE', #2122, #182 ) ;
#10550=LINE ( 'NONE', #17644, #1378 ) ;
#10555=DIRECTION ( 'NONE',  ( 0.9396926207859185309, 0.3420201433256406798, -1.086737899653001478E-16 ) ) ;
#10557=ADVANCED_FACE ( 'NONE', ( #16004 ), #17307, .T. ) ;
#10560=VECTOR ( 'NONE', #9630, 1000.000000000000114 ) ;
#10561=VERTEX_POINT ( 'NONE', #4674 ) ;
#10563=ORIENTED_EDGE ( 'NONE', *, *, #7346, .T. ) ;
#10567=DIRECTION ( 'NONE',  ( 0.9396926207859084279, 0.3420201433256686574, 0.000000000000000000 ) ) ;
#10571=DIRECTION ( 'NONE',  ( 0.9396926207859078728, 0.3420201433256701007, 4.890320548438446933E-16 ) ) ;
#10572=VECTOR ( 'NONE', #14880, 1000.000000000000000 ) ;
#10576=DIRECTION ( 'NONE',  ( -0.9396926207859084279, 0.3420201433256686574, -4.890320548438448905E-16 ) ) ;
#10582=PLANE ( 'NONE',  #2853 ) ;
#10589=ORIENTED_EDGE ( 'NONE', *, *, #17940, .T. ) ;
#10594=PLANE ( 'NONE',  #3967 ) ;
#10598=DIRECTION ( 'NONE',  ( 0.9396926207859065405, 0.3420201433256737089, 4.890320548438440031E-16 ) ) ;
#10599=ORIENTED_EDGE ( 'NONE', *, *, #17045, .T. ) ;
#10605=EDGE_LOOP ( 'NONE', ( #3492, #14897, #7977, #7148 ) ) ;
#10609=DIRECTION ( 'NONE',  ( 0.000000000000000000, 0.000000000000000000, 1.000000000000000000 ) ) ;
#10614=AXIS2_PLACEMENT_3D ( 'NONE', #9323, #6500, #15019 ) ;
#10615=DIRECTION ( 'NONE',  ( 1.000000000000000000, 0.000000000000000000, 0.000000000000000000 ) ) ;
#10619=LINE ( 'NONE', #9210, #8091 ) ;
#10622=CARTESIAN_POINT ( 'NONE',  ( -68.99615306438111872, 8.293196988130274505, -167.1454815528550739 ) ) ;
#10626=EDGE_CURVE ( 'NONE', #4697, #5159, #1609, .T. ) ;
#10634=EDGE_CURVE ( 'NONE', #13457, #2374, #13115, .T. ) ;
#10635=VERTEX_POINT ( 'NONE', #5136 ) ;
#10637=DIRECTION ( 'NONE',  ( 0.000000000000000000, 1.000000000000000000, 0.000000000000000000 ) ) ;
#10638=DIRECTION ( 'NONE',  ( 0.9396926207859185309, 0.3420201433256406798, 0.000000000000000000 ) ) ;
#10641=CARTESIAN_POINT ( 'NONE',  ( -71.24615306438079188, 113.6735582045637045, -167.1454815528550739 ) ) ;
#10642=CARTESIAN_POINT ( 'NONE',  ( -68.99615306438104767, 36.56753083813026706, -15.00000000000001421 ) ) ;
#10644=ORIENTED_EDGE ( 'NONE', *, *, #17047, .F. ) ;
#10655=EDGE_CURVE ( 'NONE', #3274, #6455, #9451, .T. ) ;
#10656=DIRECTION ( 'NONE',  ( 0.000000000000000000, 1.000000000000000000, 0.000000000000000000 ) ) ;
#10662=ORIENTED_EDGE ( 'NONE', *, *, #2874, .T. ) ;
#10666=EDGE_CURVE ( 'NONE', #8044, #15152, #3747, .T. ) ;
#10671=VERTEX_POINT ( 'NONE', #6159 ) ;
#10673=DIRECTION ( 'NONE',  ( 0.3420201433256661594, 0.9396926207859093161, -0.000000000000000000 ) ) ;
#10674=ORIENTED_EDGE ( 'NONE', *, *, #13221, .T. ) ;
#10675=DIRECTION ( 'NONE',  ( 0.000000000000000000, 1.000000000000000000, 0.000000000000000000 ) ) ;
#10676=ORIENTED_EDGE ( 'NONE', *, *, #11577, .T. ) ;
#10679=DIRECTION ( 'NONE',  ( 0.000000000000000000, 0.000000000000000000, 1.000000000000000000 ) ) ;
#10681=DIRECTION ( 'NONE',  ( -0.9396926207859084279, 0.3420201433256686574, 0.000000000000000000 ) ) ;
#10682=ORIENTED_EDGE ( 'NONE', *, *, #1271, .T. ) ;
#10683=LINE ( 'NONE', #10774, #9248 ) ;
#10686=LINE ( 'NONE', #17593, #3628 ) ;
#10687=DIRECTION ( 'NONE',  ( -0.9396926207859022107, 0.3420201433256853663, 0.000000000000000000 ) ) ;
#10689=EDGE_LOOP ( 'NONE', ( #9734, #5996, #10272, #2487 ) ) ;
#10693=ORIENTED_EDGE ( 'NONE', *, *, #16155, .F. ) ;
#10695=VERTEX_POINT ( 'NONE', #12547 ) ;
#10700=VERTEX_POINT ( 'NONE', #10954 ) ;
#10703=ORIENTED_EDGE ( 'NONE', *, *, #226, .T. ) ;
#10704=LINE ( 'NONE', #9306, #9002 ) ;
#10706=LINE ( 'NONE', #16399, #15604 ) ;
#10707=FACE_OUTER_BOUND ( 'NONE', #14714, .T. ) ;
#10708=CARTESIAN_POINT ( 'NONE',  ( -71.24615306438104767, 35.13374195456378857, -15.00000000000001421 ) ) ;
#10710=LINE ( 'NONE', #5194, #2076 ) ;
#10711=ORIENTED_EDGE ( 'NONE', *, *, #18190, .T. ) ;
#10712=VERTEX_POINT ( 'NONE', #3831 ) ;
#10713=VERTEX_POINT ( 'NONE', #3926 ) ;
#10717=ADVANCED_FACE ( 'NONE', ( #13850 ), #15344, .T. ) ;
#10718=CARTESIAN_POINT ( 'NONE',  ( -68.99615306438117557, 2.010011688130281193, -167.1454815528550739 ) ) ;
#10730=CARTESIAN_POINT ( 'NONE',  ( -71.24615306438079188, 116.8151508545637114, -15.00000000000001421 ) ) ;
#10733=ADVANCED_FACE ( 'NONE', ( #8240 ), #12361, .T. ) ;
#10734=FACE_OUTER_BOUND ( 'NONE', #1434, .T. ) ;
#10735=ORIENTED_EDGE ( 'NONE', *, *, #9022, .T. ) ;
#10736=VECTOR ( 'NONE', #2086, 1000.000000000000114 ) ;
#10737=ORIENTED_EDGE ( 'NONE', *, *, #16354, .T. ) ;
#10738=VECTOR ( 'NONE', #1648, 1000.000000000000000 ) ;
#10740=CARTESIAN_POINT ( 'NONE',  ( -68.99615306438072082, 133.3420471316626958, 15.00000000000006928 ) ) ;
#10742=ORIENTED_EDGE ( 'NONE', *, *, #4566, .T. ) ;
#10749=PLANE ( 'NONE',  #14117 ) ;
#10750=ORIENTED_EDGE ( 'NONE', *, *, #13373, .F. ) ;
#10752=EDGE_CURVE ( 'NONE', #5168, #14197, #723, .T. ) ;
#10754=VECTOR ( 'NONE', #11594, 1000.000000000000000 ) ;
#10757=ORIENTED_EDGE ( 'NONE', *, *, #13469, .F. ) ;
#10759=DIRECTION ( 'NONE',  ( 0.000000000000000000, 1.000000000000000000, 0.000000000000000000 ) ) ;
#10769=DIRECTION ( 'NONE',  ( 0.000000000000000000, 0.000000000000000000, 1.000000000000000000 ) ) ;
#10770=DIRECTION ( 'NONE',  ( -0.9396926207859097602, 0.3420201433256649937, 1.086737899652991371E-16 ) ) ;
#10772=LINE ( 'NONE', #4768, #12036 ) ;
#10773=ORIENTED_EDGE ( 'NONE', *, *, #15795, .F. ) ;
#10774=CARTESIAN_POINT ( 'NONE',  ( -68.99615306438091977, 76.79337943166271430, -15.00000000000001421 ) ) ;
#10775=PLANE ( 'NONE',  #4525 ) ;
#10776=EDGE_LOOP ( 'NONE', ( #6102, #1552, #11272, #8295 ) ) ;
#10784=ORIENTED_EDGE ( 'NONE', *, *, #10078, .F. ) ;
#10786=VECTOR ( 'NONE', #7362, 1000.000000000000000 ) ;
#10788=ORIENTED_EDGE ( 'NONE', *, *, #2999, .F. ) ;
#10789=ORIENTED_EDGE ( 'NONE', *, *, #11202, .F. ) ;
#10790=VECTOR ( 'NONE', #7152, 1000.000000000000000 ) ;
#10795=VECTOR ( 'NONE', #2347, 999.9999999999998863 ) ;
#10796=VECTOR ( 'NONE', #11647, 1000.000000000000000 ) ;
#10797=CARTESIAN_POINT ( 'NONE',  ( -68.99615306438083451, 96.25779118813026969, -167.1454815528550739 ) ) ;
#10798=LINE ( 'NONE', #10904, #17753 ) ;
#10799=ORIENTED_EDGE ( 'NONE', *, *, #13710, .F. ) ;
#10801=CARTESIAN_POINT ( 'NONE',  ( -68.99615306438067819, 142.7668250816626596, -15.00000000000001421 ) ) ;
#10803=ORIENTED_EDGE ( 'NONE', *, *, #13606, .F. ) ;
#10809=AXIS2_PLACEMENT_3D ( 'NONE', #11308, #12725, #18421 ) ;
#10813=PLANE ( 'NONE',  #11761 ) ;
#10814=DIRECTION ( 'NONE',  ( 0.000000000000000000, 0.000000000000000000, -1.000000000000000000 ) ) ;
#10815=VECTOR ( 'NONE', #8670, 1000.000000000000000 ) ;
#10818=LINE ( 'NONE', #10642, #3370 ) ;
#10820=ORIENTED_EDGE ( 'NONE', *, *, #7909, .T. ) ;
#10821=EDGE_CURVE ( 'NONE', #18179, #1519, #894, .T. ) ;
#10827=EDGE_LOOP ( 'NONE', ( #11049, #5029, #18160, #15687 ) ) ;
#10832=ADVANCED_FACE ( 'NONE', ( #12039 ), #18014, .T. ) ;
#10833=CARTESIAN_POINT ( 'NONE',  ( -71.24615306438091977, 71.94398301522919326, -15.00000000000001421 ) ) ;
#10835=ORIENTED_EDGE ( 'NONE', *, *, #333, .T. ) ;
#10836=ORIENTED_EDGE ( 'NONE', *, *, #4430, .F. ) ;
#10838=VECTOR ( 'NONE', #2945, 1000.000000000000000 ) ;
#10842=CARTESIAN_POINT ( 'NONE',  ( -68.99615306438100504, 39.70912348813028103, -167.1454815528550739 ) ) ;
#10845=CARTESIAN_POINT ( 'NONE',  ( -71.24615306438097662, 56.23601976522923707, 15.00000000000006928 ) ) ;
#10850=CARTESIAN_POINT ( 'NONE',  ( -71.24615306438100504, 53.09442711522921599, -15.00000000000001421 ) ) ;
#10858=DIRECTION ( 'NONE',  ( 0.9396926207859069846, 0.3420201433256723766, -1.086737899652988166E-16 ) ) ;
#10859=ORIENTED_EDGE ( 'NONE', *, *, #8600, .T. ) ;
#10861=ORIENTED_EDGE ( 'NONE', *, *, #16346, .T. ) ;
#10874=ORIENTED_EDGE ( 'NONE', *, *, #14412, .T. ) ;
#10876=CARTESIAN_POINT ( 'NONE',  ( -71.24615306438070661, 141.9478920545637664, -167.1454815528550739 ) ) ;
#10883=ADVANCED_FACE ( 'NONE', ( #16410 ), #5097, .T. ) ;
#10884=EDGE_CURVE ( 'NONE', #4573, #677, #16323, .T. ) ;
#10886=ADVANCED_FACE ( 'NONE', ( #13633 ), #808, .T. ) ;
#10888=VECTOR ( 'NONE', #16089, 1000.000000000000000 ) ;
#10892=ORIENTED_EDGE ( 'NONE', *, *, #3995, .F. ) ;
#10893=VECTOR ( 'NONE', #11178, 1000.000000000000000 ) ;
#10894=DIRECTION ( 'NONE',  ( 0.000000000000000000, 0.000000000000000000, 1.000000000000000000 ) ) ;
#10896=PLANE ( 'NONE',  #13803 ) ;
#10899=AXIS2_PLACEMENT_3D ( 'NONE', #7628, #13243, #11573 ) ;
#10904=CARTESIAN_POINT ( 'NONE',  ( -71.24615306438069240, 138.8062994045637311, -15.00000000000001421 ) ) ;
#10905=VERTEX_POINT ( 'NONE', #16897 ) ;
#10907=CARTESIAN_POINT ( 'NONE',  ( -71.24615306438109030, 28.85055665456373575, -167.1454815528550739 ) ) ;
#10915=LINE ( 'NONE', #11931, #7745 ) ;
#10917=ORIENTED_EDGE ( 'NONE', *, *, #3001, .T. ) ;
#10918=VECTOR ( 'NONE', #16138, 1000.000000000000000 ) ;
#10921=DIRECTION ( 'NONE',  ( 0.000000000000000000, 1.000000000000000000, 0.000000000000000000 ) ) ;
#10922=CARTESIAN_POINT ( 'NONE',  ( -68.99615306438104767, 30.28434553813026398, -15.00000000000001421 ) ) ;
#10924=VERTEX_POINT ( 'NONE', #9701 ) ;
#10925=LINE ( 'NONE', #9794, #17902 ) ;
#10931=CARTESIAN_POINT ( 'NONE',  ( -71.24615306438103346, 46.81124181522922356, -15.00000000000001421 ) ) ;
#10932=AXIS2_PLACEMENT_3D ( 'NONE', #12227, #8008, #3997 ) ;
#10933=LINE ( 'NONE', #15421, #12008 ) ;
#10934=CARTESIAN_POINT ( 'NONE',  ( -71.24615306438080609, 103.3599095152292193, -15.00000000000001421 ) ) ;
#10938=VERTEX_POINT ( 'NONE', #5662 ) ;
#10939=CARTESIAN_POINT ( 'NONE',  ( -68.99615306438080609, 105.6825691381303045, -167.1454815528550739 ) ) ;
#10941=ORIENTED_EDGE ( 'NONE', *, *, #8936, .F. ) ;
#10942=ADVANCED_FACE ( 'NONE', ( #5295 ), #16793, .T. ) ;
#10943=VERTEX_POINT ( 'NONE', #2681 ) ;
#10945=EDGE_CURVE ( 'NONE', #18464, #5754, #17083, .T. ) ;
#10948=DIRECTION ( 'NONE',  ( 0.000000000000000000, 0.000000000000000000, 1.000000000000000000 ) ) ;
#10954=CARTESIAN_POINT ( 'NONE',  ( -68.99615306438097662, 58.55867938813025830, 15.00000000000006928 ) ) ;
#10960=VERTEX_POINT ( 'NONE', #11010 ) ;
#10961=ORIENTED_EDGE ( 'NONE', *, *, #3771, .F. ) ;
#10963=LINE ( 'NONE', #17029, #16556 ) ;
#10964=CARTESIAN_POINT ( 'NONE',  ( -71.24615306438117557, 3.717815454563750954, -167.1454815528550739 ) ) ;
#10966=CARTESIAN_POINT ( 'NONE',  ( -71.24615306438076345, 119.0678727652292253, 15.00000000000006928 ) ) ;
#10967=EDGE_CURVE ( 'NONE', #425, #4999, #3886, .T. ) ;
#10975=CARTESIAN_POINT ( 'NONE',  ( -68.99615306438086293, 89.35975003166268493, 15.00000000000006928 ) ) ;
#10977=EDGE_LOOP ( 'NONE', ( #8366, #2393, #18039, #14245 ) ) ;
#10978=VERTEX_POINT ( 'NONE', #11105 ) ;
#10980=EDGE_CURVE ( 'NONE', #4127, #18127, #14006, .T. ) ;
#10982=LINE ( 'NONE', #594, #9709 ) ;
#10987=EDGE_CURVE ( 'NONE', #10700, #16781, #18120, .T. ) ;
#10993=FACE_OUTER_BOUND ( 'NONE', #14898, .T. ) ;
#10997=DIRECTION ( 'NONE',  ( 0.000000000000000000, 0.000000000000000000, 1.000000000000000000 ) ) ;
#11003=ORIENTED_EDGE ( 'NONE', *, *, #4378, .F. ) ;
#11004=ADVANCED_FACE ( 'NONE', ( #12516 ), #1287, .T. ) ;
#11005=EDGE_CURVE ( 'NONE', #11474, #14401, #12713, .T. ) ;
#11009=DIRECTION ( 'NONE',  ( 0.000000000000000000, 0.000000000000000000, 1.000000000000000000 ) ) ;
#11010=CARTESIAN_POINT ( 'NONE',  ( -68.99615306438077766, 117.6340838816626899, -15.00000000000001421 ) ) ;
#11017=EDGE_LOOP ( 'NONE', ( #7211, #14659, #17641, #8237 ) ) ;
#11024=FACE_OUTER_BOUND ( 'NONE', #10776, .T. ) ;
#11028=VERTEX_POINT ( 'NONE', #59 ) ;
#11029=VERTEX_POINT ( 'NONE', #16112 ) ;
#11036=CARTESIAN_POINT ( 'NONE',  ( -68.99615306438083451, 102.5409764881302692, 15.00000000000006928 ) ) ;
#11037=CARTESIAN_POINT ( 'NONE',  ( -71.24615306438109030, 24.82009326522924297, 15.00000000000006928 ) ) ;
#11038=FACE_OUTER_BOUND ( 'NONE', #17165, .T. ) ;
#11039=CARTESIAN_POINT ( 'NONE',  ( -71.24615306438113294, 10.00100075456376025, -15.00000000000001421 ) ) ;
#11042=DIRECTION ( 'NONE',  ( 0.000000000000000000, 0.000000000000000000, -1.000000000000000000 ) ) ;
#11043=FACE_OUTER_BOUND ( 'NONE', #2971, .T. ) ;
#11044=AXIS2_PLACEMENT_3D ( 'NONE', #12599, #16974, #5286 ) ;
#11046=CARTESIAN_POINT ( 'NONE',  ( -71.24615306438117557, 6.859408104563785358, -167.1454815528550739 ) ) ;
#11047=VECTOR ( 'NONE', #6798, 1000.000000000000000 ) ;
#11049=ORIENTED_EDGE ( 'NONE', *, *, #8004, .F. ) ;
#11050=ORIENTED_EDGE ( 'NONE', *, *, #5959, .T. ) ;
#11051=EDGE_LOOP ( 'NONE', ( #17841, #17101, #9334, #4826 ) ) ;
#11052=PLANE ( 'NONE',  #17453 ) ;
#11057=DIRECTION ( 'NONE',  ( 0.000000000000000000, 1.000000000000000000, 0.000000000000000000 ) ) ;
#11059=DIRECTION ( 'NONE',  ( 1.000000000000000000, 0.000000000000000000, 0.000000000000000000 ) ) ;
#11060=FACE_OUTER_BOUND ( 'NONE', #15183, .T. ) ;
#11061=ORIENTED_EDGE ( 'NONE', *, *, #14739, .F. ) ;
#11062=CARTESIAN_POINT ( 'NONE',  ( -71.24615306438111872, 21.67850061522927518, -167.1454815528550739 ) ) ;
#11066=DIRECTION ( 'NONE',  ( 0.000000000000000000, 0.000000000000000000, -1.000000000000000000 ) ) ;
#11071=EDGE_CURVE ( 'NONE', #7151, #10506, #17524, .T. ) ;
#11093=ORIENTED_EDGE ( 'NONE', *, *, #930, .F. ) ;
#11096=VECTOR ( 'NONE', #4879, 1000.000000000000000 ) ;
#11098=CARTESIAN_POINT ( 'NONE',  ( -71.24615306438091977, 78.22716831522920700, -167.1454815528550739 ) ) ;
#11100=EDGE_CURVE ( 'NONE', #5307, #10700, #7165, .T. ) ;
#11104=PLANE ( 'NONE',  #15662 ) ;
#11105=CARTESIAN_POINT ( 'NONE',  ( -71.24615306438080609, 106.5015021652292404, 15.00000000000006928 ) ) ;
#11106=ORIENTED_EDGE ( 'NONE', *, *, #137, .T. ) ;
#11107=EDGE_CURVE ( 'NONE', #12056, #593, #17177, .T. ) ;
#11109=CARTESIAN_POINT ( 'NONE',  ( -71.24615306438097662, 60.26648315456372984, 15.00000000000006928 ) ) ;
#11110=DIRECTION ( 'NONE',  ( 0.9396926207859158664, 0.3420201433256481738, 0.000000000000000000 ) ) ;
#11112=LINE ( 'NONE', #12800, #12394 ) ;
#11117=DIRECTION ( 'NONE',  ( 0.9396926207859145341, 0.3420201433256518375, -1.086737899652996918E-16 ) ) ;
#11118=LINE ( 'NONE', #5304, #12112 ) ;
#11119=EDGE_CURVE ( 'NONE', #13022, #10671, #320, .T. ) ;
#11120=CARTESIAN_POINT ( 'NONE',  ( -68.99615306438083451, 95.64293533166268446, -15.00000000000001421 ) ) ;
#11121=CARTESIAN_POINT ( 'NONE',  ( -68.99615306438097662, 61.70027203813028649, -167.1454815528550739 ) ) ;
#11124=FACE_OUTER_BOUND ( 'NONE', #12994, .T. ) ;
#11125=CARTESIAN_POINT ( 'NONE',  ( -68.99615306438091977, 76.79337943166271430, -167.1454815528550739 ) ) ;
#11126=EDGE_CURVE ( 'NONE', #4281, #12749, #161, .T. ) ;
#11131=VERTEX_POINT ( 'NONE', #8759 ) ;
#11132=VECTOR ( 'NONE', #16221, 1000.000000000000000 ) ;
#11135=VECTOR ( 'NONE', #15313, 999.9999999999998863 ) ;
#11136=DIRECTION ( 'NONE',  ( -0.9396926207859069846, 0.3420201433256723766, -4.890320548438442003E-16 ) ) ;
#11139=ORIENTED_EDGE ( 'NONE', *, *, #7483, .T. ) ;
#11141=CARTESIAN_POINT ( 'NONE',  ( -71.24615306438099083, 35.13374195456380278, 15.00000000000006928 ) ) ;
#11145=VECTOR ( 'NONE', #9958, 1000.000000000000000 ) ;
#11147=EDGE_LOOP ( 'NONE', ( #13555, #10874, #15408, #3468 ) ) ;
#11151=DIRECTION ( 'NONE',  ( 0.3420201433256444545, -0.9396926207859171987, 0.000000000000000000 ) ) ;
#11152=VERTEX_POINT ( 'NONE', #7523 ) ;
#11154=VERTEX_POINT ( 'NONE', #14549 ) ;
#11156=DIRECTION ( 'NONE',  ( 0.9396926207859158664, 0.3420201433256481738, -1.086737899652998397E-16 ) ) ;
#11162=AXIS2_PLACEMENT_3D ( 'NONE', #5632, #2565, #12570 ) ;
#11164=LINE ( 'NONE', #4055, #7511 ) ;
#11165=ORIENTED_EDGE ( 'NONE', *, *, #13978, .F. ) ;
#11166=PLANE ( 'NONE',  #5718 ) ;
#11168=CARTESIAN_POINT ( 'NONE',  ( -68.99615306438091977, 74.26664263813029265, -15.00000000000001421 ) ) ;
#11178=DIRECTION ( 'NONE',  ( 0.000000000000000000, 0.000000000000000000, 1.000000000000000000 ) ) ;
#11179=CARTESIAN_POINT ( 'NONE',  ( -68.99615306438103346, 32.81108233166271759, -15.00000000000001421 ) ) ;
#11181=VERTEX_POINT ( 'NONE', #418 ) ;
#11183=VERTEX_POINT ( 'NONE', #12247 ) ;
#11184=DIRECTION ( 'NONE',  ( 0.000000000000000000, 0.000000000000000000, 1.000000000000000000 ) ) ;
#11186=ORIENTED_EDGE ( 'NONE', *, *, #10626, .F. ) ;
#11187=CARTESIAN_POINT ( 'NONE',  ( -68.99615306438111872, 13.96152643166267993, 15.00000000000006928 ) ) ;
#11188=CARTESIAN_POINT ( 'NONE',  ( -71.24615306438114715, 15.39531531522927921, -167.1454815528550739 ) ) ;
#11192=ORIENTED_EDGE ( 'NONE', *, *, #4129, .T. ) ;
#11197=LINE ( 'NONE', #8383, #13605 ) ;
#11198=AXIS2_PLACEMENT_3D ( 'NONE', #12196, #6572, #17803 ) ;
#11200=ORIENTED_EDGE ( 'NONE', *, *, #12738, .F. ) ;
#11201=VECTOR ( 'NONE', #2309, 1000.000000000000000 ) ;
#11202=EDGE_CURVE ( 'NONE', #2538, #7201, #3741, .T. ) ;
#11206=ORIENTED_EDGE ( 'NONE', *, *, #6061, .F. ) ;
#11208=EDGE_LOOP ( 'NONE', ( #1362, #14994, #14974, #2441, #5966, #15780, #18145, #15111, #2109, #5569, #7422, #12877, #14571, #508, #16136, #10961, #12450, #16911, #9833, #8542, #16006, #13016, #5176, #4690, #1522, #11606, #8484, #3581, #7140, #12980, #10070, #10103, #15901, #9645, #5788, #4131, #5104, #17335, #17125, #3516, #12930, #11186, #54, #6835, #17652, #13105, #5092, #12370, #14910, #14411, #1671, #15447, #12572, #2625, #14003, #8247, #15683, #2967, #7246, #9131, #12508, #5311, #6451, #4241, #5239, #13773, #6366, #13173, #15568, #10051, #17185, #8978, #6033, #16679, #18210, #10195, #12388, #15016, #3347, #2854, #10836, #6436, #13244, #10789, #2593, #16887, #9913, #12293, #2656, #12773, #3895, #9743, #6233, #6595, #17897, #10892, #16767, #4834, #6945, #13785, #13532, #10788, #12239, #15484, #17072, #2564, #10757, #16316, #7690, #15490, #9409, #4862, #1467, #18400, #8620, #1718, #7846, #7053, #12675, #14109, #7410, #2230, #7021, #7565, #2413, #7701, #14882, #382, #4752, #14893, #12768, #3161, #10750, #9943, #8221, #12138, #16639, #4365, #14437, #2399, #6256, #339, #8749, #8371, #5601, #8951, #6164, #783, #14277, #10799, #14087, #7862, #17328, #12756, #4883, #9900, #12715, #8558, #7018, #16966, #10047, #6113, #16257, #14065, #13084, #7498, #3986, #15940, #9941, #16818, #12647, #10773, #6858, #3813, #1776, #7514, #15511, #4903, #18475, #4415, #11922, #12735, #18411, #2253, #7299, #5729, #4204, #1547, #10044, #521, #16407, #7656, #11200, #2753, #14377, #4571, #4484 ) ) ;
#11210=LINE ( 'NONE', #5298, #6540 ) ;
#11213=VERTEX_POINT ( 'NONE', #6444 ) ;
#11217=DIRECTION ( 'NONE',  ( 0.3420201433256637724, -0.9396926207859102043, 0.000000000000000000 ) ) ;
#11225=CARTESIAN_POINT ( 'NONE',  ( -68.99615306438087714, 67.98345733813025049, -15.00000000000001421 ) ) ;
#11230=VERTEX_POINT ( 'NONE', #9733 ) ;
#11250=CARTESIAN_POINT ( 'NONE',  ( -71.24615306438099083, 53.98329785456374452, -15.00000000000001421 ) ) ;
#11252=EDGE_CURVE ( 'NONE', #5754, #5470, #6822, .T. ) ;
#11254=DIRECTION ( 'NONE',  ( 0.000000000000000000, 1.000000000000000000, 0.000000000000000000 ) ) ;
#11255=ORIENTED_EDGE ( 'NONE', *, *, #6641, .F. ) ;
#11256=ORIENTED_EDGE ( 'NONE', *, *, #13063, .F. ) ;
#11260=DIRECTION ( 'NONE',  ( -0.9396926207859158664, 0.3420201433256481738, 0.000000000000000000 ) ) ;
#11261=PLANE ( 'NONE',  #15635 ) ;
#11263=DIRECTION ( 'NONE',  ( -0.9396926207859093161, 0.3420201433256663814, -4.890320548438453836E-16 ) ) ;
#11264=PLANE ( 'NONE',  #6936 ) ;
#11266=ORIENTED_EDGE ( 'NONE', *, *, #17045, .F. ) ;
#11272=ORIENTED_EDGE ( 'NONE', *, *, #12503, .T. ) ;
#11273=DIRECTION ( 'NONE',  ( 0.3420201433256802037, -0.9396926207859043201, 0.000000000000000000 ) ) ;
#11277=DIRECTION ( 'NONE',  ( 0.000000000000000000, 0.000000000000000000, -1.000000000000000000 ) ) ;
#11278=VERTEX_POINT ( 'NONE', #2422 ) ;
#11281=CARTESIAN_POINT ( 'NONE',  ( -71.24615306438083451, 97.96559495456375544, -167.1454815528550739 ) ) ;
#11282=CARTESIAN_POINT ( 'NONE',  ( -71.24615306438111872, 22.56737135456379661, 15.00000000000006928 ) ) ;
#11286=DIRECTION ( 'NONE',  ( 0.000000000000000000, 0.000000000000000000, -1.000000000000000000 ) ) ;
#11291=ORIENTED_EDGE ( 'NONE', *, *, #5471, .T. ) ;
#11292=FACE_OUTER_BOUND ( 'NONE', #16428, .T. ) ;
#11293=VERTEX_POINT ( 'NONE', #11322 ) ;
#11297=CARTESIAN_POINT ( 'NONE',  ( -71.24615306438083451, 97.07672421522921979, -167.1454815528550739 ) ) ;
#11298=DIRECTION ( 'NONE',  ( -0.9396926207859093161, 0.3420201433256661039, -4.890320548438453836E-16 ) ) ;
#11299=ORIENTED_EDGE ( 'NONE', *, *, #15515, .T. ) ;
#11300=LINE ( 'NONE', #10245, #9859 ) ;
#11301=LINE ( 'NONE', #15302, #7727 ) ;
#11302=PLANE ( 'NONE',  #12969 ) ;
#11303=DIRECTION ( 'NONE',  ( -0.9396926207859145341, 0.3420201433256519485, 0.000000000000000000 ) ) ;
#11304=ORIENTED_EDGE ( 'NONE', *, *, #2752, .T. ) ;
#11306=PLANE ( 'NONE',  #3399 ) ;
#11308=CARTESIAN_POINT ( 'NONE',  ( -68.99615306438077766, 118.2489397381302751, -167.1454815528550739 ) ) ;
#11309=ORIENTED_EDGE ( 'NONE', *, *, #12235, .T. ) ;
#11310=PLANE ( 'NONE',  #9414 ) ;
#11311=DIRECTION ( 'NONE',  ( 0.000000000000000000, 0.000000000000000000, -1.000000000000000000 ) ) ;
#11312=LINE ( 'NONE', #17002, #29 ) ;
#11313=LINE ( 'NONE', #6909, #12267 ) ;
#11315=ORIENTED_EDGE ( 'NONE', *, *, #6375, .T. ) ;
#11316=EDGE_CURVE ( 'NONE', #6650, #4400, #12914, .T. ) ;
#11322=CARTESIAN_POINT ( 'NONE',  ( -71.24615306438100504, 49.95283446522918780, -15.00000000000001421 ) ) ;
#11330=CARTESIAN_POINT ( 'NONE',  ( -71.24615306438070661, 138.8062994045637311, 15.00000000000006928 ) ) ;
#11336=EDGE_LOOP ( 'NONE', ( #15544, #11528, #13808, #4676 ) ) ;
#11339=VERTEX_POINT ( 'NONE', #88 ) ;
#11340=CARTESIAN_POINT ( 'NONE',  ( -71.24615306438091977, 78.22716831522920700, -15.00000000000001421 ) ) ;
#11341=FACE_OUTER_BOUND ( 'NONE', #4235, .T. ) ;
#11342=CARTESIAN_POINT ( 'NONE',  ( -68.99615306438070661, 136.4836397816626743, -15.00000000000001421 ) ) ;
#11346=EDGE_LOOP ( 'NONE', ( #5989, #11634, #14262, #13714 ) ) ;
#11348=EDGE_CURVE ( 'NONE', #4697, #10024, #4388, .T. ) ;
#11349=CARTESIAN_POINT ( 'NONE',  ( -68.99615306438080609, 108.8241617881302545, 15.00000000000006928 ) ) ;
#11351=CARTESIAN_POINT ( 'NONE',  ( -68.99615306438083451, 98.78452798166264870, 15.00000000000006928 ) ) ;
#11353=EDGE_CURVE ( 'NONE', #8311, #13617, #6917, .T. ) ;
#11359=ADVANCED_FACE ( 'NONE', ( #5872 ), #7024, .T. ) ;
#11360=AXIS2_PLACEMENT_3D ( 'NONE', #11633, #2947, #8651 ) ;
#11365=DIRECTION ( 'NONE',  ( 0.000000000000000000, 0.000000000000000000, -1.000000000000000000 ) ) ;
#11366=PLANE ( 'NONE',  #379 ) ;
#11371=CARTESIAN_POINT ( 'NONE',  ( -71.24615306438109030, 31.10327856522923540, 15.00000000000006928 ) ) ;
#11373=DIRECTION ( 'NONE',  ( 0.9396926207859084279, 0.3420201433256686574, 4.890320548438448905E-16 ) ) ;
#11376=VERTEX_POINT ( 'NONE', #10013 ) ;
#11378=ADVANCED_FACE ( 'NONE', ( #15724 ), #8606, .T. ) ;
#11379=PLANE ( 'NONE',  #14041 ) ;
#11382=ORIENTED_EDGE ( 'NONE', *, *, #16823, .F. ) ;
#11384=DIRECTION ( 'NONE',  ( 0.000000000000000000, 1.000000000000000000, 0.000000000000000000 ) ) ;
#11386=VECTOR ( 'NONE', #12734, 1000.000000000000000 ) ;
#11388=AXIS2_PLACEMENT_3D ( 'NONE', #7118, #2719, #12826 ) ;
#11389=DIRECTION ( 'NONE',  ( 0.9396926207859158664, 0.3420201433256481738, 0.000000000000000000 ) ) ;
#11392=DIRECTION ( 'NONE',  ( 1.000000000000000000, 0.000000000000000000, 0.000000000000000000 ) ) ;
#11397=ORIENTED_EDGE ( 'NONE', *, *, #16938, .F. ) ;
#11398=CARTESIAN_POINT ( 'NONE',  ( -71.24615306438089135, 84.51035361522924916, -15.00000000000001421 ) ) ;
#11399=FACE_OUTER_BOUND ( 'NONE', #4960, .T. ) ;
#11400=FACE_OUTER_BOUND ( 'NONE', #14278, .T. ) ;
#11403=LINE ( 'NONE', #12731, #1644 ) ;
#11407=AXIS2_PLACEMENT_3D ( 'NONE', #8664, #6111, #11838 ) ;
#11409=EDGE_LOOP ( 'NONE', ( #2588, #10737, #16039, #9024 ) ) ;
#11410=VERTEX_POINT ( 'NONE', #527 ) ;
#11412=ADVANCED_FACE ( 'NONE', ( #6039 ), #8963, .T. ) ;
#11416=DIRECTION ( 'NONE',  ( 0.000000000000000000, 0.000000000000000000, -1.000000000000000000 ) ) ;
#11421=CARTESIAN_POINT ( 'NONE',  ( -71.24615306438103346, 41.41692725456378099, -15.00000000000001421 ) ) ;
#11422=EDGE_LOOP ( 'NONE', ( #9563, #18375, #6925, #1685 ) ) ;
#11424=PLANE ( 'NONE',  #11388 ) ;
#11430=ORIENTED_EDGE ( 'NONE', *, *, #16169, .T. ) ;
#11431=AXIS2_PLACEMENT_3D ( 'NONE', #9899, #8505, #5673 ) ;
#11432=VECTOR ( 'NONE', #189, 1000.000000000000000 ) ;
#11436=CARTESIAN_POINT ( 'NONE',  ( -71.24615306438117557, 5.970537365229261262, -15.00000000000001421 ) ) ;
#11439=DIRECTION ( 'NONE',  ( 0.000000000000000000, 0.000000000000000000, 1.000000000000000000 ) ) ;
#11443=ORIENTED_EDGE ( 'NONE', *, *, #10420, .F. ) ;
#11445=CARTESIAN_POINT ( 'NONE',  ( -71.24615306438066398, 129.3815214545637389, 15.00000000000006928 ) ) ;
#11447=VECTOR ( 'NONE', #13779, 1000.000000000000000 ) ;
#11449=EDGE_LOOP ( 'NONE', ( #12854, #12979, #13081, #9708 ) ) ;
#11451=DIRECTION ( 'NONE',  ( -0.9396926207859157554, 0.3420201433256481738, -4.890320548438487362E-16 ) ) ;
#11452=VERTEX_POINT ( 'NONE', #4650 ) ;
#11453=VECTOR ( 'NONE', #15363, 1000.000000000000000 ) ;
#11454=EDGE_CURVE ( 'NONE', #11183, #14076, #16054, .T. ) ;
#11455=ADVANCED_FACE ( 'NONE', ( #17544 ), #8785, .T. ) ;
#11462=CARTESIAN_POINT ( 'NONE',  ( -68.99615306438083451, 98.78452798166264870, -167.1454815528550739 ) ) ;
#11471=ADVANCED_FACE ( 'NONE', ( #9146 ), #1670, .T. ) ;
#11474=VERTEX_POINT ( 'NONE', #17363 ) ;
#11476=ORIENTED_EDGE ( 'NONE', *, *, #716, .F. ) ;
#11477=EDGE_CURVE ( 'NONE', #288, #13807, #10271, .T. ) ;
#11478=( GEOMETRIC_REPRESENTATION_CONTEXT ( 3 ) GLOBAL_UNCERTAINTY_ASSIGNED_CONTEXT ( ( #15252 ) ) GLOBAL_UNIT_ASSIGNED_CONTEXT ( ( #14833, #5005, #13539 ) ) REPRESENTATION_CONTEXT ( 'NONE', 'WORKASPACE' ) );
#11481=EDGE_CURVE ( 'NONE', #14342, #9825, #14658, .T. ) ;
#11486=ORIENTED_EDGE ( 'NONE', *, *, #9126, .T. ) ;
#11488=LINE ( 'NONE', #3479, #6248 ) ;
#11490=DIRECTION ( 'NONE',  ( 1.000000000000000000, 0.000000000000000000, 0.000000000000000000 ) ) ;
#11494=DIRECTION ( 'NONE',  ( 0.000000000000000000, 0.000000000000000000, 1.000000000000000000 ) ) ;
#11495=CARTESIAN_POINT ( 'NONE',  ( -71.24615306438070661, 137.9174286652292096, -15.00000000000001421 ) ) ;
#11499=VECTOR ( 'NONE', #10381, 1000.000000000000114 ) ;
#11505=AXIS2_PLACEMENT_3D ( 'NONE', #16648, #15257, #2555 ) ;
#11512=DIRECTION ( 'NONE',  ( 0.000000000000000000, 0.000000000000000000, 1.000000000000000000 ) ) ;
#11516=DIRECTION ( 'NONE',  ( 0.000000000000000000, 0.000000000000000000, -1.000000000000000000 ) ) ;
#11520=CARTESIAN_POINT ( 'NONE',  ( -68.99615306438094819, 64.84186468813030046, 15.00000000000006928 ) ) ;
#11521=ORIENTED_EDGE ( 'NONE', *, *, #7501, .F. ) ;
#11523=DIRECTION ( 'NONE',  ( 0.000000000000000000, 0.000000000000000000, 1.000000000000000000 ) ) ;
#11526=DIRECTION ( 'NONE',  ( 0.9396926207859171987, 0.3420201433256444545, -1.086737899652999999E-16 ) ) ;
#11528=ORIENTED_EDGE ( 'NONE', *, *, #12927, .T. ) ;
#11529=ORIENTED_EDGE ( 'NONE', *, *, #7898, .F. ) ;
#11534=DIRECTION ( 'NONE',  ( 0.000000000000000000, 1.000000000000000000, 0.000000000000000000 ) ) ;
#11545=VERTEX_POINT ( 'NONE', #12328 ) ;
#11546=ORIENTED_EDGE ( 'NONE', *, *, #3008, .T. ) ;
#11557=CARTESIAN_POINT ( 'NONE',  ( -68.99615306438060713, 146.5232735881302517, 15.00000000000006928 ) ) ;
#11558=VERTEX_POINT ( 'NONE', #12431 ) ;
#11559=EDGE_CURVE ( 'NONE', #15985, #11213, #6603, .T. ) ;
#11560=CARTESIAN_POINT ( 'NONE',  ( -68.99615306438077766, 123.9172691816626610, 15.00000000000006928 ) ) ;
#11562=EDGE_CURVE ( 'NONE', #6571, #9843, #5103, .T. ) ;
#11564=ORIENTED_EDGE ( 'NONE', *, *, #762, .F. ) ;
#11567=CARTESIAN_POINT ( 'NONE',  ( -71.24615306438086293, 90.79353891522923448, 15.00000000000006928 ) ) ;
#11570=CARTESIAN_POINT ( 'NONE',  ( -93.54007869656273044, 187.7866419848965052, -15.00000000000001421 ) ) ;
#11571=CARTESIAN_POINT ( 'NONE',  ( -68.99615306438083451, 101.9261206316626698, 15.00000000000006928 ) ) ;
#11572=DIRECTION ( 'NONE',  ( -0.9396926207859008784, 0.3420201433256891965, 1.086737899652981141E-16 ) ) ;
#11573=DIRECTION ( 'NONE',  ( -0.9396926207859084279, 0.3420201433256686574, 0.000000000000000000 ) ) ;
#11576=CARTESIAN_POINT ( 'NONE',  ( -68.99615306438106188, 23.38630438166269698, 15.00000000000006928 ) ) ;
#11577=EDGE_CURVE ( 'NONE', #16048, #4518, #9326, .T. ) ;
#11593=ORIENTED_EDGE ( 'NONE', *, *, #7680, .T. ) ;
#11594=DIRECTION ( 'NONE',  ( 0.9396926207859084279, 0.3420201433256686574, 4.890320548438448905E-16 ) ) ;
#11604=ORIENTED_EDGE ( 'NONE', *, *, #13499, .F. ) ;
#11606=ORIENTED_EDGE ( 'NONE', *, *, #3, .F. ) ;
#11607=CARTESIAN_POINT ( 'NONE',  ( -71.24615306438070661, 138.8062994045637311, -167.1454815528550739 ) ) ;
#11608=DIRECTION ( 'NONE',  ( 0.000000000000000000, 0.000000000000000000, 1.000000000000000000 ) ) ;
#11611=CARTESIAN_POINT ( 'NONE',  ( -68.99615306438100504, 45.37745293166267402, -167.1454815528550739 ) ) ;
#11612=VERTEX_POINT ( 'NONE', #5007 ) ;
#11614=LINE ( 'NONE', #11445, #3084 ) ;
#11616=VECTOR ( 'NONE', #11254, 1000.000000000000000 ) ;
#11618=FACE_OUTER_BOUND ( 'NONE', #18387, .T. ) ;
#11620=ORIENTED_EDGE ( 'NONE', *, *, #8314, .F. ) ;
#11622=PRODUCT_DEFINITION ( 'UNKNOWN', '', #5483, #17679 ) ;
#11631=DIRECTION ( 'NONE',  ( -0.9396926207859158664, 0.3420201433256481738, 1.086737899652998397E-16 ) ) ;
#11632=ORIENTED_EDGE ( 'NONE', *, *, #10166, .T. ) ;
#11633=CARTESIAN_POINT ( 'NONE',  ( -68.99615306438083451, 101.9261206316626698, -167.1454815528550739 ) ) ;
#11634=ORIENTED_EDGE ( 'NONE', *, *, #16684, .T. ) ;
#11636=ORIENTED_EDGE ( 'NONE', *, *, #376, .F. ) ;
#11637=VECTOR ( 'NONE', #9874, 1000.000000000000000 ) ;
#11639=ORIENTED_EDGE ( 'NONE', *, *, #12398, .F. ) ;
#11644=ADVANCED_FACE ( 'NONE', ( #13638 ), #816, .T. ) ;
#11647=DIRECTION ( 'NONE',  ( 0.000000000000000000, 1.000000000000000000, 0.000000000000000000 ) ) ;
#11652=AXIS2_PLACEMENT_3D ( 'NONE', #13746, #6632, #17770 ) ;
#11654=DIRECTION ( 'NONE',  ( 0.000000000000000000, 1.000000000000000000, 0.000000000000000000 ) ) ;
#11656=EDGE_CURVE ( 'NONE', #11452, #2278, #15498, .T. ) ;
#11660=CARTESIAN_POINT ( 'NONE',  ( -71.24615306438100504, 49.95283446522918780, -15.00000000000001421 ) ) ;
#11661=ORIENTED_EDGE ( 'NONE', *, *, #8712, .T. ) ;
#11662=AXIS2_PLACEMENT_3D ( 'NONE', #7383, #13360, #5961 ) ;
#11663=ORIENTED_EDGE ( 'NONE', *, *, #13405, .F. ) ;
#11664=AXIS2_PLACEMENT_3D ( 'NONE', #10180, #4729, #11516 ) ;
#11665=ADVANCED_FACE ( 'NONE', ( #12989 ), #9993, .T. ) ;
#11667=EDGE_CURVE ( 'NONE', #5560, #4662, #2790, .T. ) ;
#11669=ADVANCED_FACE ( 'NONE', ( #18316 ), #7172, .T. ) ;
#11674=ADVANCED_FACE ( 'NONE', ( #9707 ), #15415, .T. ) ;
#11675=DIRECTION ( 'NONE',  ( 0.9396926207859084279, 0.3420201433256686574, 0.000000000000000000 ) ) ;
#11676=ORIENTED_EDGE ( 'NONE', *, *, #7019, .T. ) ;
#11679=LINE ( 'NONE', #17370, #6105 ) ;
#11681=DIRECTION ( 'NONE',  ( -0.9396926207859097602, 0.3420201433256649937, 0.000000000000000000 ) ) ;
#11685=EDGE_CURVE ( 'NONE', #3670, #11213, #11112, .T. ) ;
#11689=ORIENTED_EDGE ( 'NONE', *, *, #12346, .F. ) ;
#11692=ORIENTED_EDGE ( 'NONE', *, *, #11910, .F. ) ;
#11693=ORIENTED_EDGE ( 'NONE', *, *, #14734, .T. ) ;
#11694=AXIS2_PLACEMENT_3D ( 'NONE', #14350, #17160, #1538 ) ;
#11698=EDGE_CURVE ( 'NONE', #10905, #11612, #6998, .T. ) ;
#11700=DIRECTION ( 'NONE',  ( 0.000000000000000000, 0.000000000000000000, 1.000000000000000000 ) ) ;
#11710=CARTESIAN_POINT ( 'NONE',  ( -68.99615306438067819, 142.7668250816626596, -167.1454815528550739 ) ) ;
#11713=CARTESIAN_POINT ( 'NONE',  ( -68.99615306438106188, 27.14275288813031040, -167.1454815528550739 ) ) ;
#11714=VECTOR ( 'NONE', #14949, 1000.000000000000114 ) ;
#11717=VECTOR ( 'NONE', #17092, 1000.000000000000000 ) ;
#11718=FACE_OUTER_BOUND ( 'NONE', #8707, .T. ) ;
#11722=AXIS2_PLACEMENT_3D ( 'NONE', #12804, #5395, #8212 ) ;
#11727=LINE ( 'NONE', #18419, #4069 ) ;
#11732=VECTOR ( 'NONE', #2660, 1000.000000000000000 ) ;
#11733=LINE ( 'NONE', #14217, #13465 ) ;
#11740=DIRECTION ( 'NONE',  ( 1.000000000000000000, 0.000000000000000000, 0.000000000000000000 ) ) ;
#11742=AXIS2_PLACEMENT_3D ( 'NONE', #16140, #260, #3242 ) ;
#11745=CARTESIAN_POINT ( 'NONE',  ( -68.99615306438104767, 8.293196988130247860, 15.00000000000006928 ) ) ;
#11749=AXIS2_PLACEMENT_3D ( 'NONE', #13263, #10173, #16052 ) ;
#11754=VERTEX_POINT ( 'NONE', #5580 ) ;
#11761=AXIS2_PLACEMENT_3D ( 'NONE', #4818, #3421, #7721 ) ;
#11763=CARTESIAN_POINT ( 'NONE',  ( -71.24615306438103346, 43.66964916522919538, 15.00000000000006928 ) ) ;
#11767=FACE_OUTER_BOUND ( 'NONE', #8324, .T. ) ;
#11769=EDGE_LOOP ( 'NONE', ( #2155, #17525, #14115, #13072 ) ) ;
#11775=VECTOR ( 'NONE', #6895, 1000.000000000000000 ) ;
#11778=EDGE_CURVE ( 'NONE', #8597, #15702, #14206, .T. ) ;
#11784=EDGE_LOOP ( 'NONE', ( #18305, #17805, #1422, #1409 ) ) ;
#11796=DIRECTION ( 'NONE',  ( 0.9396926207859043201, 0.3420201433256802037, -1.086737899652985085E-16 ) ) ;
#11797=EDGE_CURVE ( 'NONE', #16527, #3118, #5930, .T. ) ;
#11803=AXIS2_PLACEMENT_3D ( 'NONE', #490, #15751, #3282 ) ;
#11806=CARTESIAN_POINT ( 'NONE',  ( -68.99615306438106188, 30.28434553813027108, -15.00000000000001421 ) ) ;
#11808=AXIS2_PLACEMENT_3D ( 'NONE', #3058, #14476, #17448 ) ;
#11809=CARTESIAN_POINT ( 'NONE',  ( -71.24615306438111872, 18.53690796522925055, -167.1454815528550739 ) ) ;
#11810=VECTOR ( 'NONE', #18393, 1000.000000000000114 ) ;
#11812=ADVANCED_FACE ( 'NONE', ( #14632 ), #1918, .T. ) ;
#11814=ORIENTED_EDGE ( 'NONE', *, *, #12242, .T. ) ;
#11815=EDGE_CURVE ( 'NONE', #103, #15787, #9032, .T. ) ;
#11818=CARTESIAN_POINT ( 'NONE',  ( -71.24615306438100504, 49.95283446522918780, 15.00000000000006928 ) ) ;
#11820=FACE_OUTER_BOUND ( 'NONE', #14026, .T. ) ;
#11823=VECTOR ( 'NONE', #2986, 1000.000000000000000 ) ;
#11824=ORIENTED_EDGE ( 'NONE', *, *, #9045, .T. ) ;
#11826=DIRECTION ( 'NONE',  ( 0.000000000000000000, 0.000000000000000000, 1.000000000000000000 ) ) ;
#11830=CARTESIAN_POINT ( 'NONE',  ( -68.99615306438089135, 67.36860148166267948, -167.1454815528550739 ) ) ;
#11832=DIRECTION ( 'NONE',  ( 0.000000000000000000, 0.000000000000000000, 1.000000000000000000 ) ) ;
#11838=DIRECTION ( 'NONE',  ( 0.000000000000000000, 0.000000000000000000, -1.000000000000000000 ) ) ;
#11842=DIRECTION ( 'NONE',  ( 0.000000000000000000, 0.000000000000000000, 1.000000000000000000 ) ) ;
#11845=EDGE_CURVE ( 'NONE', #6867, #1022, #5858, .T. ) ;
#11850=EDGE_LOOP ( 'NONE', ( #7826, #15013, #2095, #15803 ) ) ;
#11852=LINE ( 'NONE', #3513, #10918 ) ;
#11854=DIRECTION ( 'NONE',  ( 0.000000000000000000, 0.000000000000000000, 1.000000000000000000 ) ) ;
#11857=FACE_OUTER_BOUND ( 'NONE', #2946, .T. ) ;
#11858=DIRECTION ( 'NONE',  ( 0.9396926207859097602, 0.3420201433256649937, 0.000000000000000000 ) ) ;
#11859=DIRECTION ( 'NONE',  ( -0.9396926207859103153, 0.3420201433256634949, -4.890320548438458766E-16 ) ) ;
#11862=ORIENTED_EDGE ( 'NONE', *, *, #10303, .T. ) ;
#11863=LINE ( 'NONE', #7465, #2097 ) ;
#11868=ORIENTED_EDGE ( 'NONE', *, *, #7104, .F. ) ;
#11869=ORIENTED_EDGE ( 'NONE', *, *, #16353, .T. ) ;
#11873=EDGE_CURVE ( 'NONE', #1167, #10354, #6017, .T. ) ;
#11875=DIRECTION ( 'NONE',  ( 0.000000000000000000, 0.000000000000000000, 1.000000000000000000 ) ) ;
#11876=DIRECTION ( 'NONE',  ( -0.9396926207859084279, 0.3420201433256686574, 1.086737899652989892E-16 ) ) ;
#11877=DIRECTION ( 'NONE',  ( 0.000000000000000000, 1.000000000000000000, 0.000000000000000000 ) ) ;
#11879=ORIENTED_EDGE ( 'NONE', *, *, #4576, .T. ) ;
#11882=CARTESIAN_POINT ( 'NONE',  ( -68.99615306438083451, 95.64293533166268446, -167.1454815528550739 ) ) ;
#11884=ADVANCED_FACE ( 'NONE', ( #16213 ), #17528, .T. ) ;
#11886=DIRECTION ( 'NONE',  ( 0.3420201433256444545, 0.9396926207859171987, -0.000000000000000000 ) ) ;
#11893=EDGE_CURVE ( 'NONE', #12176, #5068, #10248, .T. ) ;
#11895=CARTESIAN_POINT ( 'NONE',  ( -71.24615306438086293, 94.82400230456377699, 15.00000000000006928 ) ) ;
#11898=DIRECTION ( 'NONE',  ( 0.000000000000000000, 1.000000000000000000, 0.000000000000000000 ) ) ;
#11906=VERTEX_POINT ( 'NONE', #3869 ) ;
#11907=DIRECTION ( 'NONE',  ( 1.000000000000000000, 0.000000000000000000, 0.000000000000000000 ) ) ;
#11910=EDGE_CURVE ( 'NONE', #4613, #14266, #8075, .T. ) ;
#11914=VECTOR ( 'NONE', #12717, 1000.000000000000000 ) ;
#11918=VERTEX_POINT ( 'NONE', #15100 ) ;
#11922=ORIENTED_EDGE ( 'NONE', *, *, #1512, .F. ) ;
#11923=DIRECTION ( 'NONE',  ( -0.9396926207859097602, 0.3420201433256649937, 0.000000000000000000 ) ) ;
#11924=ORIENTED_EDGE ( 'NONE', *, *, #9820, .T. ) ;
#11930=CARTESIAN_POINT ( 'NONE',  ( -71.24615306438097662, 62.51920506522922949, -167.1454815528550739 ) ) ;
#11931=CARTESIAN_POINT ( 'NONE',  ( -68.99615306438084872, 93.11619853813030545, -15.00000000000001421 ) ) ;
#11932=ORIENTED_EDGE ( 'NONE', *, *, #13860, .F. ) ;
#11935=AXIS2_PLACEMENT_3D ( 'NONE', #10233, #7076, #17166 ) ;
#11938=VERTEX_POINT ( 'NONE', #17996 ) ;
#11941=PLANE ( 'NONE',  #10614 ) ;
#11942=DIRECTION ( 'NONE',  ( 0.000000000000000000, 1.000000000000000000, 0.000000000000000000 ) ) ;
#11943=DIRECTION ( 'NONE',  ( 0.9396926207859084279, 0.3420201433256686574, 0.000000000000000000 ) ) ;
#11946=PLANE ( 'NONE',  #13927 ) ;
#11952=CARTESIAN_POINT ( 'NONE',  ( -68.99615306438072082, 133.9569029881302811, -15.00000000000001421 ) ) ;
#11955=VECTOR ( 'NONE', #16831, 1000.000000000000000 ) ;
#11956=VERTEX_POINT ( 'NONE', #5078 ) ;
#11958=EDGE_CURVE ( 'NONE', #13900, #16082, #5278, .T. ) ;
#11959=ORIENTED_EDGE ( 'NONE', *, *, #18323, .T. ) ;
#11964=AXIS2_PLACEMENT_3D ( 'NONE', #9925, #2822, #5792 ) ;
#11966=DIRECTION ( 'NONE',  ( -0.9396926207858995461, 0.3420201433256928603, 0.000000000000000000 ) ) ;
#11968=LINE ( 'NONE', #17666, #3141 ) ;
#11972=DIRECTION ( 'NONE',  ( 0.000000000000000000, 0.000000000000000000, 1.000000000000000000 ) ) ;
#11978=CARTESIAN_POINT ( 'NONE',  ( -71.24615306438114715, 13.14259340456377956, -15.00000000000001421 ) ) ;
#11979=VERTEX_POINT ( 'NONE', #4902 ) ;
#11986=LINE ( 'NONE', #3283, #10572 ) ;
#11989=VECTOR ( 'NONE', #383, 1000.000000000000000 ) ;
#11998=VECTOR ( 'NONE', #6225, 1000.000000000000000 ) ;
#12001=LINE ( 'NONE', #16300, #4006 ) ;
#12003=EDGE_CURVE ( 'NONE', #13170, #16976, #10798, .T. ) ;
#12008=VECTOR ( 'NONE', #16618, 1000.000000000000000 ) ;
#12017=ADVANCED_FACE ( 'NONE', ( #2098 ), #14998, .T. ) ;
#12018=CARTESIAN_POINT ( 'NONE',  ( -68.99615306438089135, 86.83301323813024908, -167.1454815528550739 ) ) ;
#12019=CARTESIAN_POINT ( 'NONE',  ( -68.99615306438072082, 140.2400882881302948, -167.1454815528550739 ) ) ;
#12021=VECTOR ( 'NONE', #5275, 1000.000000000000000 ) ;
#12024=ORIENTED_EDGE ( 'NONE', *, *, #13161, .F. ) ;
#12025=CARTESIAN_POINT ( 'NONE',  ( -68.99615306438094819, 54.80223088166269463, 15.00000000000006928 ) ) ;
#12027=EDGE_CURVE ( 'NONE', #1519, #17396, #13518, .T. ) ;
#12033=ADVANCED_FACE ( 'NONE', ( #13613 ), #6391, .T. ) ;
#12036=VECTOR ( 'NONE', #772, 1000.000000000000000 ) ;
#12037=ORIENTED_EDGE ( 'NONE', *, *, #5247, .F. ) ;
#12038=FACE_OUTER_BOUND ( 'NONE', #15208, .T. ) ;
#12039=FACE_OUTER_BOUND ( 'NONE', #6526, .T. ) ;
#12040=VERTEX_POINT ( 'NONE', #13899 ) ;
#12053=AXIS2_PLACEMENT_3D ( 'NONE', #6706, #6602, #18125 ) ;
#12054=LINE ( 'NONE', #9517, #15062 ) ;
#12056=VERTEX_POINT ( 'NONE', #11371 ) ;
#12061=ORIENTED_EDGE ( 'NONE', *, *, #3106, .T. ) ;
#12062=VECTOR ( 'NONE', #4920, 1000.000000000000227 ) ;
#12063=VERTEX_POINT ( 'NONE', #12498 ) ;
#12065=VERTEX_POINT ( 'NONE', #17157 ) ;
#12068=PLANE ( 'NONE',  #12127 ) ;
#12070=VECTOR ( 'NONE', #5600, 1000.000000000000000 ) ;
#12079=LINE ( 'NONE', #10476, #2090 ) ;
#12080=ORIENTED_EDGE ( 'NONE', *, *, #17376, .T. ) ;
#12084=LINE ( 'NONE', #3551, #13707 ) ;
#12085=ORIENTED_EDGE ( 'NONE', *, *, #18329, .T. ) ;
#12086=VECTOR ( 'NONE', #1686, 1000.000000000000000 ) ;
#12087=ORIENTED_EDGE ( 'NONE', *, *, #5048, .T. ) ;
#12089=CARTESIAN_POINT ( 'NONE',  ( -71.24615306438091977, 79.11603905456372843, -167.1454815528550739 ) ) ;
#12090=CARTESIAN_POINT ( 'NONE',  ( -71.24615306438097662, 57.12489050456376560, 15.00000000000006928 ) ) ;
#12091=DIRECTION ( 'NONE',  ( 0.3420201433256686574, 0.9396926207859084279, -0.000000000000000000 ) ) ;
#12093=VERTEX_POINT ( 'NONE', #5648 ) ;
#12097=VECTOR ( 'NONE', #10352, 1000.000000000000000 ) ;
#12103=ORIENTED_EDGE ( 'NONE', *, *, #366, .F. ) ;
#12104=VECTOR ( 'NONE', #2324, 1000.000000000000000 ) ;
#12105=DIRECTION ( 'NONE',  ( 0.000000000000000000, 0.000000000000000000, -1.000000000000000000 ) ) ;
#12106=ORIENTED_EDGE ( 'NONE', *, *, #3204, .F. ) ;
#12111=VECTOR ( 'NONE', #3930, 1000.000000000000114 ) ;
#12112=VECTOR ( 'NONE', #5108, 1000.000000000000114 ) ;
#12116=ORIENTED_EDGE ( 'NONE', *, *, #3795, .T. ) ;
#12117=CARTESIAN_POINT ( 'NONE',  ( -71.24615306438114715, 9.112130015229229940, -15.00000000000001421 ) ) ;
#12119=CARTESIAN_POINT ( 'NONE',  ( -68.99615306438080609, 108.8241617881302545, -167.1454815528550739 ) ) ;
#12121=EDGE_CURVE ( 'NONE', #409, #8399, #14270, .T. ) ;
#12123=VERTEX_POINT ( 'NONE', #11282 ) ;
#12124=DIRECTION ( 'NONE',  ( -0.9396926207859093161, 0.3420201433256661039, -4.890320548438453836E-16 ) ) ;
#12127=AXIS2_PLACEMENT_3D ( 'NONE', #8985, #13371, #8895 ) ;
#12129=CARTESIAN_POINT ( 'NONE',  ( -68.99615306438077766, 117.6340838816626899, -15.00000000000001421 ) ) ;
#12130=ADVANCED_FACE ( 'NONE', ( #15671 ), #8564, .T. ) ;
#12132=DIRECTION ( 'NONE',  ( 0.000000000000000000, 0.000000000000000000, -1.000000000000000000 ) ) ;
#12136=DIRECTION ( 'NONE',  ( 0.3420201433256481738, 0.9396926207859158664, -0.000000000000000000 ) ) ;
#12138=ORIENTED_EDGE ( 'NONE', *, *, #12927, .F. ) ;
#12144=VERTEX_POINT ( 'NONE', #5741 ) ;
#12145=CARTESIAN_POINT ( 'NONE',  ( -68.99615306438094819, 51.66063823166267355, 15.00000000000006928 ) ) ;
#12153=DIRECTION ( 'NONE',  ( 0.000000000000000000, 1.000000000000000000, 0.000000000000000000 ) ) ;
#12163=LINE ( 'NONE', #7947, #15325 ) ;
#12165=CARTESIAN_POINT ( 'NONE',  ( -68.99615306438089135, 86.83301323813024908, -167.1454815528550739 ) ) ;
#12171=EDGE_LOOP ( 'NONE', ( #11003, #10143, #15873, #9869 ) ) ;
#12176=VERTEX_POINT ( 'NONE', #18192 ) ;
#12177=DIRECTION ( 'NONE',  ( 0.9396926207859093161, 0.3420201433256663814, 4.890320548438453836E-16 ) ) ;
#12184=ORIENTED_EDGE ( 'NONE', *, *, #5402, .F. ) ;
#12186=DIRECTION ( 'NONE',  ( -1.000000000000000000, 0.000000000000000000, 1.156482317317869999E-16 ) ) ;
#12191=ORIENTED_EDGE ( 'NONE', *, *, #7885, .F. ) ;
#12192=DIRECTION ( 'NONE',  ( -0.9396926207859069846, 0.3420201433256723766, 0.000000000000000000 ) ) ;
#12194=EDGE_CURVE ( 'NONE', #12144, #16133, #1264, .T. ) ;
#12196=CARTESIAN_POINT ( 'NONE',  ( -71.24615306438080609, 106.5015021652292404, -167.1454815528550739 ) ) ;
#12199=VERTEX_POINT ( 'NONE', #9868 ) ;
#12201=DIRECTION ( 'NONE',  ( -0.9396926207859084279, 0.3420201433256686574, 0.000000000000000000 ) ) ;
#12202=ORIENTED_EDGE ( 'NONE', *, *, #15561, .T. ) ;
#12207=LINE ( 'NONE', #12025, #11132 ) ;
#12216=DIRECTION ( 'NONE',  ( 1.000000000000000000, 0.000000000000000000, 0.000000000000000000 ) ) ;
#12217=VERTEX_POINT ( 'NONE', #18477 ) ;
#12225=EDGE_CURVE ( 'NONE', #16358, #18030, #17488, .T. ) ;
#12227=CARTESIAN_POINT ( 'NONE',  ( -71.24615306438086293, 88.54081700456373483, -167.1454815528550739 ) ) ;
#12228=EDGE_CURVE ( 'NONE', #14842, #7034, #652, .T. ) ;
#12229=LINE ( 'NONE', #10934, #6950 ) ;
#12230=ORIENTED_EDGE ( 'NONE', *, *, #12608, .T. ) ;
#12232=DIRECTION ( 'NONE',  ( -0.9396926207859171987, 0.3420201433256444545, 0.000000000000000000 ) ) ;
#12233=ORIENTED_EDGE ( 'NONE', *, *, #12953, .T. ) ;
#12235=EDGE_CURVE ( 'NONE', #15896, #6911, #14680, .T. ) ;
#12239=ORIENTED_EDGE ( 'NONE', *, *, #1838, .F. ) ;
#12242=EDGE_CURVE ( 'NONE', #797, #11558, #6446, .T. ) ;
#12244=ORIENTED_EDGE ( 'NONE', *, *, #11893, .F. ) ;
#12246=DIRECTION ( 'NONE',  ( 0.3420201433256686574, -0.9396926207859084279, 0.000000000000000000 ) ) ;
#12247=CARTESIAN_POINT ( 'NONE',  ( -68.99615306438100504, 45.37745293166267402, -15.00000000000001421 ) ) ;
#12248=EDGE_CURVE ( 'NONE', #13617, #16048, #6342, .T. ) ;
#12254=CARTESIAN_POINT ( 'NONE',  ( -68.99615306438106188, 24.00116023813026445, 15.00000000000006928 ) ) ;
#12255=ORIENTED_EDGE ( 'NONE', *, *, #5822, .F. ) ;
#12257=EDGE_CURVE ( 'NONE', #9827, #6461, #14860, .T. ) ;
#12259=AXIS2_PLACEMENT_3D ( 'NONE', #280, #6151, #7581 ) ;
#12261=DIRECTION ( 'NONE',  ( 0.000000000000000000, 1.000000000000000000, 0.000000000000000000 ) ) ;
#12263=CARTESIAN_POINT ( 'NONE',  ( -68.99615306438100504, 45.37745293166267402, 15.00000000000006928 ) ) ;
#12265=ORIENTED_EDGE ( 'NONE', *, *, #7560, .F. ) ;
#12266=EDGE_LOOP ( 'NONE', ( #12499, #16307, #16958, #10146 ) ) ;
#12267=VECTOR ( 'NONE', #12636, 1000.000000000000000 ) ;
#12274=CARTESIAN_POINT ( 'NONE',  ( -71.24615306438109030, 31.99214930456376038, 15.00000000000006928 ) ) ;
#12275=LINE ( 'NONE', #13768, #4549 ) ;
#12276=CARTESIAN_POINT ( 'NONE',  ( -68.99615306438099083, 30.28434553813024621, 15.00000000000006928 ) ) ;
#12277=LINE ( 'NONE', #9463, #8760 ) ;
#12279=DIRECTION ( 'NONE',  ( 1.000000000000000000, 0.000000000000000000, 0.000000000000000000 ) ) ;
#12281=PLANE ( 'NONE',  #18279 ) ;
#12282=DIRECTION ( 'NONE',  ( 0.000000000000000000, 0.000000000000000000, 1.000000000000000000 ) ) ;
#12283=LINE ( 'NONE', #16571, #12999 ) ;
#12288=CARTESIAN_POINT ( 'NONE',  ( -71.24615306438083451, 97.07672421522921979, -15.00000000000001421 ) ) ;
#12290=AXIS2_PLACEMENT_3D ( 'NONE', #15394, #15577, #15482 ) ;
#12291=VECTOR ( 'NONE', #6016, 1000.000000000000000 ) ;
#12292=PLANE ( 'NONE',  #9817 ) ;
#12293=ORIENTED_EDGE ( 'NONE', *, *, #12194, .F. ) ;
#12297=CARTESIAN_POINT ( 'NONE',  ( -71.24615306438091977, 75.08557566522922855, -15.00000000000001421 ) ) ;
#12301=VECTOR ( 'NONE', #5976, 1000.000000000000000 ) ;
#12307=CARTESIAN_POINT ( 'NONE',  ( -68.99615306438118978, -1.131580961869738999, -15.00000000000001421 ) ) ;
#12312=ORIENTED_EDGE ( 'NONE', *, *, #9977, .F. ) ;
#12314=CARTESIAN_POINT ( 'NONE',  ( -68.99615306438072082, 127.0588618316627105, 15.00000000000006928 ) ) ;
#12315=EDGE_CURVE ( 'NONE', #17731, #15948, #1971, .T. ) ;
#12328=CARTESIAN_POINT ( 'NONE',  ( -71.24615306438117557, 2.828944715229236628, -15.00000000000001421 ) ) ;
#12330=CARTESIAN_POINT ( 'NONE',  ( -68.99615306438110451, 8.293196988130269176, -15.00000000000001421 ) ) ;
#12332=AXIS2_PLACEMENT_3D ( 'NONE', #14274, #3970, #6785 ) ;
#12334=DIRECTION ( 'NONE',  ( 0.000000000000000000, 0.000000000000000000, 1.000000000000000000 ) ) ;
#12339=PLANE ( 'NONE',  #10185 ) ;
#12340=ORIENTED_EDGE ( 'NONE', *, *, #12228, .T. ) ;
#12342=LINE ( 'NONE', #7838, #8065 ) ;
#12346=EDGE_CURVE ( 'NONE', #16349, #3860, #11968, .T. ) ;
#12349=CARTESIAN_POINT ( 'NONE',  ( -71.24615306438070661, 187.7866419848965052, -167.1454815528550739 ) ) ;
#12352=CARTESIAN_POINT ( 'NONE',  ( -68.99615306438072082, 127.0588618316627105, 15.00000000000006928 ) ) ;
#12357=LINE ( 'NONE', #11039, #15621 ) ;
#12359=EDGE_CURVE ( 'NONE', #9812, #7225, #3541, .T. ) ;
#12361=PLANE ( 'NONE',  #12363 ) ;
#12363=AXIS2_PLACEMENT_3D ( 'NONE', #18054, #940, #11042 ) ;
#12366=VERTEX_POINT ( 'NONE', #14037 ) ;
#12367=DIRECTION ( 'NONE',  ( 0.9396926207859185309, 0.3420201433256406798, 0.000000000000000000 ) ) ;
#12370=ORIENTED_EDGE ( 'NONE', *, *, #10358, .F. ) ;
#12373=EDGE_CURVE ( 'NONE', #13368, #14342, #3744, .T. ) ;
#12374=ORIENTED_EDGE ( 'NONE', *, *, #13367, .T. ) ;
#12380=CARTESIAN_POINT ( 'NONE',  ( -68.99615306438089135, 83.69142058813029905, -167.1454815528550739 ) ) ;
#12382=LINE ( 'NONE', #1064, #5369 ) ;
#12384=ORIENTED_EDGE ( 'NONE', *, *, #10508, .F. ) ;
#12385=CARTESIAN_POINT ( 'NONE',  ( -68.99615306438100504, 39.70912348813028103, 15.00000000000006928 ) ) ;
#12388=ORIENTED_EDGE ( 'NONE', *, *, #7891, .F. ) ;
#12390=ADVANCED_FACE ( 'NONE', ( #11038 ), #6634, .T. ) ;
#12393=ORIENTED_EDGE ( 'NONE', *, *, #4688, .T. ) ;
#12394=VECTOR ( 'NONE', #4369, 1000.000000000000000 ) ;
#12395=CARTESIAN_POINT ( 'NONE',  ( -71.24615306438097662, 62.51920506522922949, 15.00000000000006928 ) ) ;
#12397=ORIENTED_EDGE ( 'NONE', *, *, #2640, .T. ) ;
#12398=EDGE_CURVE ( 'NONE', #10161, #14281, #17947, .T. ) ;
#12399=ORIENTED_EDGE ( 'NONE', *, *, #1955, .F. ) ;
#12400=DIRECTION ( 'NONE',  ( 0.9396926207859097602, 0.3420201433256649937, -1.086737899652991371E-16 ) ) ;
#12401=DIRECTION ( 'NONE',  ( 0.9396926207859171987, 0.3420201433256444545, 0.000000000000000000 ) ) ;
#12403=VECTOR ( 'NONE', #2609, 1000.000000000000000 ) ;
#12404=ORIENTED_EDGE ( 'NONE', *, *, #1475, .T. ) ;
#12408=LINE ( 'NONE', #6966, #14962 ) ;
#12410=EDGE_LOOP ( 'NONE', ( #14135, #2165, #9536, #12881 ) ) ;
#12412=DIRECTION ( 'NONE',  ( -0.9396926207859158664, 0.3420201433256481738, 1.086737899652998397E-16 ) ) ;
#12413=CARTESIAN_POINT ( 'NONE',  ( -68.99615306438072082, 130.2004544816626890, 15.00000000000006928 ) ) ;
#12417=VERTEX_POINT ( 'NONE', #8235 ) ;
#12422=ORIENTED_EDGE ( 'NONE', *, *, #4359, .T. ) ;
#12423=AXIS2_PLACEMENT_3D ( 'NONE', #9921, #17435, #14493 ) ;
#12425=DIRECTION ( 'NONE',  ( -0.9396926207859088720, 0.3420201433256675472, 0.000000000000000000 ) ) ;
#12426=CARTESIAN_POINT ( 'NONE',  ( -71.24615306438091977, 71.94398301522919326, 15.00000000000006928 ) ) ;
#12431=CARTESIAN_POINT ( 'NONE',  ( -68.99615306438072082, 127.6737176881302958, 15.00000000000006928 ) ) ;
#12432=VERTEX_POINT ( 'NONE', #1219 ) ;
#12434=DIRECTION ( 'NONE',  ( 0.000000000000000000, 0.000000000000000000, 1.000000000000000000 ) ) ;
#12437=PLANE ( 'NONE',  #10041 ) ;
#12439=LINE ( 'NONE', #15312, #2434 ) ;
#12448=EDGE_LOOP ( 'NONE', ( #6205, #3162, #10218, #16219 ) ) ;
#12449=FACE_OUTER_BOUND ( 'NONE', #2357, .T. ) ;
#12450=ORIENTED_EDGE ( 'NONE', *, *, #7035, .F. ) ;
#12452=FACE_OUTER_BOUND ( 'NONE', #15300, .T. ) ;
#12456=LINE ( 'NONE', #15524, #17384 ) ;
#12471=CARTESIAN_POINT ( 'NONE',  ( -71.24615306438089135, 82.25763170456374951, 15.00000000000006928 ) ) ;
#12474=CARTESIAN_POINT ( 'NONE',  ( -71.24615306438100504, 53.09442711522921599, -167.1454815528550739 ) ) ;
#12479=LINE ( 'NONE', #1150, #5111 ) ;
#12494=FACE_OUTER_BOUND ( 'NONE', #1221, .T. ) ;
#12495=LINE ( 'NONE', #14074, #9035 ) ;
#12498=CARTESIAN_POINT ( 'NONE',  ( -71.24615306438091977, 75.08557566522922855, 15.00000000000006928 ) ) ;
#12499=ORIENTED_EDGE ( 'NONE', *, *, #7019, .F. ) ;
#12503=EDGE_CURVE ( 'NONE', #18002, #4483, #4208, .T. ) ;
#12504=CARTESIAN_POINT ( 'NONE',  ( -71.24615306438086293, 90.79353891522923448, -167.1454815528550739 ) ) ;
#12508=ORIENTED_EDGE ( 'NONE', *, *, #8928, .F. ) ;
#12509=CARTESIAN_POINT ( 'NONE',  ( -71.24615306438111872, 21.67850061522927518, -15.00000000000001421 ) ) ;
#12510=CARTESIAN_POINT ( 'NONE',  ( -71.24615306438070661, 137.9174286652292096, 15.00000000000006928 ) ) ;
#12516=FACE_OUTER_BOUND ( 'NONE', #14708, .T. ) ;
#12519=DIRECTION ( 'NONE',  ( 0.9396926207859158664, 0.3420201433256481738, 0.000000000000000000 ) ) ;
#12521=CARTESIAN_POINT ( 'NONE',  ( -68.99615306438100504, 39.09426763166271002, -15.00000000000001421 ) ) ;
#12523=CARTESIAN_POINT ( 'NONE',  ( -68.99615306438120399, -1.131580961869733448, -167.1454815528550739 ) ) ;
#12526=VECTOR ( 'NONE', #15810, 1000.000000000000000 ) ;
#12528=DIRECTION ( 'NONE',  ( 0.9396926207859097602, 0.3420201433256649937, 0.000000000000000000 ) ) ;
#12530=LINE ( 'NONE', #11225, #17789 ) ;
#12531=FACE_OUTER_BOUND ( 'NONE', #13740, .T. ) ;
#12532=PLANE ( 'NONE',  #13458 ) ;
#12541=EDGE_LOOP ( 'NONE', ( #7055, #8659, #10835, #7037 ) ) ;
#12543=CARTESIAN_POINT ( 'NONE',  ( -71.24615306438086293, 93.93513156522925556, -15.00000000000001421 ) ) ;
#12547=CARTESIAN_POINT ( 'NONE',  ( -71.24615306438114715, 9.112130015229229940, -15.00000000000001421 ) ) ;
#12551=DIRECTION ( 'NONE',  ( 0.000000000000000000, 1.000000000000000000, 0.000000000000000000 ) ) ;
#12556=ORIENTED_EDGE ( 'NONE', *, *, #10319, .T. ) ;
#12559=VECTOR ( 'NONE', #15083, 1000.000000000000000 ) ;
#12560=DIRECTION ( 'NONE',  ( -0.9396926207859084279, 0.3420201433256687684, -4.890320548438449892E-16 ) ) ;
#12561=LINE ( 'NONE', #10966, #3674 ) ;
#12563=VECTOR ( 'NONE', #17132, 1000.000000000000000 ) ;
#12564=LINE ( 'NONE', #9761, #950 ) ;
#12570=DIRECTION ( 'NONE',  ( 0.9396926207859171987, 0.3420201433256444545, 0.000000000000000000 ) ) ;
#12572=ORIENTED_EDGE ( 'NONE', *, *, #5835, .F. ) ;
#12573=DIRECTION ( 'NONE',  ( 0.000000000000000000, 0.000000000000000000, 1.000000000000000000 ) ) ;
#12574=ORIENTED_EDGE ( 'NONE', *, *, #17850, .T. ) ;
#12575=VECTOR ( 'NONE', #7564, 1000.000000000000114 ) ;
#12583=DIRECTION ( 'NONE',  ( -0.9396926207859069846, 0.3420201433256723766, 1.086737899652988166E-16 ) ) ;
#12584=ORIENTED_EDGE ( 'NONE', *, *, #15356, .F. ) ;
#12587=ORIENTED_EDGE ( 'NONE', *, *, #3664, .T. ) ;
#12588=LINE ( 'NONE', #11281, #4799 ) ;
#12592=LINE ( 'NONE', #16881, #18269 ) ;
#12593=PLANE ( 'NONE',  #14961 ) ;
#12594=DIRECTION ( 'NONE',  ( 1.000000000000000000, 0.000000000000000000, 0.000000000000000000 ) ) ;
#12597=ORIENTED_EDGE ( 'NONE', *, *, #1721, .T. ) ;
#12599=CARTESIAN_POINT ( 'NONE',  ( -71.24615306438086293, 93.93513156522925556, -167.1454815528550739 ) ) ;
#12601=ORIENTED_EDGE ( 'NONE', *, *, #3135, .F. ) ;
#12603=DIRECTION ( 'NONE',  ( 0.000000000000000000, 0.000000000000000000, 1.000000000000000000 ) ) ;
#12606=VERTEX_POINT ( 'NONE', #14574 ) ;
#12608=EDGE_CURVE ( 'NONE', #593, #11376, #6223, .T. ) ;
#12615=VERTEX_POINT ( 'NONE', #7831 ) ;
#12619=DIRECTION ( 'NONE',  ( 1.000000000000000000, 0.000000000000000000, 0.000000000000000000 ) ) ;
#12620=CARTESIAN_POINT ( 'NONE',  ( -68.99615306438106188, 35.95267498166268894, -15.00000000000001421 ) ) ;
#12623=VECTOR ( 'NONE', #18265, 1000.000000000000000 ) ;
#12628=ORIENTED_EDGE ( 'NONE', *, *, #5806, .T. ) ;
#12630=VECTOR ( 'NONE', #8052, 1000.000000000000000 ) ;
#12632=LINE ( 'NONE', #1204, #10311 ) ;
#12634=EDGE_CURVE ( 'NONE', #13327, #12063, #16058, .T. ) ;
#12636=DIRECTION ( 'NONE',  ( 0.000000000000000000, 0.000000000000000000, 1.000000000000000000 ) ) ;
#12638=ORIENTED_EDGE ( 'NONE', *, *, #4199, .F. ) ;
#12639=VECTOR ( 'NONE', #9121, 1000.000000000000000 ) ;
#12640=DIRECTION ( 'NONE',  ( 0.9396926207859078728, 0.3420201433256701007, -1.086737899652989152E-16 ) ) ;
#12641=VERTEX_POINT ( 'NONE', #3519 ) ;
#12644=CARTESIAN_POINT ( 'NONE',  ( -68.99615306438103346, 33.42593818813029571, -15.00000000000001421 ) ) ;
#12647=ORIENTED_EDGE ( 'NONE', *, *, #3398, .F. ) ;
#12655=ORIENTED_EDGE ( 'NONE', *, *, #2972, .F. ) ;
#12656=AXIS2_PLACEMENT_3D ( 'NONE', #12089, #568, #16286 ) ;
#12659=PLANE ( 'NONE',  #5027 ) ;
#12662=ORIENTED_EDGE ( 'NONE', *, *, #10666, .F. ) ;
#12663=VECTOR ( 'NONE', #4553, 1000.000000000000000 ) ;
#12667=EDGE_CURVE ( 'NONE', #11154, #12950, #10550, .T. ) ;
#12668=VECTOR ( 'NONE', #5229, 1000.000000000000000 ) ;
#12670=VECTOR ( 'NONE', #10210, 1000.000000000000000 ) ;
#12672=CARTESIAN_POINT ( 'NONE',  ( -68.99615306438086293, 92.50134268166266338, -167.1454815528550739 ) ) ;
#12674=DIRECTION ( 'NONE',  ( 0.000000000000000000, 0.000000000000000000, 1.000000000000000000 ) ) ;
#12675=ORIENTED_EDGE ( 'NONE', *, *, #1800, .F. ) ;
#12677=CARTESIAN_POINT ( 'NONE',  ( -68.99615306438120399, -1.131580961869733448, -15.00000000000001421 ) ) ;
#12687=CARTESIAN_POINT ( 'NONE',  ( -68.99615306438117557, 5.151604338130305827, -167.1454815528550739 ) ) ;
#12690=CARTESIAN_POINT ( 'NONE',  ( -68.99615306438100504, 49.13390143813029454, -15.00000000000001421 ) ) ;
#12691=CARTESIAN_POINT ( 'NONE',  ( -68.99615306438087714, 83.69142058813029905, -15.00000000000001421 ) ) ;
#12695=DIRECTION ( 'NONE',  ( 1.000000000000000000, 0.000000000000000000, 0.000000000000000000 ) ) ;
#12701=EDGE_LOOP ( 'NONE', ( #10036, #11632, #6471, #15788 ) ) ;
#12703=FACE_OUTER_BOUND ( 'NONE', #6175, .T. ) ;
#12704=AXIS2_PLACEMENT_3D ( 'NONE', #4893, #10615, #16305 ) ;
#12707=VECTOR ( 'NONE', #13450, 1000.000000000000000 ) ;
#12709=VECTOR ( 'NONE', #5, 1000.000000000000000 ) ;
#12713=LINE ( 'NONE', #5574, #1328 ) ;
#12715=ORIENTED_EDGE ( 'NONE', *, *, #3907, .F. ) ;
#12717=DIRECTION ( 'NONE',  ( 0.000000000000000000, 1.000000000000000000, 0.000000000000000000 ) ) ;
#12722=DIRECTION ( 'NONE',  ( 0.9396926207859158664, 0.3420201433256481738, -1.086737899652998397E-16 ) ) ;
#12723=DIRECTION ( 'NONE',  ( 0.000000000000000000, 1.000000000000000000, 0.000000000000000000 ) ) ;
#12725=DIRECTION ( 'NONE',  ( 0.3420201433256724322, 0.9396926207859070956, -0.000000000000000000 ) ) ;
#12729=VECTOR ( 'NONE', #754, 1000.000000000000000 ) ;
#12731=CARTESIAN_POINT ( 'NONE',  ( -68.99615306438100504, 48.51904558166270220, -15.00000000000001421 ) ) ;
#12732=CARTESIAN_POINT ( 'NONE',  ( -68.99615306438072082, 139.6252324316626812, -167.1454815528550739 ) ) ;
#12734=DIRECTION ( 'NONE',  ( 0.000000000000000000, 1.000000000000000000, 0.000000000000000000 ) ) ;
#12735=ORIENTED_EDGE ( 'NONE', *, *, #9610, .F. ) ;
#12738=EDGE_CURVE ( 'NONE', #4587, #14830, #2605, .T. ) ;
#12740=VECTOR ( 'NONE', #12603, 1000.000000000000000 ) ;
#12743=ADVANCED_FACE ( 'NONE', ( #733 ), #18027, .T. ) ;
#12747=EDGE_CURVE ( 'NONE', #8708, #5168, #11118, .T. ) ;
#12749=VERTEX_POINT ( 'NONE', #6608 ) ;
#12750=CARTESIAN_POINT ( 'NONE',  ( -71.24615306438103346, 43.66964916522919538, -15.00000000000001421 ) ) ;
#12751=CARTESIAN_POINT ( 'NONE',  ( -71.24615306438091977, 79.11603905456372843, 15.00000000000006928 ) ) ;
#12753=ORIENTED_EDGE ( 'NONE', *, *, #9174, .T. ) ;
#12754=ADVANCED_FACE ( 'NONE', ( #6805 ), #12437, .T. ) ;
#12755=LINE ( 'NONE', #14040, #2406 ) ;
#12756=ORIENTED_EDGE ( 'NONE', *, *, #17315, .F. ) ;
#12757=LINE ( 'NONE', #101, #261 ) ;
#12765=DIRECTION ( 'NONE',  ( 1.000000000000000000, 0.000000000000000000, 0.000000000000000000 ) ) ;
#12768=ORIENTED_EDGE ( 'NONE', *, *, #14584, .F. ) ;
#12769=CARTESIAN_POINT ( 'NONE',  ( -68.99615306438091977, 77.40823528813029952, -15.00000000000001421 ) ) ;
#12773=ORIENTED_EDGE ( 'NONE', *, *, #18187, .F. ) ;
#12774=ORIENTED_EDGE ( 'NONE', *, *, #1271, .F. ) ;
#12778=ORIENTED_EDGE ( 'NONE', *, *, #10534, .F. ) ;
#12780=ORIENTED_EDGE ( 'NONE', *, *, #11100, .F. ) ;
#12784=LINE ( 'NONE', #4513, #7799 ) ;
#12787=ORIENTED_EDGE ( 'NONE', *, *, #11071, .F. ) ;
#12790=VERTEX_POINT ( 'NONE', #10931 ) ;
#12794=LINE ( 'NONE', #11297, #9676 ) ;
#12796=ORIENTED_EDGE ( 'NONE', *, *, #2784, .F. ) ;
#12800=CARTESIAN_POINT ( 'NONE',  ( -68.99615306438079188, 93.11619853813027703, 15.00000000000006928 ) ) ;
#12802=PLANE ( 'NONE',  #312 ) ;
#12803=LINE ( 'NONE', #5672, #11717 ) ;
#12804=CARTESIAN_POINT ( 'NONE',  ( -68.99615306438106188, 36.56753083813027416, -167.1454815528550739 ) ) ;
#12806=LINE ( 'NONE', #2798, #12403 ) ;
#12807=PLANE ( 'NONE',  #3595 ) ;
#12814=ADVANCED_FACE ( 'NONE', ( #6508 ), #3612, .T. ) ;
#12816=VECTOR ( 'NONE', #15469, 1000.000000000000000 ) ;
#12820=CARTESIAN_POINT ( 'NONE',  ( -71.24615306438103346, 44.55851990456372391, 15.00000000000006928 ) ) ;
#12826=DIRECTION ( 'NONE',  ( 0.000000000000000000, 0.000000000000000000, -1.000000000000000000 ) ) ;
#12829=EDGE_CURVE ( 'NONE', #10484, #9665, #8210, .T. ) ;
#12830=DIRECTION ( 'NONE',  ( -0.9396926207859084279, 0.3420201433256686574, 1.086737899652989892E-16 ) ) ;
#12832=CARTESIAN_POINT ( 'NONE',  ( -71.24615306438117557, 2.828944715229236628, -167.1454815528550739 ) ) ;
#12834=VECTOR ( 'NONE', #10675, 1000.000000000000000 ) ;
#12836=VERTEX_POINT ( 'NONE', #6713 ) ;
#12841=CARTESIAN_POINT ( 'NONE',  ( -71.24615306438076345, 126.2399288045637462, -167.1454815528550739 ) ) ;
#12843=LINE ( 'NONE', #9936, #9540 ) ;
#12844=ADVANCED_FACE ( 'NONE', ( #17391 ), #9253, .T. ) ;
#12845=LINE ( 'NONE', #10, #1501 ) ;
#12854=ORIENTED_EDGE ( 'NONE', *, *, #4863, .F. ) ;
#12856=EDGE_CURVE ( 'NONE', #3722, #8797, #14858, .T. ) ;
#12863=CARTESIAN_POINT ( 'NONE',  ( -68.99615306438076345, 102.5409764881302408, 15.00000000000006928 ) ) ;
#12869=LINE ( 'NONE', #8647, #10478 ) ;
#12877=ORIENTED_EDGE ( 'NONE', *, *, #10100, .F. ) ;
#12881=ORIENTED_EDGE ( 'NONE', *, *, #17516, .F. ) ;
#12885=DIRECTION ( 'NONE',  ( 0.000000000000000000, 1.000000000000000000, 0.000000000000000000 ) ) ;
#12893=EDGE_LOOP ( 'NONE', ( #8076, #2074, #3268, #12662 ) ) ;
#12894=EDGE_CURVE ( 'NONE', #13601, #18188, #14944, .T. ) ;
#12895=PLANE ( 'NONE',  #13782 ) ;
#12896=DIRECTION ( 'NONE',  ( 1.000000000000000000, 0.000000000000000000, 0.000000000000000000 ) ) ;
#12900=AXIS2_PLACEMENT_3D ( 'NONE', #4609, #2079, #1989 ) ;
#12910=VECTOR ( 'NONE', #2561, 1000.000000000000000 ) ;
#12911=ORIENTED_EDGE ( 'NONE', *, *, #13961, .T. ) ;
#12913=LINE ( 'NONE', #6755, #14146 ) ;
#12914=LINE ( 'NONE', #15519, #12070 ) ;
#12919=DIRECTION ( 'NONE',  ( 0.000000000000000000, 0.000000000000000000, -1.000000000000000000 ) ) ;
#12921=LINE ( 'NONE', #18443, #16787 ) ;
#12922=ORIENTED_EDGE ( 'NONE', *, *, #7340, .T. ) ;
#12927=EDGE_CURVE ( 'NONE', #10943, #12790, #14774, .T. ) ;
#12929=DIRECTION ( 'NONE',  ( 0.000000000000000000, 1.000000000000000000, 0.000000000000000000 ) ) ;
#12930=ORIENTED_EDGE ( 'NONE', *, *, #4913, .F. ) ;
#12932=VERTEX_POINT ( 'NONE', #3264 ) ;
#12936=LINE ( 'NONE', #107, #17120 ) ;
#12937=EDGE_CURVE ( 'NONE', #5348, #17556, #1772, .T. ) ;
#12939=EDGE_CURVE ( 'NONE', #689, #2737, #15998, .T. ) ;
#12942=PLANE ( 'NONE',  #15593 ) ;
#12943=ORIENTED_EDGE ( 'NONE', *, *, #4458, .F. ) ;
#12949=DIRECTION ( 'NONE',  ( 0.9396926207859171987, 0.3420201433256444545, 0.000000000000000000 ) ) ;
#12950=VERTEX_POINT ( 'NONE', #13199 ) ;
#12952=ADVANCED_FACE ( 'NONE', ( #7480 ), #12068, .T. ) ;
#12953=EDGE_CURVE ( 'NONE', #5917, #10355, #6067, .T. ) ;
#12957=ADVANCED_FACE ( 'NONE', ( #14678 ), #7579, .T. ) ;
#12959=VECTOR ( 'NONE', #15745, 1000.000000000000000 ) ;
#12963=LINE ( 'NONE', #5992, #5450 ) ;
#12964=EDGE_LOOP ( 'NONE', ( #6722, #3522, #10491, #12191 ) ) ;
#12965=EDGE_CURVE ( 'NONE', #17050, #5068, #17769, .T. ) ;
#12968=VERTEX_POINT ( 'NONE', #15589 ) ;
#12969=AXIS2_PLACEMENT_3D ( 'NONE', #4179, #11490, #1465 ) ;
#12979=ORIENTED_EDGE ( 'NONE', *, *, #9394, .T. ) ;
#12980=ORIENTED_EDGE ( 'NONE', *, *, #15071, .F. ) ;
#12982=CARTESIAN_POINT ( 'NONE',  ( -71.24615306438079188, 91.68240965456378433, 15.00000000000006928 ) ) ;
#12987=VECTOR ( 'NONE', #13585, 1000.000000000000114 ) ;
#12988=CARTESIAN_POINT ( 'NONE',  ( -71.24615306438069240, 119.9567435045637893, 15.00000000000006928 ) ) ;
#12989=FACE_OUTER_BOUND ( 'NONE', #5331, .T. ) ;
#12992=CARTESIAN_POINT ( 'NONE',  ( -71.24615306438080609, 115.9262801152292042, 15.00000000000006928 ) ) ;
#12994=EDGE_LOOP ( 'NONE', ( #8206, #3736, #943, #13140 ) ) ;
#12998=CARTESIAN_POINT ( 'NONE',  ( -68.99615306438100504, 42.23586028166270978, 15.00000000000006928 ) ) ;
#12999=VECTOR ( 'NONE', #581, 1000.000000000000114 ) ;
#13000=VECTOR ( 'NONE', #4280, 1000.000000000000000 ) ;
#13001=ORIENTED_EDGE ( 'NONE', *, *, #5739, .F. ) ;
#13010=AXIS2_PLACEMENT_3D ( 'NONE', #11930, #17903, #887 ) ;
#13015=CARTESIAN_POINT ( 'NONE',  ( -71.24615306438070661, 135.6647067545637242, -167.1454815528550739 ) ) ;
#13016=ORIENTED_EDGE ( 'NONE', *, *, #3781, .F. ) ;
#13018=DIRECTION ( 'NONE',  ( 0.000000000000000000, 0.000000000000000000, 1.000000000000000000 ) ) ;
#13019=ORIENTED_EDGE ( 'NONE', *, *, #5948, .F. ) ;
#13021=CARTESIAN_POINT ( 'NONE',  ( -68.99615306438070661, 136.4836397816626743, 15.00000000000006928 ) ) ;
#13022=VERTEX_POINT ( 'NONE', #14279 ) ;
#13023=ORIENTED_EDGE ( 'NONE', *, *, #5293, .F. ) ;
#13024=AXIS2_PLACEMENT_3D ( 'NONE', #16083, #7402, #562 ) ;
#13029=CARTESIAN_POINT ( 'NONE',  ( -68.99615306438090556, 74.26664263813029265, -15.00000000000001421 ) ) ;
#13030=CARTESIAN_POINT ( 'NONE',  ( -68.99615306438072082, 130.8153103381302742, -167.1454815528550739 ) ) ;
#13031=EDGE_CURVE ( 'NONE', #13368, #17232, #6694, .T. ) ;
#13032=DIRECTION ( 'NONE',  ( 0.000000000000000000, 1.000000000000000000, 0.000000000000000000 ) ) ;
#13039=AXIS2_PLACEMENT_3D ( 'NONE', #15026, #16420, #17920 ) ;
#13040=LINE ( 'NONE', #5548, #13751 ) ;
#13041=VERTEX_POINT ( 'NONE', #14191 ) ;
#13042=DIRECTION ( 'NONE',  ( 0.000000000000000000, 0.000000000000000000, -1.000000000000000000 ) ) ;
#13044=VERTEX_POINT ( 'NONE', #12510 ) ;
#13045=EDGE_CURVE ( 'NONE', #6896, #1716, #14094, .T. ) ;
#13049=LINE ( 'NONE', #14264, #9688 ) ;
#13050=DIRECTION ( 'NONE',  ( 0.000000000000000000, 1.000000000000000000, 0.000000000000000000 ) ) ;
#13051=EDGE_CURVE ( 'NONE', #10924, #5018, #15294, .T. ) ;
#13063=EDGE_CURVE ( 'NONE', #10938, #13044, #2774, .T. ) ;
#13067=EDGE_CURVE ( 'NONE', #12093, #7210, #8574, .T. ) ;
#13068=ORIENTED_EDGE ( 'NONE', *, *, #9186, .T. ) ;
#13069=CARTESIAN_POINT ( 'NONE',  ( -68.99615306438117557, 4.536748481662661092, -167.1454815528550739 ) ) ;
#13071=EDGE_CURVE ( 'NONE', #12065, #6928, #18205, .T. ) ;
#13072=ORIENTED_EDGE ( 'NONE', *, *, #13267, .F. ) ;
#13074=DIRECTION ( 'NONE',  ( 0.9396926207859185309, 0.3420201433256406798, 4.890320548438501168E-16 ) ) ;
#13075=CARTESIAN_POINT ( 'NONE',  ( -71.24615306438114715, 9.112130015229229940, -167.1454815528550739 ) ) ;
#13077=CARTESIAN_POINT ( 'NONE',  ( -71.24615306438096241, 47.70011255456377341, 15.00000000000006928 ) ) ;
#13078=ORIENTED_EDGE ( 'NONE', *, *, #14855, .T. ) ;
#13081=ORIENTED_EDGE ( 'NONE', *, *, #17719, .T. ) ;
#13082=DIRECTION ( 'NONE',  ( 0.000000000000000000, 0.000000000000000000, 1.000000000000000000 ) ) ;
#13084=ORIENTED_EDGE ( 'NONE', *, *, #14579, .F. ) ;
#13086=EDGE_CURVE ( 'NONE', #11956, #14266, #5371, .T. ) ;
#13088=DIRECTION ( 'NONE',  ( 0.000000000000000000, 0.000000000000000000, -1.000000000000000000 ) ) ;
#13091=DIRECTION ( 'NONE',  ( 0.000000000000000000, 0.000000000000000000, -1.000000000000000000 ) ) ;
#13092=EDGE_LOOP ( 'NONE', ( #14031, #698, #694, #5796 ) ) ;
#13093=CARTESIAN_POINT ( 'NONE',  ( -71.24615306438070661, 147.3422066152292871, 15.00000000000006928 ) ) ;
#13102=EDGE_LOOP ( 'NONE', ( #8057, #10735, #4017, #17901 ) ) ;
#13105=ORIENTED_EDGE ( 'NONE', *, *, #5121, .F. ) ;
#13107=LINE ( 'NONE', #13029, #13235 ) ;
#13108=DIRECTION ( 'NONE',  ( 0.9396926207859097602, 0.3420201433256649381, 4.890320548438455808E-16 ) ) ;
#13109=DIRECTION ( 'NONE',  ( 0.000000000000000000, 0.000000000000000000, 1.000000000000000000 ) ) ;
#13114=CARTESIAN_POINT ( 'NONE',  ( -68.99615306438094819, 71.12504998813029999, 15.00000000000006928 ) ) ;
#13115=LINE ( 'NONE', #10850, #6978 ) ;
#13116=PLANE ( 'NONE',  #5069 ) ;
#13117=VECTOR ( 'NONE', #10759, 1000.000000000000000 ) ;
#13125=CARTESIAN_POINT ( 'NONE',  ( -71.24615306438094819, 68.80239036522922902, 15.00000000000006928 ) ) ;
#13126=CARTESIAN_POINT ( 'NONE',  ( -68.99615306438097662, 61.70027203813028649, -167.1454815528550739 ) ) ;
#13127=ORIENTED_EDGE ( 'NONE', *, *, #8889, .T. ) ;
#13130=CARTESIAN_POINT ( 'NONE',  ( -71.24615306438097662, 59.37761241522920841, 15.00000000000006928 ) ) ;
#13133=ORIENTED_EDGE ( 'NONE', *, *, #16152, .T. ) ;
#13134=CARTESIAN_POINT ( 'NONE',  ( -68.99615306438100504, 42.23586028166270978, -15.00000000000001421 ) ) ;
#13135=ORIENTED_EDGE ( 'NONE', *, *, #2974, .F. ) ;
#13136=ORIENTED_EDGE ( 'NONE', *, *, #14096, .F. ) ;
#13137=VECTOR ( 'NONE', #10336, 1000.000000000000000 ) ;
#13140=ORIENTED_EDGE ( 'NONE', *, *, #5617, .F. ) ;
#13142=DIRECTION ( 'NONE',  ( 0.000000000000000000, 0.000000000000000000, 1.000000000000000000 ) ) ;
#13143=VERTEX_POINT ( 'NONE', #8656 ) ;
#13145=DIRECTION ( 'NONE',  ( 1.000000000000000000, 0.000000000000000000, 0.000000000000000000 ) ) ;
#13153=FACE_OUTER_BOUND ( 'NONE', #14071, .T. ) ;
#13156=DIRECTION ( 'NONE',  ( 0.000000000000000000, 0.000000000000000000, 1.000000000000000000 ) ) ;
#13157=ORIENTED_EDGE ( 'NONE', *, *, #12965, .F. ) ;
#13159=EDGE_CURVE ( 'NONE', #11181, #1460, #8015, .T. ) ;
#13161=EDGE_CURVE ( 'NONE', #4254, #17707, #12054, .T. ) ;
#13163=EDGE_CURVE ( 'NONE', #9789, #2703, #15128, .T. ) ;
#13167=EDGE_CURVE ( 'NONE', #13281, #3722, #15218, .T. ) ;
#13170=VERTEX_POINT ( 'NONE', #9157 ) ;
#13173=ORIENTED_EDGE ( 'NONE', *, *, #7003, .F. ) ;
#13177=VERTEX_POINT ( 'NONE', #2404 ) ;
#13178=CARTESIAN_POINT ( 'NONE',  ( -71.24615306438090556, 60.26648315456375826, 15.00000000000006928 ) ) ;
#13179=LINE ( 'NONE', #16332, #7934 ) ;
#13180=EDGE_CURVE ( 'NONE', #15619, #14794, #14843, .T. ) ;
#13183=EDGE_CURVE ( 'NONE', #115, #13022, #2128, .T. ) ;
#13187=ORIENTED_EDGE ( 'NONE', *, *, #5822, .T. ) ;
#13194=VECTOR ( 'NONE', #13876, 1000.000000000000000 ) ;
#13199=CARTESIAN_POINT ( 'NONE',  ( -71.24615306438109030, 27.96168591522921076, -15.00000000000001421 ) ) ;
#13206=CARTESIAN_POINT ( 'NONE',  ( -71.24615306438091977, 72.83285375456371469, -167.1454815528550739 ) ) ;
#13207=LINE ( 'NONE', #17775, #14912 ) ;
#13208=ORIENTED_EDGE ( 'NONE', *, *, #12346, .T. ) ;
#13210=CARTESIAN_POINT ( 'NONE',  ( -68.99615306438106188, 36.56753083813027416, 15.00000000000006928 ) ) ;
#13211=VECTOR ( 'NONE', #13872, 1000.000000000000000 ) ;
#13212=CARTESIAN_POINT ( 'NONE',  ( -71.24615306438106188, 37.38646386522923137, 15.00000000000006928 ) ) ;
#13219=LINE ( 'NONE', #11462, #79 ) ;
#13221=EDGE_CURVE ( 'NONE', #18030, #12968, #536, .T. ) ;
#13227=FACE_OUTER_BOUND ( 'NONE', #618, .T. ) ;
#13229=ORIENTED_EDGE ( 'NONE', *, *, #3450, .F. ) ;
#13230=PLANE ( 'NONE',  #4457 ) ;
#13233=DIRECTION ( 'NONE',  ( 0.3420201433256724322, 0.9396926207859070956, -0.000000000000000000 ) ) ;
#13234=ORIENTED_EDGE ( 'NONE', *, *, #140, .T. ) ;
#13235=VECTOR ( 'NONE', #15995, 1000.000000000000000 ) ;
#13236=VECTOR ( 'NONE', #15675, 1000.000000000000000 ) ;
#13243=DIRECTION ( 'NONE',  ( 0.3420201433256686574, 0.9396926207859084279, -0.000000000000000000 ) ) ;
#13244=ORIENTED_EDGE ( 'NONE', *, *, #6384, .F. ) ;
#13246=CARTESIAN_POINT ( 'NONE',  ( -71.24615306438114715, 15.39531531522927921, -15.00000000000001421 ) ) ;
#13249=LINE ( 'NONE', #3699, #6622 ) ;
#13250=LINE ( 'NONE', #8671, #9330 ) ;
#13251=ORIENTED_EDGE ( 'NONE', *, *, #18329, .F. ) ;
#13258=VECTOR ( 'NONE', #5850, 1000.000000000000227 ) ;
#13263=CARTESIAN_POINT ( 'NONE',  ( -68.99615306438100504, 45.99230878813026635, -167.1454815528550739 ) ) ;
#13267=EDGE_CURVE ( 'NONE', #14227, #11339, #738, .T. ) ;
#13269=CARTESIAN_POINT ( 'NONE',  ( -71.24615306438080609, 116.8151508545637114, 15.00000000000006928 ) ) ;
#13270=PLANE ( 'NONE',  #18406 ) ;
#13271=DIRECTION ( 'NONE',  ( 0.9396926207859110924, 0.3420201433256612189, 4.890320548438462711E-16 ) ) ;
#13277=ORIENTED_EDGE ( 'NONE', *, *, #18213, .T. ) ;
#13281=VERTEX_POINT ( 'NONE', #9434 ) ;
#13285=EDGE_CURVE ( 'NONE', #7166, #2933, #17925, .T. ) ;
#13286=EDGE_CURVE ( 'NONE', #7142, #4127, #17755, .T. ) ;
#13287=VECTOR ( 'NONE', #15711, 1000.000000000000000 ) ;
#13290=VECTOR ( 'NONE', #106, 1000.000000000000000 ) ;
#13292=LINE ( 'NONE', #14588, #14150 ) ;
#13294=CARTESIAN_POINT ( 'NONE',  ( -71.24615306438091977, 75.97444640456376419, -167.1454815528550739 ) ) ;
#13297=CARTESIAN_POINT ( 'NONE',  ( -71.24615306438086293, 100.2183168652291982, -167.1454815528550739 ) ) ;
#13302=DIRECTION ( 'NONE',  ( 1.000000000000000000, 0.000000000000000000, 0.000000000000000000 ) ) ;
#13303=ORIENTED_EDGE ( 'NONE', *, *, #11778, .T. ) ;
#13306=VECTOR ( 'NONE', #7852, 1000.000000000000114 ) ;
#13307=LINE ( 'NONE', #765, #15192 ) ;
#13318=ORIENTED_EDGE ( 'NONE', *, *, #8100, .F. ) ;
#13320=LINE ( 'NONE', #2168, #17080 ) ;
#13321=PLANE ( 'NONE',  #15376 ) ;
#13322=LINE ( 'NONE', #499, #15309 ) ;
#13324=DIRECTION ( 'NONE',  ( -0.000000000000000000, 1.000000000000000000, -0.000000000000000000 ) ) ;
#13327=VERTEX_POINT ( 'NONE', #16912 ) ;
#13329=VERTEX_POINT ( 'NONE', #18505 ) ;
#13332=VERTEX_POINT ( 'NONE', #14020 ) ;
#13336=CARTESIAN_POINT ( 'NONE',  ( -71.24615306438080609, 106.5015021652292404, -167.1454815528550739 ) ) ;
#13340=EDGE_CURVE ( 'NONE', #2025, #9102, #12530, .T. ) ;
#13341=ORIENTED_EDGE ( 'NONE', *, *, #11698, .T. ) ;
#13343=LINE ( 'NONE', #7278, #4213 ) ;
#13344=ORIENTED_EDGE ( 'NONE', *, *, #8358, .F. ) ;
#13345=EDGE_LOOP ( 'NONE', ( #17587, #8022, #15843, #9724 ) ) ;
#13347=LINE ( 'NONE', #16409, #12062 ) ;
#13352=CARTESIAN_POINT ( 'NONE',  ( -71.24615306438080609, 107.3903729045637192, -167.1454815528550739 ) ) ;
#13353=VERTEX_POINT ( 'NONE', #15611 ) ;
#13354=CARTESIAN_POINT ( 'NONE',  ( -71.24615306438094819, 68.80239036522922902, -167.1454815528550739 ) ) ;
#13357=CARTESIAN_POINT ( 'NONE',  ( -68.99615306438077766, 124.5321250381302747, -167.1454815528550739 ) ) ;
#13360=DIRECTION ( 'NONE',  ( 1.000000000000000000, 0.000000000000000000, 0.000000000000000000 ) ) ;
#13366=ADVANCED_FACE ( 'NONE', ( #11124 ), #9902, .T. ) ;
#13367=EDGE_CURVE ( 'NONE', #11181, #9065, #12632, .T. ) ;
#13368=VERTEX_POINT ( 'NONE', #15507 ) ;
#13370=LINE ( 'NONE', #2239, #13834 ) ;
#13371=DIRECTION ( 'NONE',  ( 0.3420201433256686574, -0.9396926207859084279, 0.000000000000000000 ) ) ;
#13373=EDGE_CURVE ( 'NONE', #17050, #9018, #11403, .T. ) ;
#13374=DIRECTION ( 'NONE',  ( 0.000000000000000000, 1.000000000000000000, 0.000000000000000000 ) ) ;
#13376=VERTEX_POINT ( 'NONE', #6720 ) ;
#13378=EDGE_CURVE ( 'NONE', #794, #1345, #12806, .T. ) ;
#13381=PLANE ( 'NONE',  #4194 ) ;
#13382=ORIENTED_EDGE ( 'NONE', *, *, #2067, .F. ) ;
#13388=ADVANCED_FACE ( 'NONE', ( #17000 ), #13826, .T. ) ;
#13389=ADVANCED_FACE ( 'NONE', ( #17097 ), #11310, .T. ) ;
#13392=EDGE_CURVE ( 'NONE', #3197, #7512, #14216, .T. ) ;
#13393=LINE ( 'NONE', #2338, #10305 ) ;
#13394=DIRECTION ( 'NONE',  ( 0.000000000000000000, 0.000000000000000000, 1.000000000000000000 ) ) ;
#13395=CARTESIAN_POINT ( 'NONE',  ( -68.99615306438086293, 92.50134268166266338, 15.00000000000006928 ) ) ;
#13396=ORIENTED_EDGE ( 'NONE', *, *, #18208, .T. ) ;
#13397=FACE_OUTER_BOUND ( 'NONE', #7384, .T. ) ;
#13398=ORIENTED_EDGE ( 'NONE', *, *, #17888, .T. ) ;
#13400=LINE ( 'NONE', #14611, #13778 ) ;
#13405=EDGE_CURVE ( 'NONE', #4483, #10712, #18134, .T. ) ;
#13406=ADVANCED_FACE ( 'NONE', ( #11024 ), #3904, .T. ) ;
#13407=LINE ( 'NONE', #11830, #3859 ) ;
#13412=VECTOR ( 'NONE', #17257, 1000.000000000000000 ) ;
#13413=ORIENTED_EDGE ( 'NONE', *, *, #6400, .T. ) ;
#13414=LINE ( 'NONE', #16389, #1642 ) ;
#13415=CARTESIAN_POINT ( 'NONE',  ( -71.24615306438076345, 123.0983361545637109, -167.1454815528550739 ) ) ;
#13417=CARTESIAN_POINT ( 'NONE',  ( -68.99615306438117557, 5.151604338130305827, -15.00000000000001421 ) ) ;
#13423=CARTESIAN_POINT ( 'NONE',  ( -70.27900850916093134, -2.213358015103445098, 15.00000000000008171 ) ) ;
#13424=DIRECTION ( 'NONE',  ( 0.3420201433256891965, 0.9396926207859008784, -0.000000000000000000 ) ) ;
#13431=VECTOR ( 'NONE', #4145, 1000.000000000000000 ) ;
#13447=PLANE ( 'NONE',  #6026 ) ;
#13448=DIRECTION ( 'NONE',  ( 0.000000000000000000, 1.000000000000000000, 0.000000000000000000 ) ) ;
#13450=DIRECTION ( 'NONE',  ( 0.000000000000000000, 0.000000000000000000, 1.000000000000000000 ) ) ;
#13452=VECTOR ( 'NONE', #14844, 1000.000000000000000 ) ;
#13457=VERTEX_POINT ( 'NONE', #5863 ) ;
#13458=AXIS2_PLACEMENT_3D ( 'NONE', #1309, #17099, #8308 ) ;
#13459=ORIENTED_EDGE ( 'NONE', *, *, #13630, .T. ) ;
#13460=PLANE ( 'NONE',  #1315 ) ;
#13464=PLANE ( 'NONE',  #4858 ) ;
#13465=VECTOR ( 'NONE', #8509, 1000.000000000000000 ) ;
#13466=CARTESIAN_POINT ( 'NONE',  ( -70.27900850916091713, -2.213358015103439325, -15.00000000000001421 ) ) ;
#13467=CARTESIAN_POINT ( 'NONE',  ( -68.99615306438111872, 20.24471173166267235, 15.00000000000006928 ) ) ;
#13468=VECTOR ( 'NONE', #8586, 1000.000000000000000 ) ;
#13469=EDGE_CURVE ( 'NONE', #9102, #5451, #1829, .T. ) ;
#13470=DIRECTION ( 'NONE',  ( 0.9396926207859084279, 0.3420201433256686574, 4.890320548438448905E-16 ) ) ;
#13479=LINE ( 'NONE', #7592, #858 ) ;
#13482=VECTOR ( 'NONE', #6554, 1000.000000000000000 ) ;
#13487=FACE_OUTER_BOUND ( 'NONE', #178, .T. ) ;
#13489=DIRECTION ( 'NONE',  ( 1.000000000000000000, 0.000000000000000000, 0.000000000000000000 ) ) ;
#13491=VECTOR ( 'NONE', #5543, 1000.000000000000114 ) ;
#13492=CARTESIAN_POINT ( 'NONE',  ( -71.24615306438107609, 10.00100075456378157, 15.00000000000006928 ) ) ;
#13493=FACE_OUTER_BOUND ( 'NONE', #17333, .T. ) ;
#13495=EDGE_CURVE ( 'NONE', #2512, #12063, #16127, .T. ) ;
#13499=EDGE_CURVE ( 'NONE', #4091, #6989, #73, .T. ) ;
#13500=CARTESIAN_POINT ( 'NONE',  ( -71.24615306438109030, 27.96168591522921076, -167.1454815528550739 ) ) ;
#13503=FACE_OUTER_BOUND ( 'NONE', #13757, .T. ) ;
#13504=ORIENTED_EDGE ( 'NONE', *, *, #8928, .T. ) ;
#13505=CARTESIAN_POINT ( 'NONE',  ( -71.24615306438086293, 91.68240965456375591, -167.1454815528550739 ) ) ;
#13508=VECTOR ( 'NONE', #14715, 1000.000000000000227 ) ;
#13512=VECTOR ( 'NONE', #631, 1000.000000000000000 ) ;
#13514=EDGE_CURVE ( 'NONE', #5525, #6089, #15868, .T. ) ;
#13515=CARTESIAN_POINT ( 'NONE',  ( -71.24615306438090556, 57.12489050456379402, 15.00000000000006928 ) ) ;
#13518=LINE ( 'NONE', #7902, #1930 ) ;
#13520=ADVANCED_FACE ( 'NONE', ( #14295 ), #7444, .T. ) ;
#13521=VECTOR ( 'NONE', #17413, 1000.000000000000000 ) ;
#13523=ORIENTED_EDGE ( 'NONE', *, *, #9593, .T. ) ;
#13529=CARTESIAN_POINT ( 'NONE',  ( -68.99615306438080609, 108.2093059316626693, 15.00000000000006928 ) ) ;
#13532=ORIENTED_EDGE ( 'NONE', *, *, #140, .F. ) ;
#13533=CARTESIAN_POINT ( 'NONE',  ( -71.24615306438110451, 22.56737135456380372, -15.00000000000001421 ) ) ;
#13539=( NAMED_UNIT ( * ) SI_UNIT ( $, .STERADIAN. ) SOLID_ANGLE_UNIT ( ) );
#13543=ORIENTED_EDGE ( 'NONE', *, *, #8937, .T. ) ;
#13544=LINE ( 'NONE', #529, #9274 ) ;
#13545=CARTESIAN_POINT ( 'NONE',  ( -71.24615306438103346, 47.70011255456374499, -167.1454815528550739 ) ) ;
#13547=DIRECTION ( 'NONE',  ( 0.000000000000000000, 1.000000000000000000, 0.000000000000000000 ) ) ;
#13549=CARTESIAN_POINT ( 'NONE',  ( -68.99615306438087714, 71.12504998813027157, 15.00000000000006928 ) ) ;
#13555=ORIENTED_EDGE ( 'NONE', *, *, #11656, .F. ) ;
#13559=ORIENTED_EDGE ( 'NONE', *, *, #5806, .F. ) ;
#13561=DIRECTION ( 'NONE',  ( 0.3420201433256727097, 0.9396926207859069846, -0.000000000000000000 ) ) ;
#13566=VECTOR ( 'NONE', #5152, 1000.000000000000000 ) ;
#13568=ORIENTED_EDGE ( 'NONE', *, *, #13340, .T. ) ;
#13569=CARTESIAN_POINT ( 'NONE',  ( -71.24615306438079188, 94.82400230456380541, 15.00000000000006928 ) ) ;
#13571=ORIENTED_EDGE ( 'NONE', *, *, #13983, .F. ) ;
#13574=CARTESIAN_POINT ( 'NONE',  ( -71.24615306438107609, 16.28418605456382906, 15.00000000000006928 ) ) ;
#13576=VERTEX_POINT ( 'NONE', #16044 ) ;
#13585=DIRECTION ( 'NONE',  ( 0.9396926207859069846, 0.3420201433256723766, 4.890320548438442003E-16 ) ) ;
#13589=DIRECTION ( 'NONE',  ( 0.3420201433256724322, 0.9396926207859070956, -0.000000000000000000 ) ) ;
#13592=VECTOR ( 'NONE', #3411, 1000.000000000000000 ) ;
#13596=DIRECTION ( 'NONE',  ( 0.9396926207859157554, 0.3420201433256481738, 4.890320548438487362E-16 ) ) ;
#13601=VERTEX_POINT ( 'NONE', #7275 ) ;
#13602=LINE ( 'NONE', #16385, #533 ) ;
#13604=ORIENTED_EDGE ( 'NONE', *, *, #14181, .T. ) ;
#13605=VECTOR ( 'NONE', #16888, 1000.000000000000000 ) ;
#13606=EDGE_CURVE ( 'NONE', #14578, #15061, #17267, .T. ) ;
#13611=EDGE_LOOP ( 'NONE', ( #10477, #16717, #4906, #2200 ) ) ;
#13612=CARTESIAN_POINT ( 'NONE',  ( -71.24615306438080609, 115.9262801152292042, -15.00000000000001421 ) ) ;
#13613=FACE_OUTER_BOUND ( 'NONE', #1376, .T. ) ;
#13617=VERTEX_POINT ( 'NONE', #17727 ) ;
#13620=CARTESIAN_POINT ( 'NONE',  ( -71.24615306438117557, 2.828944715229236628, 15.00000000000006928 ) ) ;
#13625=CARTESIAN_POINT ( 'NONE',  ( -68.99615306438080609, 108.8241617881302545, -167.1454815528550739 ) ) ;
#13626=ORIENTED_EDGE ( 'NONE', *, *, #3441, .T. ) ;
#13627=EDGE_LOOP ( 'NONE', ( #5873, #6236, #2631, #13135 ) ) ;
#13628=EDGE_CURVE ( 'NONE', #14282, #797, #16503, .T. ) ;
#13629=EDGE_CURVE ( 'NONE', #10960, #12217, #3318, .T. ) ;
#13630=EDGE_CURVE ( 'NONE', #6089, #7142, #9413, .T. ) ;
#13633=FACE_OUTER_BOUND ( 'NONE', #5862, .T. ) ;
#13637=DIRECTION ( 'NONE',  ( 0.000000000000000000, 0.000000000000000000, 1.000000000000000000 ) ) ;
#13638=FACE_OUTER_BOUND ( 'NONE', #17598, .T. ) ;
#13640=LINE ( 'NONE', #12330, #5696 ) ;
#13642=CARTESIAN_POINT ( 'NONE',  ( -71.24615306438114715, 16.28418605456380419, -167.1454815528550739 ) ) ;
#13644=VERTEX_POINT ( 'NONE', #12314 ) ;
#13652=ORIENTED_EDGE ( 'NONE', *, *, #5841, .F. ) ;
#13661=DIRECTION ( 'NONE',  ( 0.000000000000000000, 0.000000000000000000, 1.000000000000000000 ) ) ;
#13666=CARTESIAN_POINT ( 'NONE',  ( -71.24615306438076345, 119.9567435045637609, -15.00000000000001421 ) ) ;
#13670=ORIENTED_EDGE ( 'NONE', *, *, #7436, .F. ) ;
#13676=DIRECTION ( 'NONE',  ( -0.9396926207859069846, 0.3420201433256723766, -4.890320548438442003E-16 ) ) ;
#13679=ORIENTED_EDGE ( 'NONE', *, *, #6295, .F. ) ;
#13680=DIRECTION ( 'NONE',  ( 0.000000000000000000, 0.000000000000000000, 1.000000000000000000 ) ) ;
#13686=PLANE ( 'NONE',  #17031 ) ;
#13689=ORIENTED_EDGE ( 'NONE', *, *, #14221, .T. ) ;
#13695=ADVANCED_FACE ( 'NONE', ( #7911 ), #9219, .T. ) ;
#13696=CARTESIAN_POINT ( 'NONE',  ( -70.27900850916093134, -2.213358015103445098, -167.1454815528550739 ) ) ;
#13697=DIRECTION ( 'NONE',  ( 0.9396926207859069846, 0.3420201433256723766, -1.086737899652988166E-16 ) ) ;
#13698=ORIENTED_EDGE ( 'NONE', *, *, #3280, .T. ) ;
#13703=CARTESIAN_POINT ( 'NONE',  ( -71.24615306438117557, 3.717815454563750954, 15.00000000000006928 ) ) ;
#13707=VECTOR ( 'NONE', #5045, 1000.000000000000000 ) ;
#13710=EDGE_CURVE ( 'NONE', #1317, #10905, #7813, .T. ) ;
#13713=EDGE_CURVE ( 'NONE', #3860, #15763, #3591, .T. ) ;
#13714=ORIENTED_EDGE ( 'NONE', *, *, #4838, .F. ) ;
#13720=DIRECTION ( 'NONE',  ( 0.000000000000000000, 0.000000000000000000, 1.000000000000000000 ) ) ;
#13724=VERTEX_POINT ( 'NONE', #3877 ) ;
#13732=PLANE ( 'NONE',  #13755 ) ;
#13735=AXIS2_PLACEMENT_3D ( 'NONE', #6098, #11907, #9201 ) ;
#13740=EDGE_LOOP ( 'NONE', ( #15448, #995, #11309, #4963 ) ) ;
#13742=CARTESIAN_POINT ( 'NONE',  ( -71.24615306438114715, 15.39531531522927921, -15.00000000000001421 ) ) ;
#13746=CARTESIAN_POINT ( 'NONE',  ( -71.24615306438097662, 60.26648315456372984, -167.1454815528550739 ) ) ;
#13751=VECTOR ( 'NONE', #1350, 999.9999999999998863 ) ;
#13752=ADVANCED_FACE ( 'NONE', ( #8191 ), #7324, .T. ) ;
#13753=DIRECTION ( 'NONE',  ( 0.3420201433256649937, 0.9396926207859097602, -0.000000000000000000 ) ) ;
#13754=VECTOR ( 'NONE', #18240, 1000.000000000000000 ) ;
#13755=AXIS2_PLACEMENT_3D ( 'NONE', #10939, #15034, #5220 ) ;
#13756=LINE ( 'NONE', #5041, #7770 ) ;
#13757=EDGE_LOOP ( 'NONE', ( #18023, #17273, #520, #11529 ) ) ;
#13760=ORIENTED_EDGE ( 'NONE', *, *, #3106, .F. ) ;
#13762=VECTOR ( 'NONE', #7015, 1000.000000000000000 ) ;
#13768=CARTESIAN_POINT ( 'NONE',  ( -71.24615306438109030, 24.82009326522924297, -15.00000000000001421 ) ) ;
#13771=LINE ( 'NONE', #13492, #886 ) ;
#13773=ORIENTED_EDGE ( 'NONE', *, *, #2298, .F. ) ;
#13776=FACE_OUTER_BOUND ( 'NONE', #15305, .T. ) ;
#13777=VERTEX_POINT ( 'NONE', #211 ) ;
#13778=VECTOR ( 'NONE', #3482, 1000.000000000000000 ) ;
#13779=DIRECTION ( 'NONE',  ( 0.000000000000000000, 0.000000000000000000, 1.000000000000000000 ) ) ;
#13780=DIRECTION ( 'NONE',  ( 0.3420201433256686574, -0.9396926207859084279, 0.000000000000000000 ) ) ;
#13782=AXIS2_PLACEMENT_3D ( 'NONE', #17263, #67, #5764 ) ;
#13785=ORIENTED_EDGE ( 'NONE', *, *, #18207, .F. ) ;
#13787=EDGE_LOOP ( 'NONE', ( #18361, #5758, #2119, #18136 ) ) ;
#13789=LINE ( 'NONE', #4072, #12021 ) ;
#13794=CARTESIAN_POINT ( 'NONE',  ( -68.99615306438066398, 130.8153103381302458, 15.00000000000006928 ) ) ;
#13796=LINE ( 'NONE', #9407, #1812 ) ;
#13797=DIRECTION ( 'NONE',  ( 0.000000000000000000, 0.000000000000000000, 1.000000000000000000 ) ) ;
#13798=LINE ( 'NONE', #12307, #17096 ) ;
#13799=EDGE_LOOP ( 'NONE', ( #8941, #1619, #17082, #8242 ) ) ;
#13803=AXIS2_PLACEMENT_3D ( 'NONE', #13415, #16589, #9027 ) ;
#13804=DIRECTION ( 'NONE',  ( 0.9396926207859158664, 0.3420201433256481738, -1.086737899652998397E-16 ) ) ;
#13807=VERTEX_POINT ( 'NONE', #16978 ) ;
#13808=ORIENTED_EDGE ( 'NONE', *, *, #6041, .T. ) ;
#13814=LINE ( 'NONE', #6993, #17606 ) ;
#13826=PLANE ( 'NONE',  #6405 ) ;
#13832=ORIENTED_EDGE ( 'NONE', *, *, #5576, .T. ) ;
#13834=VECTOR ( 'NONE', #10948, 1000.000000000000000 ) ;
#13837=DIRECTION ( 'NONE',  ( 0.000000000000000000, 1.000000000000000000, -0.000000000000000000 ) ) ;
#13838=EDGE_CURVE ( 'NONE', #7151, #11452, #15191, .T. ) ;
#13839=VERTEX_POINT ( 'NONE', #1098 ) ;
#13842=DIRECTION ( 'NONE',  ( 0.3420201433256854218, 0.9396926207859023217, -0.000000000000000000 ) ) ;
#13845=DIRECTION ( 'NONE',  ( 0.3420201433256929158, 0.9396926207858996571, -0.000000000000000000 ) ) ;
#13848=LINE ( 'NONE', #16544, #16489 ) ;
#13850=FACE_OUTER_BOUND ( 'NONE', #16046, .T. ) ;
#13852=AXIS2_PLACEMENT_3D ( 'NONE', #15618, #14226, #5684 ) ;
#13854=EDGE_CURVE ( 'NONE', #5784, #17050, #18300, .T. ) ;
#13855=VERTEX_POINT ( 'NONE', #12509 ) ;
#13858=EDGE_CURVE ( 'NONE', #10943, #12606, #18202, .T. ) ;
#13859=EDGE_LOOP ( 'NONE', ( #6007, #12404, #7330, #11521 ) ) ;
#13860=EDGE_CURVE ( 'NONE', #10561, #6934, #11197, .T. ) ;
#13863=ADVANCED_FACE ( 'NONE', ( #12703 ), #4085, .T. ) ;
#13864=ADVANCED_FACE ( 'NONE', ( #11292 ), #1979, .T. ) ;
#13869=CARTESIAN_POINT ( 'NONE',  ( -71.24615306438076345, 125.3510580652292248, -167.1454815528550739 ) ) ;
#13870=CARTESIAN_POINT ( 'NONE',  ( -68.99615306438089135, 80.54982793813027797, -167.1454815528550739 ) ) ;
#13872=DIRECTION ( 'NONE',  ( 0.000000000000000000, 0.000000000000000000, 1.000000000000000000 ) ) ;
#13875=FACE_OUTER_BOUND ( 'NONE', #16301, .T. ) ;
#13876=DIRECTION ( 'NONE',  ( 0.000000000000000000, 0.000000000000000000, 1.000000000000000000 ) ) ;
#13878=EDGE_LOOP ( 'NONE', ( #2726, #12753, #1641, #12184 ) ) ;
#13887=ADVANCED_FACE ( 'NONE', ( #11618 ), #8999, .T. ) ;
#13888=ORIENTED_EDGE ( 'NONE', *, *, #9328, .T. ) ;
#13899=CARTESIAN_POINT ( 'NONE',  ( -71.24615306438080609, 110.5319655545637403, 15.00000000000006928 ) ) ;
#13900=VERTEX_POINT ( 'NONE', #6162 ) ;
#13902=DIRECTION ( 'NONE',  ( 1.000000000000000000, 0.000000000000000000, 0.000000000000000000 ) ) ;
#13904=ORIENTED_EDGE ( 'NONE', *, *, #9492, .F. ) ;
#13909=AXIS2_PLACEMENT_3D ( 'NONE', #15919, #3109, #14521 ) ;
#13912=ORIENTED_EDGE ( 'NONE', *, *, #12894, .F. ) ;
#13916=ORIENTED_EDGE ( 'NONE', *, *, #11910, .T. ) ;
#13919=CARTESIAN_POINT ( 'NONE',  ( -71.24615306438097662, 57.12489050456376560, -167.1454815528550739 ) ) ;
#13922=EDGE_CURVE ( 'NONE', #13177, #16319, #7493, .T. ) ;
#13923=CARTESIAN_POINT ( 'NONE',  ( -71.24615306438086293, 93.93513156522925556, 15.00000000000006928 ) ) ;
#13924=VECTOR ( 'NONE', #13271, 1000.000000000000114 ) ;
#13926=DIRECTION ( 'NONE',  ( 0.9396926207859185309, 0.3420201433256406798, 0.000000000000000000 ) ) ;
#13927=AXIS2_PLACEMENT_3D ( 'NONE', #13545, #629, #11858 ) ;
#13929=FACE_OUTER_BOUND ( 'NONE', #3770, .T. ) ;
#13930=ORIENTED_EDGE ( 'NONE', *, *, #16015, .T. ) ;
#13936=ORIENTED_EDGE ( 'NONE', *, *, #11252, .T. ) ;
#13941=VERTEX_POINT ( 'NONE', #13210 ) ;
#13942=ADVANCED_FACE ( 'NONE', ( #7766 ), #10582, .T. ) ;
#13943=LINE ( 'NONE', #18439, #11955 ) ;
#13956=ORIENTED_EDGE ( 'NONE', *, *, #8004, .T. ) ;
#13957=UNCERTAINTY_MEASURE_WITH_UNIT (LENGTH_MEASURE( 1.000000000000000082E-05 ), #368, 'distance_accuracy_value', 'NONE');
#13961=EDGE_CURVE ( 'NONE', #2933, #4021, #6078, .T. ) ;
#13962=DIRECTION ( 'NONE',  ( 0.000000000000000000, 1.000000000000000000, 0.000000000000000000 ) ) ;
#13965=LINE ( 'NONE', #1145, #5057 ) ;
#13968=CARTESIAN_POINT ( 'NONE',  ( -68.99615306438067819, 146.5232735881302801, -15.00000000000001421 ) ) ;
#13973=DIRECTION ( 'NONE',  ( 0.000000000000000000, 1.000000000000000000, 0.000000000000000000 ) ) ;
#13976=ADVANCED_FACE ( 'NONE', ( #14784 ), #4500, .F. ) ;
#13978=EDGE_CURVE ( 'NONE', #6648, #4422, #289, .T. ) ;
#13979=CARTESIAN_POINT ( 'NONE',  ( -71.24615306438070661, 141.9478920545637664, -15.00000000000001421 ) ) ;
#13983=EDGE_CURVE ( 'NONE', #1662, #16693, #5983, .T. ) ;
#13984=CARTESIAN_POINT ( 'NONE',  ( -71.24615306438076345, 123.0983361545637109, 15.00000000000006928 ) ) ;
#13992=DIRECTION ( 'NONE',  ( 1.000000000000000000, 0.000000000000000000, 0.000000000000000000 ) ) ;
#13993=ORIENTED_EDGE ( 'NONE', *, *, #4922, .T. ) ;
#14000=ORIENTED_EDGE ( 'NONE', *, *, #14103, .T. ) ;
#14003=ORIENTED_EDGE ( 'NONE', *, *, #16977, .F. ) ;
#14006=LINE ( 'NONE', #12426, #9988 ) ;
#14008=LINE ( 'NONE', #5384, #18515 ) ;
#14010=CARTESIAN_POINT ( 'NONE',  ( -68.99615306438080609, 105.0677132816627051, -167.1454815528550739 ) ) ;
#14013=DIRECTION ( 'NONE',  ( -0.9396926207859084279, 0.3420201433256686574, 1.086737899652989892E-16 ) ) ;
#14020=CARTESIAN_POINT ( 'NONE',  ( -71.24615306438086293, 88.54081700456373483, -15.00000000000001421 ) ) ;
#14024=ORIENTED_EDGE ( 'NONE', *, *, #3091, .F. ) ;
#14026=EDGE_LOOP ( 'NONE', ( #9597, #8766, #1082, #14500 ) ) ;
#14031=ORIENTED_EDGE ( 'NONE', *, *, #15334, .F. ) ;
#14032=CARTESIAN_POINT ( 'NONE',  ( -71.24615306438114715, 12.25372266522925457, -15.00000000000001421 ) ) ;
#14035=ORIENTED_EDGE ( 'NONE', *, *, #2539, .F. ) ;
#14037=CARTESIAN_POINT ( 'NONE',  ( -71.24615306438080609, 115.9262801152292042, 15.00000000000006928 ) ) ;
#14038=DIRECTION ( 'NONE',  ( 0.000000000000000000, 1.000000000000000000, 0.000000000000000000 ) ) ;
#14040=CARTESIAN_POINT ( 'NONE',  ( -71.24615306438096241, 63.40807580456375803, -15.00000000000001421 ) ) ;
#14041=AXIS2_PLACEMENT_3D ( 'NONE', #14186, #1373, #14540 ) ;
#14046=ORIENTED_EDGE ( 'NONE', *, *, #9629, .T. ) ;
#14048=VERTEX_POINT ( 'NONE', #3834 ) ;
#14050=CARTESIAN_POINT ( 'NONE',  ( -71.24615306438113294, 13.14259340456378489, -15.00000000000001421 ) ) ;
#14051=VECTOR ( 'NONE', #3273, 1000.000000000000000 ) ;
#14054=EDGE_CURVE ( 'NONE', #16133, #288, #5326, .T. ) ;
#14059=LINE ( 'NONE', #207, #7226 ) ;
#14064=FACE_OUTER_BOUND ( 'NONE', #7943, .T. ) ;
#14065=ORIENTED_EDGE ( 'NONE', *, *, #10485, .F. ) ;
#14068=EDGE_CURVE ( 'NONE', #4994, #409, #16731, .T. ) ;
#14069=VECTOR ( 'NONE', #1389, 1000.000000000000000 ) ;
#14070=VECTOR ( 'NONE', #12551, 1000.000000000000000 ) ;
#14071=EDGE_LOOP ( 'NONE', ( #10941, #291, #11814, #831 ) ) ;
#14074=CARTESIAN_POINT ( 'NONE',  ( -68.99615306438076345, 118.2489397381302751, -15.00000000000001421 ) ) ;
#14076=VERTEX_POINT ( 'NONE', #12263 ) ;
#14078=ADVANCED_FACE ( 'NONE', ( #8039 ), #9642, .T. ) ;
#14080=CARTESIAN_POINT ( 'NONE',  ( -68.99615306438072082, 127.0588618316627105, -167.1454815528550739 ) ) ;
#14086=VECTOR ( 'NONE', #4631, 1000.000000000000000 ) ;
#14087=ORIENTED_EDGE ( 'NONE', *, *, #16106, .F. ) ;
#14093=EDGE_CURVE ( 'NONE', #6728, #18478, #5240, .T. ) ;
#14094=LINE ( 'NONE', #16891, #4316 ) ;
#14096=EDGE_CURVE ( 'NONE', #6867, #15862, #17778, .T. ) ;
#14098=VECTOR ( 'NONE', #5258, 1000.000000000000000 ) ;
#14100=LINE ( 'NONE', #10067, #7007 ) ;
#14103=EDGE_CURVE ( 'NONE', #8931, #13353, #4216, .T. ) ;
#14105=LINE ( 'NONE', #15495, #11047 ) ;
#14109=ORIENTED_EDGE ( 'NONE', *, *, #6957, .F. ) ;
#14112=PLANE ( 'NONE',  #141 ) ;
#14115=ORIENTED_EDGE ( 'NONE', *, *, #907, .T. ) ;
#14117=AXIS2_PLACEMENT_3D ( 'NONE', #16076, #8989, #1875 ) ;
#14119=CARTESIAN_POINT ( 'NONE',  ( -68.99615306438100504, 49.13390143813029454, -167.1454815528550739 ) ) ;
#14121=LINE ( 'NONE', #1310, #13762 ) ;
#14122=ORIENTED_EDGE ( 'NONE', *, *, #6530, .F. ) ;
#14126=VECTOR ( 'NONE', #13547, 1000.000000000000000 ) ;
#14131=EDGE_LOOP ( 'NONE', ( #6773, #16855, #16321, #10803 ) ) ;
#14132=CARTESIAN_POINT ( 'NONE',  ( -68.99615306438104767, 20.85956758813029310, 15.00000000000006928 ) ) ;
#14135=ORIENTED_EDGE ( 'NONE', *, *, #5959, .F. ) ;
#14143=ORIENTED_EDGE ( 'NONE', *, *, #13405, .T. ) ;
#14145=ORIENTED_EDGE ( 'NONE', *, *, #14312, .T. ) ;
#14146=VECTOR ( 'NONE', #11512, 1000.000000000000000 ) ;
#14147=DIRECTION ( 'NONE',  ( 0.3420201433256686574, -0.9396926207859084279, 0.000000000000000000 ) ) ;
#14148=CARTESIAN_POINT ( 'NONE',  ( -71.24615306438083451, 97.07672421522921979, -167.1454815528550739 ) ) ;
#14150=VECTOR ( 'NONE', #17219, 1000.000000000000114 ) ;
#14152=VECTOR ( 'NONE', #1246, 1000.000000000000114 ) ;
#14153=CARTESIAN_POINT ( 'NONE',  ( -71.24615306438086293, 87.65194626522927024, -167.1454815528550739 ) ) ;
#14154=ORIENTED_EDGE ( 'NONE', *, *, #13163, .T. ) ;
#14156=PLANE ( 'NONE',  #16763 ) ;
#14166=AXIS2_PLACEMENT_3D ( 'NONE', #5200, #9321, #10638 ) ;
#14167=VECTOR ( 'NONE', #15474, 1000.000000000000000 ) ;
#14178=ORIENTED_EDGE ( 'NONE', *, *, #5942, .T. ) ;
#14181=EDGE_CURVE ( 'NONE', #11028, #1745, #2994, .T. ) ;
#14184=VERTEX_POINT ( 'NONE', #10025 ) ;
#14186=CARTESIAN_POINT ( 'NONE',  ( -68.99615306438072082, 130.2004544816626890, -167.1454815528550739 ) ) ;
#14189=EDGE_LOOP ( 'NONE', ( #13157, #4982, #7106, #13318 ) ) ;
#14191=CARTESIAN_POINT ( 'NONE',  ( -68.99615306438086293, 89.97460588813027016, 15.00000000000006928 ) ) ;
#14192=VERTEX_POINT ( 'NONE', #1500 ) ;
#14195=VECTOR ( 'NONE', #10154, 999.9999999999998863 ) ;
#14196=VECTOR ( 'NONE', #18433, 1000.000000000000000 ) ;
#14197=VERTEX_POINT ( 'NONE', #5423 ) ;
#14206=LINE ( 'NONE', #5668, #13000 ) ;
#14209=LINE ( 'NONE', #8101, #5975 ) ;
#14213=ORIENTED_EDGE ( 'NONE', *, *, #14956, .F. ) ;
#14216=LINE ( 'NONE', #10000, #13287 ) ;
#14217=CARTESIAN_POINT ( 'NONE',  ( -68.99615306438083451, 98.78452798166264870, -15.00000000000001421 ) ) ;
#14219=ADVANCED_FACE ( 'NONE', ( #5613 ), #9928, .T. ) ;
#14221=EDGE_CURVE ( 'NONE', #797, #11906, #1418, .T. ) ;
#14223=EDGE_LOOP ( 'NONE', ( #589, #5362, #4407, #9523 ) ) ;
#14226=DIRECTION ( 'NONE',  ( 0.3420201433256444545, -0.9396926207859171987, 0.000000000000000000 ) ) ;
#14227=VERTEX_POINT ( 'NONE', #3083 ) ;
#14229=CARTESIAN_POINT ( 'NONE',  ( -71.24615306438097662, 62.51920506522922949, -167.1454815528550739 ) ) ;
#14230=CARTESIAN_POINT ( 'NONE',  ( -68.99615306438089135, 83.07656473166271383, 15.00000000000006928 ) ) ;
#14240=DIRECTION ( 'NONE',  ( 0.3420201433256649937, -0.9396926207859097602, 0.000000000000000000 ) ) ;
#14242=DIRECTION ( 'NONE',  ( 0.000000000000000000, 0.000000000000000000, -1.000000000000000000 ) ) ;
#14245=ORIENTED_EDGE ( 'NONE', *, *, #344, .F. ) ;
#14247=LINE ( 'NONE', #16948, #16866 ) ;
#14254=ORIENTED_EDGE ( 'NONE', *, *, #3536, .T. ) ;
#14255=DIRECTION ( 'NONE',  ( -0.9396926207859097602, 0.3420201433256649937, 1.086737899652991371E-16 ) ) ;
#14257=ORIENTED_EDGE ( 'NONE', *, *, #459, .F. ) ;
#14262=ORIENTED_EDGE ( 'NONE', *, *, #9951, .T. ) ;
#14264=CARTESIAN_POINT ( 'NONE',  ( -71.24615306438090556, 72.83285375456371469, -15.00000000000001421 ) ) ;
#14265=LINE ( 'NONE', #13126, #13521 ) ;
#14266=VERTEX_POINT ( 'NONE', #6053 ) ;
#14270=LINE ( 'NONE', #8281, #17175 ) ;
#14274=CARTESIAN_POINT ( 'NONE',  ( -68.99615306438083451, 98.78452798166264870, -167.1454815528550739 ) ) ;
#14276=FACE_OUTER_BOUND ( 'NONE', #1594, .T. ) ;
#14277=ORIENTED_EDGE ( 'NONE', *, *, #11698, .F. ) ;
#14278=EDGE_LOOP ( 'NONE', ( #12037, #13068, #6849, #16699 ) ) ;
#14279=CARTESIAN_POINT ( 'NONE',  ( -71.24615306438086293, 91.68240965456375591, 15.00000000000006928 ) ) ;
#14281=VERTEX_POINT ( 'NONE', #9070 ) ;
#14282=VERTEX_POINT ( 'NONE', #8886 ) ;
#14287=CARTESIAN_POINT ( 'NONE',  ( -71.24615306438094819, 69.69126110456375045, -167.1454815528550739 ) ) ;
#14288=CARTESIAN_POINT ( 'NONE',  ( -71.24615306438070661, 134.7758360152292312, -15.00000000000001421 ) ) ;
#14290=EDGE_LOOP ( 'NONE', ( #14024, #78, #5015, #15411 ) ) ;
#14292=FACE_OUTER_BOUND ( 'NONE', #2608, .T. ) ;
#14293=CARTESIAN_POINT ( 'NONE',  ( -71.24615306438076345, 132.5231141045637457, -167.1454815528550739 ) ) ;
#14295=FACE_OUTER_BOUND ( 'NONE', #14189, .T. ) ;
#14298=CARTESIAN_POINT ( 'NONE',  ( -68.99615306438066398, 140.2400882881302664, 15.00000000000006928 ) ) ;
#14304=ORIENTED_EDGE ( 'NONE', *, *, #3691, .T. ) ;
#14312=EDGE_CURVE ( 'NONE', #11918, #11230, #6139, .T. ) ;
#14313=DIRECTION ( 'NONE',  ( 1.000000000000000000, 0.000000000000000000, 0.000000000000000000 ) ) ;
#14317=CARTESIAN_POINT ( 'NONE',  ( -68.99615306438072082, 139.6252324316626812, -15.00000000000001421 ) ) ;
#14318=PLANE ( 'NONE',  #11964 ) ;
#14320=ADVANCED_FACE ( 'NONE', ( #17293 ), #4479, .T. ) ;
#14325=ORIENTED_EDGE ( 'NONE', *, *, #17276, .T. ) ;
#14330=LINE ( 'NONE', #4226, #4740 ) ;
#14332=LINE ( 'NONE', #4321, #10443 ) ;
#14334=ORIENTED_EDGE ( 'NONE', *, *, #3999, .T. ) ;
#14336=ORIENTED_EDGE ( 'NONE', *, *, #9247, .T. ) ;
#14338=VECTOR ( 'NONE', #12132, 1000.000000000000000 ) ;
#14339=LINE ( 'NONE', #5896, #10456 ) ;
#14340=ORIENTED_EDGE ( 'NONE', *, *, #18315, .F. ) ;
#14342=VERTEX_POINT ( 'NONE', #6519 ) ;
#14344=ORIENTED_EDGE ( 'NONE', *, *, #14871, .F. ) ;
#14346=CARTESIAN_POINT ( 'NONE',  ( -68.99615306438111872, 10.81993378166265529, 15.00000000000006928 ) ) ;
#14347=CARTESIAN_POINT ( 'NONE',  ( -68.99615306438067819, 145.9084177316626949, 15.00000000000006928 ) ) ;
#14350=CARTESIAN_POINT ( 'NONE',  ( -71.24615306438106188, 35.13374195456378146, -167.1454815528550739 ) ) ;
#14358=VECTOR ( 'NONE', #11876, 1000.000000000000114 ) ;
#14359=VERTEX_POINT ( 'NONE', #7940 ) ;
#14368=CARTESIAN_POINT ( 'NONE',  ( -71.24615306438114715, 10.00100075456375492, 15.00000000000006928 ) ) ;
#14370=VECTOR ( 'NONE', #17271, 1000.000000000000000 ) ;
#14377=ORIENTED_EDGE ( 'NONE', *, *, #16934, .F. ) ;
#14380=DIRECTION ( 'NONE',  ( 0.000000000000000000, 0.000000000000000000, 1.000000000000000000 ) ) ;
#14381=VECTOR ( 'NONE', #16040, 1000.000000000000000 ) ;
#14385=EDGE_CURVE ( 'NONE', #1535, #14470, #9339, .T. ) ;
#14387=EDGE_CURVE ( 'NONE', #5064, #2297, #12342, .T. ) ;
#14389=VECTOR ( 'NONE', #10576, 1000.000000000000000 ) ;
#14391=CARTESIAN_POINT ( 'NONE',  ( -71.24615306438073503, 129.3815214545637104, 15.00000000000006928 ) ) ;
#14392=CARTESIAN_POINT ( 'NONE',  ( -71.24615306438106188, 37.38646386522923137, -15.00000000000001421 ) ) ;
#14398=DIRECTION ( 'NONE',  ( 0.000000000000000000, 1.000000000000000000, 0.000000000000000000 ) ) ;
#14401=VERTEX_POINT ( 'NONE', #2228 ) ;
#14405=CARTESIAN_POINT ( 'NONE',  ( -71.24615306438100504, 50.84170520456370923, -15.00000000000001421 ) ) ;
#14409=DIRECTION ( 'NONE',  ( -0.9396926207859084279, 0.3420201433256689905, -4.890320548438449892E-16 ) ) ;
#14411=ORIENTED_EDGE ( 'NONE', *, *, #9174, .F. ) ;
#14412=EDGE_CURVE ( 'NONE', #11452, #6852, #1019, .T. ) ;
#14413=ADVANCED_FACE ( 'NONE', ( #10734 ), #13732, .T. ) ;
#14416=EDGE_CURVE ( 'NONE', #1616, #14359, #16624, .T. ) ;
#14417=VERTEX_POINT ( 'NONE', #10833 ) ;
#14418=CARTESIAN_POINT ( 'NONE',  ( -71.24615306438103346, 41.41692725456378099, -167.1454815528550739 ) ) ;
#14421=VECTOR ( 'NONE', #2361, 1000.000000000000000 ) ;
#14424=DIRECTION ( 'NONE',  ( 0.3420201433256481738, 0.9396926207859158664, -0.000000000000000000 ) ) ;
#14426=ADVANCED_FACE ( 'NONE', ( #16711 ), #6434, .T. ) ;
#14432=VECTOR ( 'NONE', #18084, 1000.000000000000000 ) ;
#14434=DIRECTION ( 'NONE',  ( 0.000000000000000000, 1.000000000000000000, 0.000000000000000000 ) ) ;
#14437=ORIENTED_EDGE ( 'NONE', *, *, #9629, .F. ) ;
#14440=EDGE_CURVE ( 'NONE', #18243, #13143, #4191, .T. ) ;
#14447=DIRECTION ( 'NONE',  ( 0.000000000000000000, 1.000000000000000000, 0.000000000000000000 ) ) ;
#14450=CARTESIAN_POINT ( 'NONE',  ( -68.99615306438089135, 86.21815738166266385, -167.1454815528550739 ) ) ;
#14456=ORIENTED_EDGE ( 'NONE', *, *, #7501, .T. ) ;
#14464=AXIS2_PLACEMENT_3D ( 'NONE', #14744, #15879, #11675 ) ;
#14465=CARTESIAN_POINT ( 'NONE',  ( -68.99615306438106188, 29.66948968166269296, 15.00000000000006928 ) ) ;
#14470=VERTEX_POINT ( 'NONE', #6907 ) ;
#14472=CARTESIAN_POINT ( 'NONE',  ( -71.24615306438094819, 65.66079771522920794, -167.1454815528550739 ) ) ;
#14475=VECTOR ( 'NONE', #6190, 1000.000000000000000 ) ;
#14476=DIRECTION ( 'NONE',  ( 1.000000000000000000, 0.000000000000000000, 0.000000000000000000 ) ) ;
#14487=CARTESIAN_POINT ( 'NONE',  ( -71.24615306438103346, 40.52805651522925245, -167.1454815528550739 ) ) ;
#14493=DIRECTION ( 'NONE',  ( 0.9396926207859065405, 0.3420201433256737089, 0.000000000000000000 ) ) ;
#14499=LINE ( 'NONE', #3444, #3292 ) ;
#14500=ORIENTED_EDGE ( 'NONE', *, *, #15718, .F. ) ;
#14509=CARTESIAN_POINT ( 'NONE',  ( -71.24615306438076345, 131.6342433652292243, -15.00000000000001421 ) ) ;
#14510=DIRECTION ( 'NONE',  ( 0.000000000000000000, 1.000000000000000000, 0.000000000000000000 ) ) ;
#14511=LINE ( 'NONE', #10203, #558 ) ;
#14515=PLANE ( 'NONE',  #4231 ) ;
#14516=EDGE_CURVE ( 'NONE', #14266, #16358, #1397, .T. ) ;
#14521=DIRECTION ( 'NONE',  ( 0.9396926207859084279, 0.3420201433256686574, 0.000000000000000000 ) ) ;
#14524=ADVANCED_FACE ( 'NONE', ( #2510 ), #12532, .T. ) ;
#14525=EDGE_LOOP ( 'NONE', ( #93, #10676, #6187, #11932 ) ) ;
#14527=DIRECTION ( 'NONE',  ( 0.000000000000000000, 1.000000000000000000, 0.000000000000000000 ) ) ;
#14531=ORIENTED_EDGE ( 'NONE', *, *, #14387, .T. ) ;
#14535=DIRECTION ( 'NONE',  ( 0.3420201433256687684, 0.9396926207859084279, -0.000000000000000000 ) ) ;
#14539=EDGE_LOOP ( 'NONE', ( #16895, #10662, #7162, #926 ) ) ;
#14540=DIRECTION ( 'NONE',  ( 0.000000000000000000, 0.000000000000000000, -1.000000000000000000 ) ) ;
#14543=ORIENTED_EDGE ( 'NONE', *, *, #16329, .T. ) ;
#14549=CARTESIAN_POINT ( 'NONE',  ( -68.99615306438106188, 27.14275288813031040, -15.00000000000001421 ) ) ;
#14554=CARTESIAN_POINT ( 'NONE',  ( -68.99615306438067819, 142.7668250816626596, -15.00000000000001421 ) ) ;
#14556=CARTESIAN_POINT ( 'NONE',  ( -68.99615306438089135, 80.54982793813027797, 15.00000000000006928 ) ) ;
#14557=LINE ( 'NONE', #12992, #10815 ) ;
#14561=DIRECTION ( 'NONE',  ( -0.9396926207859084279, 0.3420201433256689905, 1.086737899652989769E-16 ) ) ;
#14564=ORIENTED_EDGE ( 'NONE', *, *, #14964, .F. ) ;
#14567=DIRECTION ( 'NONE',  ( 0.000000000000000000, 0.000000000000000000, 1.000000000000000000 ) ) ;
#14571=ORIENTED_EDGE ( 'NONE', *, *, #11797, .F. ) ;
#14574=CARTESIAN_POINT ( 'NONE',  ( -68.99615306438100504, 45.99230878813026635, 15.00000000000006928 ) ) ;
#14577=DIRECTION ( 'NONE',  ( 0.000000000000000000, 0.000000000000000000, 1.000000000000000000 ) ) ;
#14578=VERTEX_POINT ( 'NONE', #15318 ) ;
#14579=EDGE_CURVE ( 'NONE', #13177, #8500, #11312, .T. ) ;
#14581=DIRECTION ( 'NONE',  ( 0.9396926207859078728, 0.3420201433256701007, 4.890320548438446933E-16 ) ) ;
#14584=EDGE_CURVE ( 'NONE', #11293, #4896, #3320, .T. ) ;
#14588=CARTESIAN_POINT ( 'NONE',  ( -71.24615306438093398, 69.69126110456375045, -15.00000000000001421 ) ) ;
#14597=CARTESIAN_POINT ( 'NONE',  ( -68.99615306438097662, 58.55867938813025830, -167.1454815528550739 ) ) ;
#14598=VECTOR ( 'NONE', #5142, 1000.000000000000000 ) ;
#14599=ORIENTED_EDGE ( 'NONE', *, *, #15781, .T. ) ;
#14600=DIRECTION ( 'NONE',  ( -0.9396926207859171987, 0.3420201433256444545, 0.000000000000000000 ) ) ;
#14605=CARTESIAN_POINT ( 'NONE',  ( -68.99615306438109030, 17.10311908166270456, 15.00000000000006928 ) ) ;
#14611=CARTESIAN_POINT ( 'NONE',  ( -71.24615306438111872, 18.53690796522925055, 15.00000000000006928 ) ) ;
#14615=ORIENTED_EDGE ( 'NONE', *, *, #12121, .F. ) ;
#14621=VECTOR ( 'NONE', #3036, 1000.000000000000000 ) ;
#14623=ORIENTED_EDGE ( 'NONE', *, *, #12257, .T. ) ;
#14628=EDGE_LOOP ( 'NONE', ( #16965, #3202, #8081, #12655 ) ) ;
#14631=AXIS2_PLACEMENT_3D ( 'NONE', #2567, #13780, #6765 ) ;
#14632=FACE_OUTER_BOUND ( 'NONE', #4345, .T. ) ;
#14633=ORIENTED_EDGE ( 'NONE', *, *, #478, .T. ) ;
#14637=VECTOR ( 'NONE', #2611, 1000.000000000000114 ) ;
#14638=EDGE_CURVE ( 'NONE', #11938, #12123, #10437, .T. ) ;
#14653=VERTEX_POINT ( 'NONE', #8950 ) ;
#14656=CARTESIAN_POINT ( 'NONE',  ( -68.99615306438072082, 133.9569029881302811, 15.00000000000006928 ) ) ;
#14657=CARTESIAN_POINT ( 'NONE',  ( -71.24615306438070661, 187.7866419848965052, 15.00000000000006928 ) ) ;
#14658=LINE ( 'NONE', #3166, #2830 ) ;
#14659=ORIENTED_EDGE ( 'NONE', *, *, #7916, .T. ) ;
#14662=LINE ( 'NONE', #17549, #13512 ) ;
#14664=AXIS2_PLACEMENT_3D ( 'NONE', #10907, #15185, #3785 ) ;
#14672=ORIENTED_EDGE ( 'NONE', *, *, #10980, .T. ) ;
#14674=AXIS2_PLACEMENT_3D ( 'NONE', #112, #14424, #7314 ) ;
#14675=LINE ( 'NONE', #11607, #13290 ) ;
#14676=CARTESIAN_POINT ( 'NONE',  ( -71.24615306438109030, 28.85055665456373575, -167.1454815528550739 ) ) ;
#14678=FACE_OUTER_BOUND ( 'NONE', #2941, .T. ) ;
#14680=LINE ( 'NONE', #13297, #12729 ) ;
#14692=ORIENTED_EDGE ( 'NONE', *, *, #349, .F. ) ;
#14693=VECTOR ( 'NONE', #4339, 1000.000000000000000 ) ;
#14696=EDGE_CURVE ( 'NONE', #9888, #3197, #13343, .T. ) ;
#14697=PLANE ( 'NONE',  #8136 ) ;
#14700=AXIS2_PLACEMENT_3D ( 'NONE', #15579, #12594, #11286 ) ;
#14704=DIRECTION ( 'NONE',  ( 0.000000000000000000, 1.000000000000000000, 0.000000000000000000 ) ) ;
#14706=VERTEX_POINT ( 'NONE', #12998 ) ;
#14708=EDGE_LOOP ( 'NONE', ( #17997, #3324, #13396, #15830 ) ) ;
#14713=VECTOR ( 'NONE', #17398, 1000.000000000000000 ) ;
#14714=EDGE_LOOP ( 'NONE', ( #817, #1136, #9475, #14822 ) ) ;
#14715=DIRECTION ( 'NONE',  ( 0.9396926207859157554, 0.3420201433256481738, 4.890320548438487362E-16 ) ) ;
#14719=FACE_OUTER_BOUND ( 'NONE', #16602, .T. ) ;
#14720=DIRECTION ( 'NONE',  ( -0.9396926207859171987, 0.3420201433256445100, -4.890320548438495251E-16 ) ) ;
#14724=AXIS2_PLACEMENT_3D ( 'NONE', #6702, #4274, #11389 ) ;
#14725=VECTOR ( 'NONE', #16348, 1000.000000000000114 ) ;
#14726=DIRECTION ( 'NONE',  ( 0.3420201433256854218, 0.9396926207859023217, -0.000000000000000000 ) ) ;
#14727=LINE ( 'NONE', #4633, #3334 ) ;
#14729=EDGE_CURVE ( 'NONE', #15101, #8820, #8777, .T. ) ;
#14733=ORIENTED_EDGE ( 'NONE', *, *, #6772, .T. ) ;
#14734=EDGE_CURVE ( 'NONE', #3722, #13457, #17450, .T. ) ;
#14736=ORIENTED_EDGE ( 'NONE', *, *, #17597, .F. ) ;
#14739=EDGE_CURVE ( 'NONE', #3439, #7034, #4640, .T. ) ;
#14743=LINE ( 'NONE', #7375, #16506 ) ;
#14744=CARTESIAN_POINT ( 'NONE',  ( -71.24615306438089135, 85.39922435456371375, -167.1454815528550739 ) ) ;
#14750=PLANE ( 'NONE',  #8743 ) ;
#14761=ADVANCED_FACE ( 'NONE', ( #9494 ), #17627, .T. ) ;
#14765=EDGE_LOOP ( 'NONE', ( #12584, #7747, #6566, #7294 ) ) ;
#14771=LINE ( 'NONE', #750, #737 ) ;
#14773=EDGE_CURVE ( 'NONE', #11278, #15985, #10915, .T. ) ;
#14774=LINE ( 'NONE', #7751, #1032 ) ;
#14775=LINE ( 'NONE', #4405, #14358 ) ;
#14776=CARTESIAN_POINT ( 'NONE',  ( -71.24615306438070661, 141.0590213152292449, 15.00000000000006928 ) ) ;
#14779=CARTESIAN_POINT ( 'NONE',  ( -71.24615306438067819, 145.0894847045637732, -15.00000000000001421 ) ) ;
#14782=ORIENTED_EDGE ( 'NONE', *, *, #7352, .F. ) ;
#14784=FACE_OUTER_BOUND ( 'NONE', #7892, .T. ) ;
#14787=VECTOR ( 'NONE', #11136, 1000.000000000000114 ) ;
#14791=CARTESIAN_POINT ( 'NONE',  ( -71.24615306438076345, 122.2094654152292037, -167.1454815528550739 ) ) ;
#14792=CARTESIAN_POINT ( 'NONE',  ( -71.24615306438063556, 138.8062994045637595, 15.00000000000006928 ) ) ;
#14794=VERTEX_POINT ( 'NONE', #8087 ) ;
#14809=ORIENTED_EDGE ( 'NONE', *, *, #8599, .T. ) ;
#14813=CARTESIAN_POINT ( 'NONE',  ( -68.99615306438070661, 115.1073470881302256, 15.00000000000006928 ) ) ;
#14819=ORIENTED_EDGE ( 'NONE', *, *, #12965, .T. ) ;
#14820=CARTESIAN_POINT ( 'NONE',  ( -68.99615306438089135, 79.93497208166267853, 15.00000000000006928 ) ) ;
#14822=ORIENTED_EDGE ( 'NONE', *, *, #14312, .F. ) ;
#14825=ORIENTED_EDGE ( 'NONE', *, *, #14871, .T. ) ;
#14826=EDGE_CURVE ( 'NONE', #14359, #10700, #10710, .T. ) ;
#14830=VERTEX_POINT ( 'NONE', #6303 ) ;
#14833=( LENGTH_UNIT ( ) NAMED_UNIT ( * ) SI_UNIT ( .MILLI., .METRE. ) );
#14834=CARTESIAN_POINT ( 'NONE',  ( -71.24615306438100504, 53.09442711522921599, -167.1454815528550739 ) ) ;
#14835=DIRECTION ( 'NONE',  ( 0.000000000000000000, 0.000000000000000000, 1.000000000000000000 ) ) ;
#14837=CARTESIAN_POINT ( 'NONE',  ( -71.24615306438106188, 34.24487121522926003, -15.00000000000001421 ) ) ;
#14838=CARTESIAN_POINT ( 'NONE',  ( -68.99615306438097662, 61.08541618166268705, -167.1454815528550739 ) ) ;
#14842=VERTEX_POINT ( 'NONE', #13529 ) ;
#14843=LINE ( 'NONE', #6227, #736 ) ;
#14844=DIRECTION ( 'NONE',  ( 0.9396926207859084279, 0.3420201433256686574, 4.890320548438448905E-16 ) ) ;
#14845=EDGE_CURVE ( 'NONE', #16693, #9789, #714, .T. ) ;
#14855=EDGE_CURVE ( 'NONE', #9751, #10505, #14008, .T. ) ;
#14857=FACE_OUTER_BOUND ( 'NONE', #18106, .T. ) ;
#14858=LINE ( 'NONE', #9079, #5798 ) ;
#14859=PLANE ( 'NONE',  #2704 ) ;
#14860=LINE ( 'NONE', #5037, #16876 ) ;
#14866=PLANE ( 'NONE',  #2701 ) ;
#14868=ORIENTED_EDGE ( 'NONE', *, *, #5364, .T. ) ;
#14870=CARTESIAN_POINT ( 'NONE',  ( -68.99615306438067819, 142.7668250816626596, 15.00000000000006928 ) ) ;
#14871=EDGE_CURVE ( 'NONE', #13777, #12432, #14105, .T. ) ;
#14874=VECTOR ( 'NONE', #6185, 1000.000000000000000 ) ;
#14880=DIRECTION ( 'NONE',  ( -0.9396926207859084279, 0.3420201433256686574, -4.890320548438448905E-16 ) ) ;
#14881=DIRECTION ( 'NONE',  ( 0.9396926207859069846, 0.3420201433256723766, 0.000000000000000000 ) ) ;
#14882=ORIENTED_EDGE ( 'NONE', *, *, #10634, .F. ) ;
#14884=CARTESIAN_POINT ( 'NONE',  ( -71.24615306438091977, 75.08557566522922855, 15.00000000000006928 ) ) ;
#14885=VERTEX_POINT ( 'NONE', #8495 ) ;
#14886=VECTOR ( 'NONE', #10858, 1000.000000000000000 ) ;
#14889=DIRECTION ( 'NONE',  ( 0.000000000000000000, 0.000000000000000000, 1.000000000000000000 ) ) ;
#14892=DIRECTION ( 'NONE',  ( 1.000000000000000000, 0.000000000000000000, 0.000000000000000000 ) ) ;
#14893=ORIENTED_EDGE ( 'NONE', *, *, #7820, .F. ) ;
#14894=CARTESIAN_POINT ( 'NONE',  ( -68.99615306438070661, 130.8153103381302742, -15.00000000000001421 ) ) ;
#14895=ORIENTED_EDGE ( 'NONE', *, *, #8712, .F. ) ;
#14897=ORIENTED_EDGE ( 'NONE', *, *, #17156, .T. ) ;
#14898=EDGE_LOOP ( 'NONE', ( #14122, #12202, #564, #3713 ) ) ;
#14910=ORIENTED_EDGE ( 'NONE', *, *, #9022, .F. ) ;
#14912=VECTOR ( 'NONE', #1782, 1000.000000000000227 ) ;
#14913=CARTESIAN_POINT ( 'NONE',  ( -68.99615306438089135, 67.36860148166267948, 15.00000000000006928 ) ) ;
#14916=VECTOR ( 'NONE', #1873, 1000.000000000000000 ) ;
#14923=DIRECTION ( 'NONE',  ( 0.9396926207859084279, 0.3420201433256686574, -1.086737899652989892E-16 ) ) ;
#14927=CARTESIAN_POINT ( 'NONE',  ( -71.24615306438063556, 141.9478920545637948, 15.00000000000006928 ) ) ;
#14941=FACE_OUTER_BOUND ( 'NONE', #10689, .T. ) ;
#14942=AXIS2_PLACEMENT_3D ( 'NONE', #12732, #9719, #15425 ) ;
#14943=EDGE_CURVE ( 'NONE', #6219, #10428, #1191, .T. ) ;
#14944=LINE ( 'NONE', #2141, #9094 ) ;
#14946=DIRECTION ( 'NONE',  ( -0.9396926207859084279, 0.3420201433256686574, 1.086737899652989892E-16 ) ) ;
#14949=DIRECTION ( 'NONE',  ( 0.9396926207859084279, 0.3420201433256686574, -1.086737899652989892E-16 ) ) ;
#14950=ORIENTED_EDGE ( 'NONE', *, *, #15877, .T. ) ;
#14956=EDGE_CURVE ( 'NONE', #17628, #5348, #10925, .T. ) ;
#14961=AXIS2_PLACEMENT_3D ( 'NONE', #11188, #9684, #16597 ) ;
#14962=VECTOR ( 'NONE', #17063, 1000.000000000000000 ) ;
#14964=EDGE_CURVE ( 'NONE', #8931, #12366, #13814, .T. ) ;
#14969=DIRECTION ( 'NONE',  ( 0.000000000000000000, 1.000000000000000000, 0.000000000000000000 ) ) ;
#14973=EDGE_CURVE ( 'NONE', #15423, #7166, #11300, .T. ) ;
#14974=ORIENTED_EDGE ( 'NONE', *, *, #13163, .F. ) ;
#14976=LINE ( 'NONE', #9197, #3321 ) ;
#14980=VECTOR ( 'NONE', #10117, 1000.000000000000000 ) ;
#14982=DIRECTION ( 'NONE',  ( 0.000000000000000000, 0.000000000000000000, 1.000000000000000000 ) ) ;
#14983=ORIENTED_EDGE ( 'NONE', *, *, #3198, .T. ) ;
#14984=EDGE_CURVE ( 'NONE', #9065, #13724, #17688, .T. ) ;
#14994=ORIENTED_EDGE ( 'NONE', *, *, #4129, .F. ) ;
#14995=ADVANCED_FACE ( 'NONE', ( #4366 ), #10072, .T. ) ;
#14998=PLANE ( 'NONE',  #15063 ) ;
#15002=ORIENTED_EDGE ( 'NONE', *, *, #1162, .T. ) ;
#15008=DIRECTION ( 'NONE',  ( 0.000000000000000000, 1.000000000000000000, 0.000000000000000000 ) ) ;
#15010=ORIENTED_EDGE ( 'NONE', *, *, #105, .T. ) ;
#15013=ORIENTED_EDGE ( 'NONE', *, *, #8810, .T. ) ;
#15014=DIRECTION ( 'NONE',  ( 0.9396926207859097602, 0.3420201433256649381, 4.890320548438455808E-16 ) ) ;
#15016=ORIENTED_EDGE ( 'NONE', *, *, #3302, .F. ) ;
#15018=VECTOR ( 'NONE', #4327, 1000.000000000000000 ) ;
#15019=DIRECTION ( 'NONE',  ( 0.000000000000000000, 0.000000000000000000, -1.000000000000000000 ) ) ;
#15021=VECTOR ( 'NONE', #5868, 1000.000000000000000 ) ;
#15022=CARTESIAN_POINT ( 'NONE',  ( -71.24615306438076345, 131.6342433652292243, -167.1454815528550739 ) ) ;
#15024=ORIENTED_EDGE ( 'NONE', *, *, #13167, .T. ) ;
#15026=CARTESIAN_POINT ( 'NONE',  ( -68.99615306438100504, 42.23586028166270978, -167.1454815528550739 ) ) ;
#15029=EDGE_LOOP ( 'NONE', ( #876, #3003, #12587, #11639 ) ) ;
#15030=DIRECTION ( 'NONE',  ( 0.000000000000000000, 0.000000000000000000, 1.000000000000000000 ) ) ;
#15031=CARTESIAN_POINT ( 'NONE',  ( -68.99615306438100504, 48.51904558166270220, 15.00000000000006928 ) ) ;
#15034=DIRECTION ( 'NONE',  ( 0.3420201433256635504, 0.9396926207859103153, -0.000000000000000000 ) ) ;
#15035=VECTOR ( 'NONE', #5032, 1000.000000000000227 ) ;
#15040=ORIENTED_EDGE ( 'NONE', *, *, #4574, .T. ) ;
#15041=DIRECTION ( 'NONE',  ( 0.3420201433256687684, 0.9396926207859084279, -0.000000000000000000 ) ) ;
#15043=ORIENTED_EDGE ( 'NONE', *, *, #11958, .T. ) ;
#15045=LINE ( 'NONE', #8027, #17704 ) ;
#15048=CARTESIAN_POINT ( 'NONE',  ( -71.24615306438070661, 141.0590213152292449, -15.00000000000001421 ) ) ;
#15061=VERTEX_POINT ( 'NONE', #14368 ) ;
#15062=VECTOR ( 'NONE', #15030, 1000.000000000000000 ) ;
#15063=AXIS2_PLACEMENT_3D ( 'NONE', #9576, #6293, #16309 ) ;
#15070=LINE ( 'NONE', #7871, #2157 ) ;
#15071=EDGE_CURVE ( 'NONE', #2577, #6571, #5759, .T. ) ;
#15072=FACE_OUTER_BOUND ( 'NONE', #12171, .T. ) ;
#15079=LINE ( 'NONE', #6274, #7844 ) ;
#15081=ORIENTED_EDGE ( 'NONE', *, *, #4770, .T. ) ;
#15083=DIRECTION ( 'NONE',  ( 0.9396926207859084279, 0.3420201433256686574, 4.890320548438448905E-16 ) ) ;
#15084=VERTEX_POINT ( 'NONE', #11570 ) ;
#15087=EDGE_CURVE ( 'NONE', #1022, #15084, #11488, .T. ) ;
#15094=DIRECTION ( 'NONE',  ( -0.9396926207859097602, 0.3420201433256649381, -4.890320548438455808E-16 ) ) ;
#15096=ORIENTED_EDGE ( 'NONE', *, *, #4667, .F. ) ;
#15097=EDGE_CURVE ( 'NONE', #2613, #5742, #8762, .T. ) ;
#15099=DIRECTION ( 'NONE',  ( 0.000000000000000000, 1.000000000000000000, 0.000000000000000000 ) ) ;
#15100=CARTESIAN_POINT ( 'NONE',  ( -68.99615306438077766, 111.9657544381302330, 15.00000000000006928 ) ) ;
#15101=VERTEX_POINT ( 'NONE', #574 ) ;
#15106=LINE ( 'NONE', #5468, #5946 ) ;
#15111=ORIENTED_EDGE ( 'NONE', *, *, #342, .F. ) ;
#15112=ADVANCED_FACE ( 'NONE', ( #7087 ), #8581, .T. ) ;
#15114=ORIENTED_EDGE ( 'NONE', *, *, #8066, .T. ) ;
#15122=VERTEX_POINT ( 'NONE', #8050 ) ;
#15128=LINE ( 'NONE', #3617, #6387 ) ;
#15129=CARTESIAN_POINT ( 'NONE',  ( -68.99615306438094819, 55.41708673813027985, -167.1454815528550739 ) ) ;
#15135=CARTESIAN_POINT ( 'NONE',  ( -68.99615306438089135, 67.36860148166267948, 15.00000000000006928 ) ) ;
#15138=PLANE ( 'NONE',  #6977 ) ;
#15140=FACE_OUTER_BOUND ( 'NONE', #16788, .T. ) ;
#15145=DIRECTION ( 'NONE',  ( 0.9396926207859171987, 0.3420201433256445100, 4.890320548438495251E-16 ) ) ;
#15146=CARTESIAN_POINT ( 'NONE',  ( -68.99615306438099083, 42.85071613813028790, -15.00000000000001421 ) ) ;
#15149=DIRECTION ( 'NONE',  ( 0.000000000000000000, 1.000000000000000000, 0.000000000000000000 ) ) ;
#15152=VERTEX_POINT ( 'NONE', #5336 ) ;
#15158=DIRECTION ( 'NONE',  ( -0.9396926207859069846, 0.3420201433256723766, 0.000000000000000000 ) ) ;
#15161=ORIENTED_EDGE ( 'NONE', *, *, #14440, .F. ) ;
#15162=CARTESIAN_POINT ( 'NONE',  ( -68.99615306438086293, 89.97460588813027016, -15.00000000000001421 ) ) ;
#15168=VECTOR ( 'NONE', #11451, 1000.000000000000227 ) ;
#15171=ORIENTED_EDGE ( 'NONE', *, *, #17249, .T. ) ;
#15176=DIRECTION ( 'NONE',  ( 0.3420201433256444545, -0.9396926207859171987, 0.000000000000000000 ) ) ;
#15177=LINE ( 'NONE', #2576, #14421 ) ;
#15181=EDGE_CURVE ( 'NONE', #15061, #4999, #13771, .T. ) ;
#15182=DIRECTION ( 'NONE',  ( 0.000000000000000000, 0.000000000000000000, 1.000000000000000000 ) ) ;
#15183=EDGE_LOOP ( 'NONE', ( #22, #3728, #15838, #915 ) ) ;
#15185=DIRECTION ( 'NONE',  ( 0.3420201433256649937, -0.9396926207859097602, 0.000000000000000000 ) ) ;
#15187=VERTEX_POINT ( 'NONE', #17872 ) ;
#15191=LINE ( 'NONE', #3976, #172 ) ;
#15192=VECTOR ( 'NONE', #9092, 1000.000000000000000 ) ;
#15195=DIRECTION ( 'NONE',  ( -0.9396926207859084279, 0.3420201433256686574, 1.086737899652989892E-16 ) ) ;
#15200=EDGE_CURVE ( 'NONE', #8291, #10484, #10683, .T. ) ;
#15201=ORIENTED_EDGE ( 'NONE', *, *, #7104, .T. ) ;
#15205=VECTOR ( 'NONE', #4489, 1000.000000000000000 ) ;
#15208=EDGE_LOOP ( 'NONE', ( #15314, #7595, #2174, #585 ) ) ;
#15213=CARTESIAN_POINT ( 'NONE',  ( -68.99615306438077766, 114.4924912316626688, -167.1454815528550739 ) ) ;
#15214=ADVANCED_FACE ( 'NONE', ( #15072 ), #7782, .T. ) ;
#15218=LINE ( 'NONE', #9238, #16863 ) ;
#15222=EDGE_CURVE ( 'NONE', #11183, #10943, #12382, .T. ) ;
#15229=DIRECTION ( 'NONE',  ( -0.9396926207859083169, 0.3420201433256687129, 0.000000000000000000 ) ) ;
#15236=CARTESIAN_POINT ( 'NONE',  ( -71.24615306438067819, 145.0894847045637732, -167.1454815528550739 ) ) ;
#15244=CARTESIAN_POINT ( 'NONE',  ( -71.24615306438120399, -0.3126479347707321610, -167.1454815528550739 ) ) ;
#15252=UNCERTAINTY_MEASURE_WITH_UNIT (LENGTH_MEASURE( 1.000000000000000082E-05 ), #14833, 'distance_accuracy_value', 'NONE');
#15256=CARTESIAN_POINT ( 'NONE',  ( -71.24615306438114715, 12.25372266522925457, 15.00000000000006928 ) ) ;
#15257=DIRECTION ( 'NONE',  ( 1.000000000000000000, 0.000000000000000000, 0.000000000000000000 ) ) ;
#15258=PLANE ( 'NONE',  #95 ) ;
#15262=CARTESIAN_POINT ( 'NONE',  ( -71.24615306438094819, 65.66079771522920794, -15.00000000000001421 ) ) ;
#15264=LINE ( 'NONE', #4949, #14725 ) ;
#15267=CARTESIAN_POINT ( 'NONE',  ( -71.24615306438106188, 34.24487121522926003, -15.00000000000001421 ) ) ;
#15274=EDGE_CURVE ( 'NONE', #11154, #1345, #5436, .T. ) ;
#15278=FACE_OUTER_BOUND ( 'NONE', #3478, .T. ) ;
#15279=CARTESIAN_POINT ( 'NONE',  ( -71.24615306438086293, 94.82400230456377699, -167.1454815528550739 ) ) ;
#15286=LINE ( 'NONE', #9579, #2727 ) ;
#15294=LINE ( 'NONE', #8483, #4608 ) ;
#15300=EDGE_LOOP ( 'NONE', ( #15487, #7615, #16472, #9389 ) ) ;
#15302=CARTESIAN_POINT ( 'NONE',  ( -68.99615306438089135, 83.07656473166271383, -15.00000000000001421 ) ) ;
#15304=DIRECTION ( 'NONE',  ( 0.000000000000000000, 0.000000000000000000, -1.000000000000000000 ) ) ;
#15305=EDGE_LOOP ( 'NONE', ( #7971, #10212, #7368, #664 ) ) ;
#15306=EDGE_CURVE ( 'NONE', #17985, #14706, #16853, .T. ) ;
#15309=VECTOR ( 'NONE', #406, 1000.000000000000000 ) ;
#15312=CARTESIAN_POINT ( 'NONE',  ( -71.24615306438080609, 116.8151508545637114, -167.1454815528550739 ) ) ;
#15313=DIRECTION ( 'NONE',  ( -0.9396926207859171987, 0.3420201433256445100, -4.890320548438495251E-16 ) ) ;
#15314=ORIENTED_EDGE ( 'NONE', *, *, #16346, .F. ) ;
#15315=DIRECTION ( 'NONE',  ( -0.9396926207859069846, 0.3420201433256723766, 0.000000000000000000 ) ) ;
#15318=CARTESIAN_POINT ( 'NONE',  ( -71.24615306438114715, 9.112130015229229940, 15.00000000000006928 ) ) ;
#15324=EDGE_CURVE ( 'NONE', #3332, #6312, #8257, .T. ) ;
#15325=VECTOR ( 'NONE', #9445, 1000.000000000000227 ) ;
#15328=DIRECTION ( 'NONE',  ( 0.9396926207859078728, 0.3420201433256701007, 0.000000000000000000 ) ) ;
#15334=EDGE_CURVE ( 'NONE', #8291, #3371, #14332, .T. ) ;
#15339=EDGE_CURVE ( 'NONE', #10505, #7990, #15541, .T. ) ;
#15343=ORIENTED_EDGE ( 'NONE', *, *, #11815, .F. ) ;
#15344=PLANE ( 'NONE',  #15650 ) ;
#15345=VECTOR ( 'NONE', #17338, 1000.000000000000227 ) ;
#15348=ORIENTED_EDGE ( 'NONE', *, *, #10420, .T. ) ;
#15353=EDGE_LOOP ( 'NONE', ( #6584, #15024, #1196, #14895 ) ) ;
#15354=VECTOR ( 'NONE', #852, 1000.000000000000000 ) ;
#15355=EDGE_CURVE ( 'NONE', #9827, #11230, #13965, .T. ) ;
#15356=EDGE_CURVE ( 'NONE', #16762, #7430, #18262, .T. ) ;
#15359=VECTOR ( 'NONE', #13962, 1000.000000000000000 ) ;
#15360=FACE_OUTER_BOUND ( 'NONE', #744, .T. ) ;
#15363=DIRECTION ( 'NONE',  ( -0.9396926207859158664, 0.3420201433256481738, 1.086737899652998397E-16 ) ) ;
#15364=CARTESIAN_POINT ( 'NONE',  ( -68.99615306438117557, 1.395155831662692192, 15.00000000000006928 ) ) ;
#15365=PLANE ( 'NONE',  #5125 ) ;
#15368=FACE_OUTER_BOUND ( 'NONE', #10977, .T. ) ;
#15371=ORIENTED_EDGE ( 'NONE', *, *, #3198, .F. ) ;
#15375=VECTOR ( 'NONE', #8193, 1000.000000000000000 ) ;
#15376=AXIS2_PLACEMENT_3D ( 'NONE', #15501, #11217, #7002 ) ;
#15377=VECTOR ( 'NONE', #15182, 1000.000000000000000 ) ;
#15379=VECTOR ( 'NONE', #5969, 1000.000000000000000 ) ;
#15382=ORIENTED_EDGE ( 'NONE', *, *, #1707, .T. ) ;
#15386=VECTOR ( 'NONE', #16404, 1000.000000000000114 ) ;
#15393=DIRECTION ( 'NONE',  ( 0.000000000000000000, 1.000000000000000000, 0.000000000000000000 ) ) ;
#15394=CARTESIAN_POINT ( 'NONE',  ( -71.24615306438094819, 65.66079771522920794, -167.1454815528550739 ) ) ;
#15397=FACE_OUTER_BOUND ( 'NONE', #10356, .T. ) ;
#15400=ORIENTED_EDGE ( 'NONE', *, *, #16993, .F. ) ;
#15402=VECTOR ( 'NONE', #846, 1000.000000000000000 ) ;
#15404=CARTESIAN_POINT ( 'NONE',  ( -68.99615306438111872, 20.24471173166267235, -15.00000000000001421 ) ) ;
#15405=VECTOR ( 'NONE', #8302, 1000.000000000000000 ) ;
#15406=ORIENTED_EDGE ( 'NONE', *, *, #9786, .T. ) ;
#15408=ORIENTED_EDGE ( 'NONE', *, *, #2186, .T. ) ;
#15409=CARTESIAN_POINT ( 'NONE',  ( -70.27900850916093134, -47.21335801510345220, -15.00000000000001599 ) ) ;
#15411=ORIENTED_EDGE ( 'NONE', *, *, #1943, .F. ) ;
#15415=PLANE ( 'NONE',  #18048 ) ;
#15416=ORIENTED_EDGE ( 'NONE', *, *, #17516, .T. ) ;
#15417=LINE ( 'NONE', #2603, #17052 ) ;
#15421=CARTESIAN_POINT ( 'NONE',  ( -68.99615306438117557, 2.010011688130281193, -167.1454815528550739 ) ) ;
#15423=VERTEX_POINT ( 'NONE', #9760 ) ;
#15424=DIRECTION ( 'NONE',  ( 0.3420201433256481738, 0.9396926207859158664, -0.000000000000000000 ) ) ;
#15425=DIRECTION ( 'NONE',  ( 0.000000000000000000, 0.000000000000000000, -1.000000000000000000 ) ) ;
#15430=EDGE_CURVE ( 'NONE', #11979, #8996, #12845, .T. ) ;
#15432=LINE ( 'NONE', #6819, #14196 ) ;
#15440=VERTEX_POINT ( 'NONE', #109 ) ;
#15443=FACE_OUTER_BOUND ( 'NONE', #7808, .T. ) ;
#15445=CARTESIAN_POINT ( 'NONE',  ( -71.24615306438079188, 110.5319655545637403, -15.00000000000001421 ) ) ;
#15446=CARTESIAN_POINT ( 'NONE',  ( -71.24615306438114715, 13.14259340456377956, -167.1454815528550739 ) ) ;
#15447=ORIENTED_EDGE ( 'NONE', *, *, #8714, .F. ) ;
#15448=ORIENTED_EDGE ( 'NONE', *, *, #1499, .F. ) ;
#15453=CARTESIAN_POINT ( 'NONE',  ( -71.24615306438109030, 31.10327856522923540, -15.00000000000001421 ) ) ;
#15454=LINE ( 'NONE', #14050, #8458 ) ;
#15462=CARTESIAN_POINT ( 'NONE',  ( -68.99615306438082030, 99.39938383813029077, -15.00000000000001421 ) ) ;
#15463=ORIENTED_EDGE ( 'NONE', *, *, #16899, .T. ) ;
#15469=DIRECTION ( 'NONE',  ( 0.000000000000000000, 0.000000000000000000, 1.000000000000000000 ) ) ;
#15470=ORIENTED_EDGE ( 'NONE', *, *, #14696, .T. ) ;
#15471=EDGE_CURVE ( 'NONE', #11293, #16643, #8986, .T. ) ;
#15474=DIRECTION ( 'NONE',  ( 0.000000000000000000, 0.000000000000000000, 1.000000000000000000 ) ) ;
#15475=DIRECTION ( 'NONE',  ( 1.000000000000000000, 0.000000000000000000, 0.000000000000000000 ) ) ;
#15477=ORIENTED_EDGE ( 'NONE', *, *, #10526, .F. ) ;
#15478=CARTESIAN_POINT ( 'NONE',  ( -68.99615306438077766, 114.4924912316626688, -15.00000000000001421 ) ) ;
#15482=DIRECTION ( 'NONE',  ( 0.000000000000000000, 0.000000000000000000, -1.000000000000000000 ) ) ;
#15484=ORIENTED_EDGE ( 'NONE', *, *, #2752, .F. ) ;
#15487=ORIENTED_EDGE ( 'NONE', *, *, #11005, .F. ) ;
#15490=ORIENTED_EDGE ( 'NONE', *, *, #7806, .F. ) ;
#15493=DIRECTION ( 'NONE',  ( 0.000000000000000000, 1.000000000000000000, 0.000000000000000000 ) ) ;
#15495=CARTESIAN_POINT ( 'NONE',  ( -71.24615306438094819, 65.66079771522920794, 15.00000000000006928 ) ) ;
#15498=LINE ( 'NONE', #9797, #8512 ) ;
#15501=CARTESIAN_POINT ( 'NONE',  ( -71.24615306438100504, 50.84170520456370923, -167.1454815528550739 ) ) ;
#15504=CARTESIAN_POINT ( 'NONE',  ( -68.99615306438072082, 130.2004544816626890, -15.00000000000001421 ) ) ;
#15505=PLANE ( 'NONE',  #6010 ) ;
#15507=CARTESIAN_POINT ( 'NONE',  ( -68.99615306438094819, 64.22700883166265839, -15.00000000000001421 ) ) ;
#15508=PLANE ( 'NONE',  #18490 ) ;
#15511=ORIENTED_EDGE ( 'NONE', *, *, #17156, .F. ) ;
#15515=EDGE_CURVE ( 'NONE', #2577, #1230, #10116, .T. ) ;
#15516=EDGE_LOOP ( 'NONE', ( #3778, #1760, #17983, #6574 ) ) ;
#15519=CARTESIAN_POINT ( 'NONE',  ( -71.24615306438109030, 27.96168591522921076, 15.00000000000006928 ) ) ;
#15520=VERTEX_POINT ( 'NONE', #3096 ) ;
#15524=CARTESIAN_POINT ( 'NONE',  ( -71.24615306438079188, 112.7846874652292399, 15.00000000000006928 ) ) ;
#15525=PRODUCT_DEFINITION_SHAPE ( 'NONE', 'NONE',  #11622 ) ;
#15527=ADVANCED_FACE ( 'NONE', ( #16000 ), #474, .T. ) ;
#15533=DIRECTION ( 'NONE',  ( 0.000000000000000000, 0.000000000000000000, 1.000000000000000000 ) ) ;
#15536=ORIENTED_EDGE ( 'NONE', *, *, #10100, .T. ) ;
#15541=LINE ( 'NONE', #15364, #2376 ) ;
#15543=DIRECTION ( 'NONE',  ( 1.000000000000000000, 0.000000000000000000, 0.000000000000000000 ) ) ;
#15544=ORIENTED_EDGE ( 'NONE', *, *, #13858, .F. ) ;
#15545=EDGE_CURVE ( 'NONE', #14830, #11545, #14775, .T. ) ;
#15548=EDGE_CURVE ( 'NONE', #10355, #18436, #15819, .T. ) ;
#15551=ORIENTED_EDGE ( 'NONE', *, *, #2516, .F. ) ;
#15553=SHAPE_REPRESENTATION ( 'Gear Rack', ( #16217 ), #11478 ) ;
#15555=VECTOR ( 'NONE', #8309, 1000.000000000000114 ) ;
#15561=EDGE_CURVE ( 'NONE', #455, #2538, #5890, .T. ) ;
#15567=CARTESIAN_POINT ( 'NONE',  ( -68.99615306438089135, 79.93497208166267853, -167.1454815528550739 ) ) ;
#15568=ORIENTED_EDGE ( 'NONE', *, *, #5207, .F. ) ;
#15572=CARTESIAN_POINT ( 'NONE',  ( -71.24615306438091977, 71.94398301522919326, -167.1454815528550739 ) ) ;
#15577=DIRECTION ( 'NONE',  ( 1.000000000000000000, 0.000000000000000000, 0.000000000000000000 ) ) ;
#15579=CARTESIAN_POINT ( 'NONE',  ( -68.99615306438086293, 89.35975003166268493, -167.1454815528550739 ) ) ;
#15585=ORIENTED_EDGE ( 'NONE', *, *, #6042, .T. ) ;
#15586=ADVANCED_FACE ( 'NONE', ( #8131 ), #14859, .T. ) ;
#15589=CARTESIAN_POINT ( 'NONE',  ( -68.99615306438067819, 142.7668250816626596, 15.00000000000006928 ) ) ;
#15591=ORIENTED_EDGE ( 'NONE', *, *, #4310, .T. ) ;
#15592=VECTOR ( 'NONE', #8613, 1000.000000000000114 ) ;
#15593=AXIS2_PLACEMENT_3D ( 'NONE', #11611, #17395, #4586 ) ;
#15600=LINE ( 'NONE', #2598, #16387 ) ;
#15604=VECTOR ( 'NONE', #6485, 1000.000000000000114 ) ;
#15605=DIRECTION ( 'NONE',  ( -0.9396926207859022107, 0.3420201433256853663, -4.890320548438415379E-16 ) ) ;
#15607=CARTESIAN_POINT ( 'NONE',  ( -68.99615306438076345, 99.39938383813026235, 15.00000000000006928 ) ) ;
#15608=ORIENTED_EDGE ( 'NONE', *, *, #6372, .T. ) ;
#15609=AXIS2_PLACEMENT_3D ( 'NONE', #16500, #13424, #515 ) ;
#15611=CARTESIAN_POINT ( 'NONE',  ( -71.24615306438080609, 116.8151508545637114, -15.00000000000001421 ) ) ;
#15612=LINE ( 'NONE', #2799, #8916 ) ;
#15614=DIRECTION ( 'NONE',  ( 0.000000000000000000, 1.000000000000000000, 0.000000000000000000 ) ) ;
#15617=AXIS2_PLACEMENT_3D ( 'NONE', #17187, #8945, #15778 ) ;
#15618=CARTESIAN_POINT ( 'NONE',  ( -71.24615306438080609, 110.5319655545637403, -167.1454815528550739 ) ) ;
#15619=VERTEX_POINT ( 'NONE', #13467 ) ;
#15621=VECTOR ( 'NONE', #16932, 1000.000000000000114 ) ;
#15629=LINE ( 'NONE', #4209, #11432 ) ;
#15631=VECTOR ( 'NONE', #789, 1000.000000000000000 ) ;
#15634=ADVANCED_FACE ( 'NONE', ( #16442 ), #3461, .T. ) ;
#15635=AXIS2_PLACEMENT_3D ( 'NONE', #16949, #4133, #8439 ) ;
#15641=ADVANCED_FACE ( 'NONE', ( #15140 ), #651, .T. ) ;
#15642=ORIENTED_EDGE ( 'NONE', *, *, #2492, .F. ) ;
#15646=CARTESIAN_POINT ( 'NONE',  ( -68.99615306438103346, 33.42593818813029571, 15.00000000000006928 ) ) ;
#15650=AXIS2_PLACEMENT_3D ( 'NONE', #9538, #13753, #6739 ) ;
#15654=CARTESIAN_POINT ( 'NONE',  ( -68.99615306438067819, 143.3816809381303585, -167.1454815528550739 ) ) ;
#15661=VECTOR ( 'NONE', #4175, 1000.000000000000000 ) ;
#15662=AXIS2_PLACEMENT_3D ( 'NONE', #8092, #18119, #12425 ) ;
#15666=LINE ( 'NONE', #12863, #5197 ) ;
#15667=CARTESIAN_POINT ( 'NONE',  ( -68.99615306438069240, 137.0984956381303164, -15.00000000000001421 ) ) ;
#15670=CARTESIAN_POINT ( 'NONE',  ( -71.24615306438103346, 46.81124181522922356, 15.00000000000006928 ) ) ;
#15671=FACE_OUTER_BOUND ( 'NONE', #7467, .T. ) ;
#15672=ORIENTED_EDGE ( 'NONE', *, *, #1269, .T. ) ;
#15674=CARTESIAN_POINT ( 'NONE',  ( -68.99615306438077766, 123.9172691816626610, -15.00000000000001421 ) ) ;
#15675=DIRECTION ( 'NONE',  ( 0.000000000000000000, 0.000000000000000000, 1.000000000000000000 ) ) ;
#15678=VECTOR ( 'NONE', #13394, 1000.000000000000000 ) ;
#15681=ORIENTED_EDGE ( 'NONE', *, *, #8192, .F. ) ;
#15683=ORIENTED_EDGE ( 'NONE', *, *, #17376, .F. ) ;
#15687=ORIENTED_EDGE ( 'NONE', *, *, #16175, .F. ) ;
#15689=EDGE_CURVE ( 'NONE', #14192, #4281, #9351, .T. ) ;
#15690=EDGE_CURVE ( 'NONE', #16809, #5572, #2323, .T. ) ;
#15696=DIRECTION ( 'NONE',  ( 0.000000000000000000, 1.000000000000000000, 0.000000000000000000 ) ) ;
#15699=DIRECTION ( 'NONE',  ( 0.9396926207859084279, 0.3420201433256686574, -1.086737899652989892E-16 ) ) ;
#15702=VERTEX_POINT ( 'NONE', #10845 ) ;
#15705=LINE ( 'NONE', #3230, #8441 ) ;
#15711=DIRECTION ( 'NONE',  ( 0.000000000000000000, 0.000000000000000000, 1.000000000000000000 ) ) ;
#15712=DIRECTION ( 'NONE',  ( 1.000000000000000000, 0.000000000000000000, 0.000000000000000000 ) ) ;
#15717=ORIENTED_EDGE ( 'NONE', *, *, #5847, .T. ) ;
#15718=EDGE_CURVE ( 'NONE', #14794, #14048, #5317, .T. ) ;
#15721=AXIS2_PLACEMENT_3D ( 'NONE', #4849, #3184, #650 ) ;
#15723=FACE_OUTER_BOUND ( 'NONE', #11336, .T. ) ;
#15724=FACE_OUTER_BOUND ( 'NONE', #8903, .T. ) ;
#15726=CARTESIAN_POINT ( 'NONE',  ( -71.24615306438100504, 53.98329785456373742, 15.00000000000006928 ) ) ;
#15731=CARTESIAN_POINT ( 'NONE',  ( -71.24615306438080609, 107.3903729045637192, -167.1454815528550739 ) ) ;
#15734=CARTESIAN_POINT ( 'NONE',  ( -68.99615306438111872, 13.96152643166267993, 15.00000000000006928 ) ) ;
#15735=ORIENTED_EDGE ( 'NONE', *, *, #1275, .T. ) ;
#15739=PLANE ( 'NONE',  #8641 ) ;
#15743=DIRECTION ( 'NONE',  ( 0.3420201433256686574, 0.9396926207859084279, -0.000000000000000000 ) ) ;
#15745=DIRECTION ( 'NONE',  ( 0.000000000000000000, 0.000000000000000000, 1.000000000000000000 ) ) ;
#15750=VERTEX_POINT ( 'NONE', #15726 ) ;
#15751=DIRECTION ( 'NONE',  ( 1.000000000000000000, 0.000000000000000000, 0.000000000000000000 ) ) ;
#15757=EDGE_LOOP ( 'NONE', ( #4370, #923, #16626, #7157 ) ) ;
#15763=VERTEX_POINT ( 'NONE', #11036 ) ;
#15774=CARTESIAN_POINT ( 'NONE',  ( -68.99615306438076345, 111.9657544381302330, -15.00000000000001421 ) ) ;
#15778=DIRECTION ( 'NONE',  ( 1.000000000000000000, 0.000000000000000000, 5.204170427930409450E-16 ) ) ;
#15779=LINE ( 'NONE', #4374, #16176 ) ;
#15780=ORIENTED_EDGE ( 'NONE', *, *, #15087, .F. ) ;
#15781=EDGE_CURVE ( 'NONE', #6312, #10938, #13943, .T. ) ;
#15782=EDGE_CURVE ( 'NONE', #7810, #5163, #6919, .T. ) ;
#15787=VERTEX_POINT ( 'NONE', #12820 ) ;
#15788=ORIENTED_EDGE ( 'NONE', *, *, #17249, .F. ) ;
#15791=CARTESIAN_POINT ( 'NONE',  ( -71.24615306438100504, 53.98329785456373742, -15.00000000000001421 ) ) ;
#15794=DIRECTION ( 'NONE',  ( 0.000000000000000000, 0.000000000000000000, 1.000000000000000000 ) ) ;
#15795=EDGE_CURVE ( 'NONE', #4091, #6648, #1322, .T. ) ;
#15802=FACE_OUTER_BOUND ( 'NONE', #341, .T. ) ;
#15803=ORIENTED_EDGE ( 'NONE', *, *, #6478, .F. ) ;
#15807=LINE ( 'NONE', #1330, #599 ) ;
#15808=VERTEX_POINT ( 'NONE', #12750 ) ;
#15810=DIRECTION ( 'NONE',  ( 0.000000000000000000, 0.000000000000000000, 1.000000000000000000 ) ) ;
#15814=EDGE_LOOP ( 'NONE', ( #3343, #17696, #17758, #3385 ) ) ;
#15815=DIRECTION ( 'NONE',  ( -0.9396926207859093161, 0.3420201433256661594, 1.086737899652990878E-16 ) ) ;
#15819=LINE ( 'NONE', #17567, #7469 ) ;
#15821=VERTEX_POINT ( 'NONE', #17111 ) ;
#15823=LINE ( 'NONE', #15462, #13491 ) ;
#15824=ORIENTED_EDGE ( 'NONE', *, *, #10197, .F. ) ;
#15830=ORIENTED_EDGE ( 'NONE', *, *, #11316, .F. ) ;
#15832=ORIENTED_EDGE ( 'NONE', *, *, #10520, .F. ) ;
#15833=VECTOR ( 'NONE', #1427, 1000.000000000000000 ) ;
#15838=ORIENTED_EDGE ( 'NONE', *, *, #587, .T. ) ;
#15840=CARTESIAN_POINT ( 'NONE',  ( -71.24615306438080609, 109.6430948152292189, -15.00000000000001421 ) ) ;
#15843=ORIENTED_EDGE ( 'NONE', *, *, #5376, .T. ) ;
#15852=STYLED_ITEM('',(#18545),#6144);
#15859=CARTESIAN_POINT ( 'NONE',  ( -71.24615306438091977, 78.22716831522920700, 15.00000000000006928 ) ) ;
#15860=CARTESIAN_POINT ( 'NONE',  ( -71.24615306438080609, 106.5015021652292404, -15.00000000000001421 ) ) ;
#15862=VERTEX_POINT ( 'NONE', #13093 ) ;
#15864=LINE ( 'NONE', #14472, #2770 ) ;
#15866=ORIENTED_EDGE ( 'NONE', *, *, #9492, .T. ) ;
#15868=LINE ( 'NONE', #1566, #2845 ) ;
#15871=AXIS2_PLACEMENT_3D ( 'NONE', #14010, #12619, #4368 ) ;
#15873=ORIENTED_EDGE ( 'NONE', *, *, #12121, .T. ) ;
#15874=ADVANCED_FACE ( 'NONE', ( #11857 ), #6131, .T. ) ;
#15876=VECTOR ( 'NONE', #12674, 1000.000000000000000 ) ;
#15877=EDGE_CURVE ( 'NONE', #3544, #7512, #8692, .T. ) ;
#15879=DIRECTION ( 'NONE',  ( 0.3420201433256686574, -0.9396926207859084279, 0.000000000000000000 ) ) ;
#15881=DIRECTION ( 'NONE',  ( 0.9396926207859110924, 0.3420201433256611634, 0.000000000000000000 ) ) ;
#15883=PLANE ( 'NONE',  #12423 ) ;
#15889=CARTESIAN_POINT ( 'NONE',  ( -71.24615306438084872, 75.97444640456379261, 15.00000000000006928 ) ) ;
#15892=ADVANCED_FACE ( 'NONE', ( #16144 ), #17546, .T. ) ;
#15894=CARTESIAN_POINT ( 'NONE',  ( -68.99615306438094819, 52.27549408813023746, -167.1454815528550739 ) ) ;
#15896=VERTEX_POINT ( 'NONE', #3333 ) ;
#15897=ORIENTED_EDGE ( 'NONE', *, *, #3135, .T. ) ;
#15901=ORIENTED_EDGE ( 'NONE', *, *, #13628, .F. ) ;
#15906=CARTESIAN_POINT ( 'NONE',  ( -71.24615306438111872, 18.53690796522925055, -15.00000000000001421 ) ) ;
#15909=DIRECTION ( 'NONE',  ( 0.000000000000000000, 0.000000000000000000, 1.000000000000000000 ) ) ;
#15911=VERTEX_POINT ( 'NONE', #8965 ) ;
#15916=VECTOR ( 'NONE', #8846, 1000.000000000000114 ) ;
#15917=LINE ( 'NONE', #3107, #7185 ) ;
#15919=CARTESIAN_POINT ( 'NONE',  ( -71.24615306438080609, 104.2487802545637408, -167.1454815528550739 ) ) ;
#15922=EDGE_LOOP ( 'NONE', ( #6636, #7720, #17310, #12255 ) ) ;
#15924=VECTOR ( 'NONE', #14969, 1000.000000000000000 ) ;
#15928=VECTOR ( 'NONE', #6525, 1000.000000000000000 ) ;
#15929=DIRECTION ( 'NONE',  ( 0.9396926207859084279, 0.3420201433256686574, 4.890320548438448905E-16 ) ) ;
#15930=DIRECTION ( 'NONE',  ( 0.9396926207859064295, 0.3420201433256737089, -1.086737899652987550E-16 ) ) ;
#15934=CARTESIAN_POINT ( 'NONE',  ( -71.24615306438080609, 104.2487802545637408, -167.1454815528550739 ) ) ;
#15935=CARTESIAN_POINT ( 'NONE',  ( -68.99615306438076345, 124.5321250381302747, -15.00000000000001421 ) ) ;
#15936=CARTESIAN_POINT ( 'NONE',  ( -68.99615306438072082, 133.3420471316626958, -15.00000000000001421 ) ) ;
#15940=ORIENTED_EDGE ( 'NONE', *, *, #1968, .F. ) ;
#15941=VECTOR ( 'NONE', #10069, 1000.000000000000000 ) ;
#15943=ORIENTED_EDGE ( 'NONE', *, *, #8487, .F. ) ;
#15944=VERTEX_POINT ( 'NONE', #4556 ) ;
#15948=VERTEX_POINT ( 'NONE', #4467 ) ;
#15949=VECTOR ( 'NONE', #16241, 1000.000000000000000 ) ;
#15950=CARTESIAN_POINT ( 'NONE',  ( -68.99615306438070661, 136.4836397816626743, -167.1454815528550739 ) ) ;
#15951=CARTESIAN_POINT ( 'NONE',  ( -71.24615306438076345, 122.2094654152292037, -167.1454815528550739 ) ) ;
#15954=DIRECTION ( 'NONE',  ( 0.9396926207859097602, 0.3420201433256649381, 4.890320548438455808E-16 ) ) ;
#15957=CARTESIAN_POINT ( 'NONE',  ( -68.99615306438111872, 7.678341131662685726, -15.00000000000001421 ) ) ;
#15963=VECTOR ( 'NONE', #18031, 999.9999999999998863 ) ;
#15965=VECTOR ( 'NONE', #15954, 1000.000000000000114 ) ;
#15968=VERTEX_POINT ( 'NONE', #13269 ) ;
#15974=DIRECTION ( 'NONE',  ( 1.000000000000000000, 0.000000000000000000, 0.000000000000000000 ) ) ;
#15978=VECTOR ( 'NONE', #2529, 1000.000000000000114 ) ;
#15981=VECTOR ( 'NONE', #8126, 1000.000000000000000 ) ;
#15984=LINE ( 'NONE', #4836, #1222 ) ;
#15985=VERTEX_POINT ( 'NONE', #6043 ) ;
#15986=EDGE_CURVE ( 'NONE', #1839, #4587, #1848, .T. ) ;
#15987=CARTESIAN_POINT ( 'NONE',  ( -71.24615306438083451, 97.07672421522921979, 15.00000000000006928 ) ) ;
#15988=VERTEX_POINT ( 'NONE', #16419 ) ;
#15993=VERTEX_POINT ( 'NONE', #12145 ) ;
#15995=DIRECTION ( 'NONE',  ( -0.9396926207859103153, 0.3420201433256635504, 1.086737899652991987E-16 ) ) ;
#15996=ADVANCED_FACE ( 'NONE', ( #3808 ), #3610, .T. ) ;
#15998=LINE ( 'NONE', #13466, #16555 ) ;
#16000=FACE_OUTER_BOUND ( 'NONE', #6413, .T. ) ;
#16004=FACE_OUTER_BOUND ( 'NONE', #842, .T. ) ;
#16005=CARTESIAN_POINT ( 'NONE',  ( -68.99615306438100504, 39.70912348813028103, -15.00000000000001421 ) ) ;
#16006=ORIENTED_EDGE ( 'NONE', *, *, #15324, .F. ) ;
#16011=VERTEX_POINT ( 'NONE', #5106 ) ;
#16015=EDGE_CURVE ( 'NONE', #9102, #8996, #17746, .T. ) ;
#16024=DIRECTION ( 'NONE',  ( 0.000000000000000000, 0.000000000000000000, 1.000000000000000000 ) ) ;
#16026=ORIENTED_EDGE ( 'NONE', *, *, #17728, .T. ) ;
#16029=EDGE_CURVE ( 'NONE', #14653, #10695, #13640, .T. ) ;
#16030=CARTESIAN_POINT ( 'NONE',  ( -68.99615306438070661, 136.4836397816626743, 15.00000000000006928 ) ) ;
#16032=VERTEX_POINT ( 'NONE', #5208 ) ;
#16035=EDGE_LOOP ( 'NONE', ( #8585, #776, #2290, #11868 ) ) ;
#16039=ORIENTED_EDGE ( 'NONE', *, *, #5511, .T. ) ;
#16040=DIRECTION ( 'NONE',  ( 0.000000000000000000, 1.000000000000000000, 0.000000000000000000 ) ) ;
#16044=CARTESIAN_POINT ( 'NONE',  ( -94.45685920050698314, -2.213358015103445098, 15.00000000000006928 ) ) ;
#16045=DIRECTION ( 'NONE',  ( 0.9396926207859084279, 0.3420201433256686574, -1.086737899652989892E-16 ) ) ;
#16046=EDGE_LOOP ( 'NONE', ( #15161, #4663, #17344, #17154 ) ) ;
#16048=VERTEX_POINT ( 'NONE', #16331 ) ;
#16052=DIRECTION ( 'NONE',  ( -0.9396926207859097602, 0.3420201433256649937, 0.000000000000000000 ) ) ;
#16053=CARTESIAN_POINT ( 'NONE',  ( -68.99615306438103346, 32.81108233166271759, -167.1454815528550739 ) ) ;
#16054=LINE ( 'NONE', #4927, #15949 ) ;
#16058=LINE ( 'NONE', #4731, #9730 ) ;
#16066=EDGE_CURVE ( 'NONE', #9970, #5754, #13544, .T. ) ;
#16075=CARTESIAN_POINT ( 'NONE',  ( -71.24615306438104767, 38.27533460456375991, -15.00000000000001421 ) ) ;
#16076=CARTESIAN_POINT ( 'NONE',  ( -71.24615306438103346, 40.52805651522925245, -167.1454815528550739 ) ) ;
#16077=VERTEX_POINT ( 'NONE', #731 ) ;
#16078=CARTESIAN_POINT ( 'NONE',  ( -68.99615306438082030, 80.54982793813024955, 15.00000000000006928 ) ) ;
#16079=CARTESIAN_POINT ( 'NONE',  ( -71.24615306438082030, 85.39922435456374217, 15.00000000000006928 ) ) ;
#16082=VERTEX_POINT ( 'NONE', #6506 ) ;
#16083=CARTESIAN_POINT ( 'NONE',  ( -70.27900850916093134, -47.21335801510345220, -15.00000000000001599 ) ) ;
#16087=CARTESIAN_POINT ( 'NONE',  ( -68.99615306438072082, 139.6252324316626812, -167.1454815528550739 ) ) ;
#16089=DIRECTION ( 'NONE',  ( 0.000000000000000000, 1.000000000000000000, 0.000000000000000000 ) ) ;
#16090=DIRECTION ( 'NONE',  ( 0.000000000000000000, 0.000000000000000000, 1.000000000000000000 ) ) ;
#16097=DIRECTION ( 'NONE',  ( 0.000000000000000000, 0.000000000000000000, -1.000000000000000000 ) ) ;
#16103=LINE ( 'NONE', #9019, #3234 ) ;
#16104=ORIENTED_EDGE ( 'NONE', *, *, #459, .T. ) ;
#16106=EDGE_CURVE ( 'NONE', #10354, #1317, #3432, .T. ) ;
#16109=ORIENTED_EDGE ( 'NONE', *, *, #4784, .T. ) ;
#16112=CARTESIAN_POINT ( 'NONE',  ( -68.99615306438109030, 17.10311908166270811, -15.00000000000001421 ) ) ;
#16116=EDGE_CURVE ( 'NONE', #10339, #15944, #9604, .T. ) ;
#16118=LINE ( 'NONE', #15774, #16460 ) ;
#16120=CARTESIAN_POINT ( 'NONE',  ( -68.99615306438101925, 33.42593818813028861, -15.00000000000001421 ) ) ;
#16123=VECTOR ( 'NONE', #12830, 1000.000000000000114 ) ;
#16126=VERTEX_POINT ( 'NONE', #4097 ) ;
#16127=LINE ( 'NONE', #17351, #6717 ) ;
#16129=ORIENTED_EDGE ( 'NONE', *, *, #16155, .T. ) ;
#16130=EDGE_CURVE ( 'NONE', #11213, #8044, #1110, .T. ) ;
#16131=VECTOR ( 'NONE', #12153, 1000.000000000000000 ) ;
#16132=EDGE_CURVE ( 'NONE', #9281, #13601, #18128, .T. ) ;
#16133=VERTEX_POINT ( 'NONE', #11398 ) ;
#16136=ORIENTED_EDGE ( 'NONE', *, *, #15690, .F. ) ;
#16138=DIRECTION ( 'NONE',  ( 0.000000000000000000, 1.000000000000000000, 0.000000000000000000 ) ) ;
#16140=CARTESIAN_POINT ( 'NONE',  ( -68.99615306438077766, 117.6340838816626899, -167.1454815528550739 ) ) ;
#16142=ORIENTED_EDGE ( 'NONE', *, *, #6030, .F. ) ;
#16144=FACE_OUTER_BOUND ( 'NONE', #7897, .T. ) ;
#16145=FACE_OUTER_BOUND ( 'NONE', #6122, .T. ) ;
#16151=VECTOR ( 'NONE', #2096, 1000.000000000000000 ) ;
#16152=EDGE_CURVE ( 'NONE', #6934, #14227, #1197, .T. ) ;
#16155=EDGE_CURVE ( 'NONE', #15948, #7142, #8502, .T. ) ;
#16157=ORIENTED_EDGE ( 'NONE', *, *, #7406, .F. ) ;
#16163=CARTESIAN_POINT ( 'NONE',  ( -68.99615306438097662, 61.08541618166268705, -15.00000000000001421 ) ) ;
#16169=EDGE_CURVE ( 'NONE', #8923, #18088, #2792, .T. ) ;
#16172=DIRECTION ( 'NONE',  ( 0.9396926207859171987, 0.3420201433256445100, 4.890320548438495251E-16 ) ) ;
#16173=CARTESIAN_POINT ( 'NONE',  ( -68.99615306438106188, 26.52789703166272162, -15.00000000000001421 ) ) ;
#16175=EDGE_CURVE ( 'NONE', #13941, #5735, #14209, .T. ) ;
#16176=VECTOR ( 'NONE', #13156, 1000.000000000000000 ) ;
#16182=AXIS2_PLACEMENT_3D ( 'NONE', #10323, #1534, #17237 ) ;
#16184=CARTESIAN_POINT ( 'NONE',  ( -68.99615306438089135, 86.21815738166266385, 15.00000000000006928 ) ) ;
#16188=VECTOR ( 'NONE', #4516, 1000.000000000000114 ) ;
#16189=DIRECTION ( 'NONE',  ( -0.9396926207859084279, 0.3420201433256686574, 0.000000000000000000 ) ) ;
#16191=CARTESIAN_POINT ( 'NONE',  ( -71.24615306438114715, 16.28418605456380419, 15.00000000000006928 ) ) ;
#16196=PLANE ( 'NONE',  #6857 ) ;
#16198=AXIS2_PLACEMENT_3D ( 'NONE', #7687, #13489, #6460 ) ;
#16200=CARTESIAN_POINT ( 'NONE',  ( -71.24615306438067819, 144.2006139652292518, -167.1454815528550739 ) ) ;
#16204=EDGE_LOOP ( 'NONE', ( #17537, #13568, #13930, #1836 ) ) ;
#16212=EDGE_CURVE ( 'NONE', #7430, #12040, #15417, .T. ) ;
#16213=FACE_OUTER_BOUND ( 'NONE', #16873, .T. ) ;
#16215=ADVANCED_FACE ( 'NONE', ( #17091 ), #12802, .T. ) ;
#16217=AXIS2_PLACEMENT_3D ( 'NONE', #5781, #6037, #8961 ) ;
#16219=ORIENTED_EDGE ( 'NONE', *, *, #15782, .F. ) ;
#16221=DIRECTION ( 'NONE',  ( 0.000000000000000000, 1.000000000000000000, 0.000000000000000000 ) ) ;
#16222=DIRECTION ( 'NONE',  ( 0.000000000000000000, 1.000000000000000000, 0.000000000000000000 ) ) ;
#16224=EDGE_CURVE ( 'NONE', #15944, #16663, #9896, .T. ) ;
#16225=EDGE_CURVE ( 'NONE', #12749, #10207, #7001, .T. ) ;
#16226=DIRECTION ( 'NONE',  ( 1.000000000000000000, 0.000000000000000000, 0.000000000000000000 ) ) ;
#16228=ORIENTED_EDGE ( 'NONE', *, *, #16823, .T. ) ;
#16230=AXIS2_PLACEMENT_3D ( 'NONE', #18517, #5687, #11416 ) ;
#16235=CARTESIAN_POINT ( 'NONE',  ( -71.24615306438091977, 79.11603905456372843, -167.1454815528550739 ) ) ;
#16241=DIRECTION ( 'NONE',  ( 0.000000000000000000, 0.000000000000000000, 1.000000000000000000 ) ) ;
#16249=CARTESIAN_POINT ( 'NONE',  ( -71.24615306438076345, 125.3510580652292248, 15.00000000000006928 ) ) ;
#16251=VECTOR ( 'NONE', #11875, 1000.000000000000000 ) ;
#16252=VECTOR ( 'NONE', #12723, 1000.000000000000000 ) ;
#16254=VECTOR ( 'NONE', #16851, 1000.000000000000114 ) ;
#16257=ORIENTED_EDGE ( 'NONE', *, *, #17940, .F. ) ;
#16259=CARTESIAN_POINT ( 'NONE',  ( -68.99615306438070661, 111.9657544381302046, 15.00000000000006928 ) ) ;
#16262=VERTEX_POINT ( 'NONE', #14556 ) ;
#16264=DIRECTION ( 'NONE',  ( 0.000000000000000000, 0.000000000000000000, 1.000000000000000000 ) ) ;
#16270=CARTESIAN_POINT ( 'NONE',  ( -71.24615306438111872, 19.42577870456376132, -167.1454815528550739 ) ) ;
#16277=DIRECTION ( 'NONE',  ( 0.9396926207859097602, 0.3420201433256649937, -1.086737899652991371E-16 ) ) ;
#16279=CARTESIAN_POINT ( 'NONE',  ( -71.24615306438091977, 75.08557566522922855, -167.1454815528550739 ) ) ;
#16283=EDGE_LOOP ( 'NONE', ( #12601, #2294, #14819, #12244 ) ) ;
#16286=DIRECTION ( 'NONE',  ( 0.9396926207859097602, 0.3420201433256649937, 0.000000000000000000 ) ) ;
#16291=VECTOR ( 'NONE', #10555, 1000.000000000000114 ) ;
#16294=ORIENTED_EDGE ( 'NONE', *, *, #18288, .T. ) ;
#16296=LINE ( 'NONE', #3288, #3615 ) ;
#16300=CARTESIAN_POINT ( 'NONE',  ( -70.27900850916093134, -47.21335801510345220, -15.00000000000001599 ) ) ;
#16301=EDGE_LOOP ( 'NONE', ( #10184, #17266, #8213, #198 ) ) ;
#16302=CARTESIAN_POINT ( 'NONE',  ( -71.24615306438094819, 69.69126110456375045, -15.00000000000001421 ) ) ;
#16305=DIRECTION ( 'NONE',  ( 0.000000000000000000, 0.000000000000000000, -1.000000000000000000 ) ) ;
#16307=ORIENTED_EDGE ( 'NONE', *, *, #11873, .T. ) ;
#16309=DIRECTION ( 'NONE',  ( 0.000000000000000000, 0.000000000000000000, -1.000000000000000000 ) ) ;
#16311=ADVANCED_FACE ( 'NONE', ( #6114 ), #3229, .T. ) ;
#16312=LINE ( 'NONE', #13336, #5706 ) ;
#16314=LINE ( 'NONE', #4992, #5731 ) ;
#16316=ORIENTED_EDGE ( 'NONE', *, *, #13340, .F. ) ;
#16317=DIRECTION ( 'NONE',  ( 0.000000000000000000, 1.000000000000000000, 0.000000000000000000 ) ) ;
#16319=VERTEX_POINT ( 'NONE', #11576 ) ;
#16320=ADVANCED_FACE ( 'NONE', ( #14292 ), #1734, .T. ) ;
#16321=ORIENTED_EDGE ( 'NONE', *, *, #10197, .T. ) ;
#16323=LINE ( 'NONE', #10922, #17424 ) ;
#16325=CARTESIAN_POINT ( 'NONE',  ( -71.24615306438070661, 147.3422066152292871, -167.1454815528550739 ) ) ;
#16326=CARTESIAN_POINT ( 'NONE',  ( -71.24615306438109030, 25.70896400456376796, 15.00000000000006928 ) ) ;
#16328=VERTEX_POINT ( 'NONE', #2886 ) ;
#16329=EDGE_CURVE ( 'NONE', #1178, #6902, #7437, .T. ) ;
#16330=ADVANCED_FACE ( 'NONE', ( #13153 ), #1468, .T. ) ;
#16331=CARTESIAN_POINT ( 'NONE',  ( -68.99615306438100504, 39.09426763166271002, -15.00000000000001421 ) ) ;
#16332=CARTESIAN_POINT ( 'NONE',  ( -68.99615306438100504, 42.23586028166270978, 15.00000000000006928 ) ) ;
#16335=ORIENTED_EDGE ( 'NONE', *, *, #8238, .T. ) ;
#16341=ADVANCED_FACE ( 'NONE', ( #5860 ), #12895, .T. ) ;
#16343=EDGE_LOOP ( 'NONE', ( #1722, #2812, #16109, #11256 ) ) ;
#16346=EDGE_CURVE ( 'NONE', #1716, #12432, #17186, .T. ) ;
#16348=DIRECTION ( 'NONE',  ( -0.9396926207859022107, 0.3420201433256853663, -4.890320548438416365E-16 ) ) ;
#16349=VERTEX_POINT ( 'NONE', #327 ) ;
#16353=EDGE_CURVE ( 'NONE', #8597, #3211, #8768, .T. ) ;
#16354=EDGE_CURVE ( 'NONE', #1460, #14653, #10348, .T. ) ;
#16358=VERTEX_POINT ( 'NONE', #16497 ) ;
#16360=DIRECTION ( 'NONE',  ( 0.000000000000000000, 0.000000000000000000, -1.000000000000000000 ) ) ;
#16363=CARTESIAN_POINT ( 'NONE',  ( -68.99615306438106188, 30.28434553813027108, 15.00000000000006928 ) ) ;
#16364=EDGE_LOOP ( 'NONE', ( #6802, #18197, #14304, #7859 ) ) ;
#16365=VECTOR ( 'NONE', #16578, 1000.000000000000000 ) ;
#16370=LINE ( 'NONE', #770, #82 ) ;
#16372=CARTESIAN_POINT ( 'NONE',  ( -71.24615306438100504, 53.09442711522921599, 15.00000000000006928 ) ) ;
#16375=LINE ( 'NONE', #775, #3629 ) ;
#16381=CARTESIAN_POINT ( 'NONE',  ( -68.99615306438094819, 55.41708673813027985, 15.00000000000006928 ) ) ;
#16385=CARTESIAN_POINT ( 'NONE',  ( -71.24615306438070661, 147.3422066152292871, 15.00000000000006928 ) ) ;
#16387=VECTOR ( 'NONE', #5385, 1000.000000000000000 ) ;
#16388=ORIENTED_EDGE ( 'NONE', *, *, #14845, .F. ) ;
#16389=CARTESIAN_POINT ( 'NONE',  ( -68.99615306438094819, 51.66063823166267355, -167.1454815528550739 ) ) ;
#16399=CARTESIAN_POINT ( 'NONE',  ( -71.24615306438101925, 28.85055665456376062, 15.00000000000006928 ) ) ;
#16402=ORIENTED_EDGE ( 'NONE', *, *, #10821, .F. ) ;
#16404=DIRECTION ( 'NONE',  ( 0.9396926207859148672, 0.3420201433256507273, -1.086737899652997288E-16 ) ) ;
#16407=ORIENTED_EDGE ( 'NONE', *, *, #9280, .F. ) ;
#16408=VECTOR ( 'NONE', #657, 1000.000000000000000 ) ;
#16409=CARTESIAN_POINT ( 'NONE',  ( -68.99615306438099083, 24.00116023813024313, 15.00000000000006928 ) ) ;
#16410=FACE_OUTER_BOUND ( 'NONE', #4215, .T. ) ;
#16413=CARTESIAN_POINT ( 'NONE',  ( -71.24615306438106188, 35.13374195456378146, -15.00000000000001421 ) ) ;
#16414=SHAPE_REPRESENTATION_RELATIONSHIP ( 'NONE' , 'NONE' ,  #15553, #6556 ) ;
#16417=CARTESIAN_POINT ( 'NONE',  ( -68.99615306438072082, 130.2004544816626890, -167.1454815528550739 ) ) ;
#16419=CARTESIAN_POINT ( 'NONE',  ( -68.99615306438086293, 89.35975003166268493, -15.00000000000001421 ) ) ;
#16420=DIRECTION ( 'NONE',  ( 1.000000000000000000, 0.000000000000000000, 0.000000000000000000 ) ) ;
#16427=VECTOR ( 'NONE', #17019, 1000.000000000000000 ) ;
#16428=EDGE_LOOP ( 'NONE', ( #1544, #5638, #11862, #2662 ) ) ;
#16437=ORIENTED_EDGE ( 'NONE', *, *, #10508, .T. ) ;
#16442=FACE_OUTER_BOUND ( 'NONE', #2336, .T. ) ;
#16451=PLANE ( 'NONE',  #9575 ) ;
#16452=ORIENTED_EDGE ( 'NONE', *, *, #8266, .T. ) ;
#16455=CARTESIAN_POINT ( 'NONE',  ( -71.24615306438117557, 2.828944715229236628, -167.1454815528550739 ) ) ;
#16457=EDGE_CURVE ( 'NONE', #16126, #10978, #16312, .T. ) ;
#16458=ADVANCED_FACE ( 'NONE', ( #9036 ), #603, .T. ) ;
#16460=VECTOR ( 'NONE', #11572, 1000.000000000000114 ) ;
#16464=LINE ( 'NONE', #7962, #17106 ) ;
#16472=ORIENTED_EDGE ( 'NONE', *, *, #10065, .T. ) ;
#16478=VECTOR ( 'NONE', #8258, 1000.000000000000000 ) ;
#16481=EDGE_CURVE ( 'NONE', #9020, #12176, #10704, .T. ) ;
#16484=DIRECTION ( 'NONE',  ( 0.000000000000000000, 0.000000000000000000, 1.000000000000000000 ) ) ;
#16486=AXIS2_PLACEMENT_3D ( 'NONE', #9898, #16704, #2795 ) ;
#16489=VECTOR ( 'NONE', #14038, 1000.000000000000000 ) ;
#16491=LINE ( 'NONE', #7894, #15631 ) ;
#16497=CARTESIAN_POINT ( 'NONE',  ( -71.24615306438070661, 141.0590213152292449, 15.00000000000006928 ) ) ;
#16498=ORIENTED_EDGE ( 'NONE', *, *, #13285, .T. ) ;
#16499=DIRECTION ( 'NONE',  ( 0.9396926207859097602, 0.3420201433256649381, 4.890320548438455808E-16 ) ) ;
#16500=CARTESIAN_POINT ( 'NONE',  ( -68.99615306438077766, 111.9657544381302330, -167.1454815528550739 ) ) ;
#16503=LINE ( 'NONE', #6589, #13592 ) ;
#16506=VECTOR ( 'NONE', #11942, 1000.000000000000000 ) ;
#16508=LINE ( 'NONE', #3711, #4307 ) ;
#16526=CARTESIAN_POINT ( 'NONE',  ( -68.99615306438086293, 89.35975003166268493, 15.00000000000006928 ) ) ;
#16527=VERTEX_POINT ( 'NONE', #10801 ) ;
#16541=AXIS2_PLACEMENT_3D ( 'NONE', #5300, #900, #15304 ) ;
#16543=AXIS2_PLACEMENT_3D ( 'NONE', #13869, #5432, #7963 ) ;
#16544=CARTESIAN_POINT ( 'NONE',  ( -71.24615306438103346, 43.66964916522919538, -15.00000000000001421 ) ) ;
#16554=ORIENTED_EDGE ( 'NONE', *, *, #14516, .F. ) ;
#16555=VECTOR ( 'NONE', #11796, 999.9999999999998863 ) ;
#16556=VECTOR ( 'NONE', #16646, 1000.000000000000000 ) ;
#16557=ADVANCED_FACE ( 'NONE', ( #1093 ), #12593, .T. ) ;
#16558=ORIENTED_EDGE ( 'NONE', *, *, #4285, .T. ) ;
#16561=CARTESIAN_POINT ( 'NONE',  ( -68.99615306438072082, 133.3420471316626958, -167.1454815528550739 ) ) ;
#16563=DIRECTION ( 'NONE',  ( 0.3420201433256686574, 0.9396926207859084279, -0.000000000000000000 ) ) ;
#16565=PLANE ( 'NONE',  #354 ) ;
#16568=ADVANCED_FACE ( 'NONE', ( #5185 ), #2668, .T. ) ;
#16569=DIRECTION ( 'NONE',  ( 0.9396926207859110924, 0.3420201433256611634, 0.000000000000000000 ) ) ;
#16571=CARTESIAN_POINT ( 'NONE',  ( -68.99615306438110451, 20.85956758813031087, -15.00000000000001421 ) ) ;
#16573=EDGE_CURVE ( 'NONE', #17232, #6896, #15286, .T. ) ;
#16578=DIRECTION ( 'NONE',  ( 0.000000000000000000, 1.000000000000000000, 0.000000000000000000 ) ) ;
#16584=ADVANCED_FACE ( 'NONE', ( #8183 ), #5282, .T. ) ;
#16587=ADVANCED_FACE ( 'NONE', ( #10993 ), #18395, .T. ) ;
#16588=LINE ( 'NONE', #2659, #5791 ) ;
#16589=DIRECTION ( 'NONE',  ( 0.3420201433256724322, -0.9396926207859070956, 0.000000000000000000 ) ) ;
#16594=ORIENTED_EDGE ( 'NONE', *, *, #6488, .T. ) ;
#16597=DIRECTION ( 'NONE',  ( 0.000000000000000000, 0.000000000000000000, -1.000000000000000000 ) ) ;
#16599=ORIENTED_EDGE ( 'NONE', *, *, #3641, .F. ) ;
#16602=EDGE_LOOP ( 'NONE', ( #228, #6771, #16498, #810 ) ) ;
#16604=DIRECTION ( 'NONE',  ( 0.000000000000000000, 0.000000000000000000, 1.000000000000000000 ) ) ;
#16605=VERTEX_POINT ( 'NONE', #5360 ) ;
#16606=EDGE_CURVE ( 'NONE', #13332, #6219, #8078, .T. ) ;
#16607=CARTESIAN_POINT ( 'NONE',  ( -68.99615306438089135, 86.83301323813024908, -15.00000000000001421 ) ) ;
#16616=CARTESIAN_POINT ( 'NONE',  ( -71.24615306438097662, 59.37761241522920841, -15.00000000000001421 ) ) ;
#16618=DIRECTION ( 'NONE',  ( 0.000000000000000000, 0.000000000000000000, 1.000000000000000000 ) ) ;
#16621=DIRECTION ( 'NONE',  ( 0.000000000000000000, 1.000000000000000000, 0.000000000000000000 ) ) ;
#16623=ORIENTED_EDGE ( 'NONE', *, *, #10289, .F. ) ;
#16624=LINE ( 'NONE', #3817, #7472 ) ;
#16626=ORIENTED_EDGE ( 'NONE', *, *, #6068, .T. ) ;
#16627=ORIENTED_EDGE ( 'NONE', *, *, #11562, .F. ) ;
#16628=PLANE ( 'NONE',  #18020 ) ;
#16636=ORIENTED_EDGE ( 'NONE', *, *, #16457, .T. ) ;
#16638=CARTESIAN_POINT ( 'NONE',  ( -71.24615306438109030, 31.10327856522923540, -15.00000000000001421 ) ) ;
#16639=ORIENTED_EDGE ( 'NONE', *, *, #15222, .F. ) ;
#16642=PLANE ( 'NONE',  #17561 ) ;
#16643=VERTEX_POINT ( 'NONE', #4078 ) ;
#16646=DIRECTION ( 'NONE',  ( 0.000000000000000000, 0.000000000000000000, 1.000000000000000000 ) ) ;
#16647=DIRECTION ( 'NONE',  ( 0.3420201433256518375, -0.9396926207859145341, 0.000000000000000000 ) ) ;
#16648=CARTESIAN_POINT ( 'NONE',  ( -68.99615306438086293, 92.50134268166266338, -167.1454815528550739 ) ) ;
#16649=CARTESIAN_POINT ( 'NONE',  ( -71.24615306438076345, 119.9567435045637609, -167.1454815528550739 ) ) ;
#16651=CARTESIAN_POINT ( 'NONE',  ( -68.99615306438097662, 61.08541618166268705, 15.00000000000006928 ) ) ;
#16652=VERTEX_POINT ( 'NONE', #984 ) ;
#16656=ORIENTED_EDGE ( 'NONE', *, *, #2999, .T. ) ;
#16657=CARTESIAN_POINT ( 'NONE',  ( -68.99615306438083451, 101.9261206316626698, -15.00000000000001421 ) ) ;
#16658=DIRECTION ( 'NONE',  ( 1.000000000000000000, 0.000000000000000000, 0.000000000000000000 ) ) ;
#16661=CARTESIAN_POINT ( 'NONE',  ( -71.24615306438070661, 137.9174286652292096, 15.00000000000006928 ) ) ;
#16663=VERTEX_POINT ( 'NONE', #18292 ) ;
#16665=FACE_OUTER_BOUND ( 'NONE', #12964, .T. ) ;
#16667=PLANE ( 'NONE',  #5189 ) ;
#16670=ORIENTED_EDGE ( 'NONE', *, *, #13978, .T. ) ;
#16671=SHAPE_DEFINITION_REPRESENTATION ( #15525, #15553 ) ;
#16677=CARTESIAN_POINT ( 'NONE',  ( -71.24615306438097662, 60.26648315456372984, -15.00000000000001421 ) ) ;
#16679=ORIENTED_EDGE ( 'NONE', *, *, #12359, .F. ) ;
#16682=CARTESIAN_POINT ( 'NONE',  ( -71.24615306438094819, 69.69126110456375045, 15.00000000000006928 ) ) ;
#16683=ORIENTED_EDGE ( 'NONE', *, *, #11477, .F. ) ;
#16684=EDGE_CURVE ( 'NONE', #6487, #663, #17417, .T. ) ;
#16690=EDGE_CURVE ( 'NONE', #663, #10924, #5910, .T. ) ;
#16692=CARTESIAN_POINT ( 'NONE',  ( -68.99615306438090556, 58.55867938813022988, 15.00000000000006928 ) ) ;
#16693=VERTEX_POINT ( 'NONE', #7248 ) ;
#16695=DIRECTION ( 'NONE',  ( 0.9396926207859145341, 0.3420201433256518930, 4.890320548438480460E-16 ) ) ;
#16697=CARTESIAN_POINT ( 'NONE',  ( -68.99615306438077766, 115.1073470881302541, 15.00000000000006928 ) ) ;
#16699=ORIENTED_EDGE ( 'NONE', *, *, #5576, .F. ) ;
#16700=DIRECTION ( 'NONE',  ( -0.9396926207859084279, 0.3420201433256686574, -4.890320548438448905E-16 ) ) ;
#16704=DIRECTION ( 'NONE',  ( 1.000000000000000000, 0.000000000000000000, 0.000000000000000000 ) ) ;
#16705=LINE ( 'NONE', #7005, #10225 ) ;
#16711=FACE_OUTER_BOUND ( 'NONE', #16343, .T. ) ;
#16717=ORIENTED_EDGE ( 'NONE', *, *, #704, .T. ) ;
#16727=AXIS2_PLACEMENT_3D ( 'NONE', #18047, #6341, #9254 ) ;
#16730=ORIENTED_EDGE ( 'NONE', *, *, #5988, .T. ) ;
#16731=LINE ( 'NONE', #9542, #15402 ) ;
#16734=ORIENTED_EDGE ( 'NONE', *, *, #13392, .F. ) ;
#16735=VECTOR ( 'NONE', #15614, 1000.000000000000000 ) ;
#16744=FACE_OUTER_BOUND ( 'NONE', #6836, .T. ) ;
#16746=DIRECTION ( 'NONE',  ( 0.000000000000000000, 0.000000000000000000, -1.000000000000000000 ) ) ;
#16747=FACE_OUTER_BOUND ( 'NONE', #8888, .T. ) ;
#16759=VECTOR ( 'NONE', #3964, 1000.000000000000000 ) ;
#16762=VERTEX_POINT ( 'NONE', #15840 ) ;
#16763=AXIS2_PLACEMENT_3D ( 'NONE', #1346, #15743, #7054 ) ;
#16766=DIRECTION ( 'NONE',  ( 0.9396926207859092051, 0.3420201433256663259, -1.086737899652990755E-16 ) ) ;
#16767=ORIENTED_EDGE ( 'NONE', *, *, #15200, .F. ) ;
#16770=VECTOR ( 'NONE', #7754, 1000.000000000000000 ) ;
#16775=CARTESIAN_POINT ( 'NONE',  ( -71.24615306438086293, 88.54081700456373483, -167.1454815528550739 ) ) ;
#16781=VERTEX_POINT ( 'NONE', #13130 ) ;
#16787=VECTOR ( 'NONE', #4559, 1000.000000000000000 ) ;
#16788=EDGE_LOOP ( 'NONE', ( #3045, #3647, #7884, #9016 ) ) ;
#16793=PLANE ( 'NONE',  #14724 ) ;
#16801=ORIENTED_EDGE ( 'NONE', *, *, #11656, .T. ) ;
#16803=VECTOR ( 'NONE', #8380, 1000.000000000000000 ) ;
#16804=VECTOR ( 'NONE', #11631, 1000.000000000000000 ) ;
#16805=CARTESIAN_POINT ( 'NONE',  ( -68.99615306438111872, 20.85956758813031797, -167.1454815528550739 ) ) ;
#16808=DIRECTION ( 'NONE',  ( 0.3420201433256661594, 0.9396926207859093161, -0.000000000000000000 ) ) ;
#16809=VERTEX_POINT ( 'NONE', #5744 ) ;
#16818=ORIENTED_EDGE ( 'NONE', *, *, #4361, .F. ) ;
#16819=ADVANCED_FACE ( 'NONE', ( #222 ), #9107, .T. ) ;
#16821=VECTOR ( 'NONE', #16172, 999.9999999999998863 ) ;
#16823=EDGE_CURVE ( 'NONE', #8923, #17556, #10686, .T. ) ;
#16827=LINE ( 'NONE', #9915, #9653 ) ;
#16831=DIRECTION ( 'NONE',  ( 0.000000000000000000, 0.000000000000000000, 1.000000000000000000 ) ) ;
#16851=DIRECTION ( 'NONE',  ( 0.9396926207859144231, 0.3420201433256520041, 4.890320548438480460E-16 ) ) ;
#16852=CARTESIAN_POINT ( 'NONE',  ( -68.99615306438073503, 121.3905323881302962, -15.00000000000001421 ) ) ;
#16853=LINE ( 'NONE', #9841, #12563 ) ;
#16854=LINE ( 'NONE', #16651, #16478 ) ;
#16855=ORIENTED_EDGE ( 'NONE', *, *, #8873, .T. ) ;
#16858=ORIENTED_EDGE ( 'NONE', *, *, #9167, .F. ) ;
#16863=VECTOR ( 'NONE', #3443, 1000.000000000000000 ) ;
#16866=VECTOR ( 'NONE', #11156, 1000.000000000000000 ) ;
#16870=DIRECTION ( 'NONE',  ( 0.000000000000000000, 0.000000000000000000, -1.000000000000000000 ) ) ;
#16871=LINE ( 'NONE', #5734, #7542 ) ;
#16873=EDGE_LOOP ( 'NONE', ( #9267, #1815, #9300, #2591 ) ) ;
#16876=VECTOR ( 'NONE', #4750, 1000.000000000000000 ) ;
#16881=CARTESIAN_POINT ( 'NONE',  ( -68.99615306438097662, 57.94382353166266597, -167.1454815528550739 ) ) ;
#16884=ORIENTED_EDGE ( 'NONE', *, *, #5375, .F. ) ;
#16886=CARTESIAN_POINT ( 'NONE',  ( -68.99615306438077766, 115.1073470881302541, -15.00000000000001421 ) ) ;
#16887=ORIENTED_EDGE ( 'NONE', *, *, #1622, .F. ) ;
#16888=DIRECTION ( 'NONE',  ( 0.000000000000000000, 1.000000000000000000, 0.000000000000000000 ) ) ;
#16891=CARTESIAN_POINT ( 'NONE',  ( -71.24615306438094819, 65.66079771522920794, -15.00000000000001421 ) ) ;
#16895=ORIENTED_EDGE ( 'NONE', *, *, #2892, .F. ) ;
#16897=CARTESIAN_POINT ( 'NONE',  ( -68.99615306438106188, 35.95267498166268894, -15.00000000000001421 ) ) ;
#16899=EDGE_CURVE ( 'NONE', #15122, #10506, #16296, .T. ) ;
#16908=VECTOR ( 'NONE', #5583, 1000.000000000000000 ) ;
#16911=ORIENTED_EDGE ( 'NONE', *, *, #12003, .F. ) ;
#16912=CARTESIAN_POINT ( 'NONE',  ( -68.99615306438091977, 74.26664263813029265, 15.00000000000006928 ) ) ;
#16917=PLANE ( 'NONE',  #8979 ) ;
#16932=DIRECTION ( 'NONE',  ( 0.9396926207859171987, 0.3420201433256444545, -1.086737899652999999E-16 ) ) ;
#16934=EDGE_CURVE ( 'NONE', #2433, #1839, #14976, .T. ) ;
#16935=FACE_OUTER_BOUND ( 'NONE', #13799, .T. ) ;
#16938=EDGE_CURVE ( 'NONE', #11028, #12040, #13320, .T. ) ;
#16944=ORIENTED_EDGE ( 'NONE', *, *, #16130, .T. ) ;
#16948=CARTESIAN_POINT ( 'NONE',  ( -71.24615306438096241, 57.12489050456377271, -15.00000000000001421 ) ) ;
#16949=CARTESIAN_POINT ( 'NONE',  ( -68.99615306438089135, 67.98345733813025049, -167.1454815528550739 ) ) ;
#16954=CARTESIAN_POINT ( 'NONE',  ( -71.24615306438114715, 10.00100075456375492, -15.00000000000001421 ) ) ;
#16955=ORIENTED_EDGE ( 'NONE', *, *, #10945, .T. ) ;
#16956=FACE_OUTER_BOUND ( 'NONE', #12893, .T. ) ;
#16958=ORIENTED_EDGE ( 'NONE', *, *, #922, .T. ) ;
#16964=DIRECTION ( 'NONE',  ( 0.000000000000000000, 0.000000000000000000, 1.000000000000000000 ) ) ;
#16965=ORIENTED_EDGE ( 'NONE', *, *, #10967, .F. ) ;
#16966=ORIENTED_EDGE ( 'NONE', *, *, #12667, .F. ) ;
#16968=CARTESIAN_POINT ( 'NONE',  ( -71.24615306438109030, 24.82009326522924297, -167.1454815528550739 ) ) ;
#16972=CARTESIAN_POINT ( 'NONE',  ( -71.24615306438094819, 68.80239036522922902, -167.1454815528550739 ) ) ;
#16974=DIRECTION ( 'NONE',  ( 1.000000000000000000, 0.000000000000000000, 0.000000000000000000 ) ) ;
#16975=LINE ( 'NONE', #8084, #16803 ) ;
#16976=VERTEX_POINT ( 'NONE', #14317 ) ;
#16977=EDGE_CURVE ( 'NONE', #16762, #11028, #17211, .T. ) ;
#16978=CARTESIAN_POINT ( 'NONE',  ( -71.24615306438089135, 85.39922435456371375, 15.00000000000006928 ) ) ;
#16984=LINE ( 'NONE', #8293, #2821 ) ;
#16988=DIRECTION ( 'NONE',  ( 0.9396926207859171987, 0.3420201433256445100, 4.890320548438495251E-16 ) ) ;
#16989=DIRECTION ( 'NONE',  ( 0.000000000000000000, 1.000000000000000000, 0.000000000000000000 ) ) ;
#16993=EDGE_CURVE ( 'NONE', #7503, #15821, #18081, .T. ) ;
#16996=VECTOR ( 'NONE', #5795, 1000.000000000000000 ) ;
#16998=PLANE ( 'NONE',  #11431 ) ;
#16999=EDGE_LOOP ( 'NONE', ( #3949, #2677, #3123, #16157 ) ) ;
#17000=FACE_OUTER_BOUND ( 'NONE', #2850, .T. ) ;
#17001=CARTESIAN_POINT ( 'NONE',  ( -68.99615306438079188, 105.6825691381303045, -15.00000000000001421 ) ) ;
#17002=CARTESIAN_POINT ( 'NONE',  ( -68.99615306438106188, 23.38630438166269698, -15.00000000000001421 ) ) ;
#17017=CARTESIAN_POINT ( 'NONE',  ( -71.24615306438086293, 94.82400230456377699, -15.00000000000001421 ) ) ;
#17019=DIRECTION ( 'NONE',  ( 0.9396926207859110924, 0.3420201433256612189, -1.086737899652992973E-16 ) ) ;
#17021=ORIENTED_EDGE ( 'NONE', *, *, #12398, .T. ) ;
#17024=AXIS2_PLACEMENT_3D ( 'NONE', #5664, #11392, #4277 ) ;
#17029=CARTESIAN_POINT ( 'NONE',  ( -68.99615306438106188, 29.66948968166269296, -167.1454815528550739 ) ) ;
#17031=AXIS2_PLACEMENT_3D ( 'NONE', #7972, #9562, #1077 ) ;
#17045=EDGE_CURVE ( 'NONE', #5342, #14885, #3763, .T. ) ;
#17047=EDGE_CURVE ( 'NONE', #5572, #18030, #8162, .T. ) ;
#17050=VERTEX_POINT ( 'NONE', #6761 ) ;
#17052=VECTOR ( 'NONE', #8301, 1000.000000000000000 ) ;
#17055=EDGE_CURVE ( 'NONE', #9789, #12932, #12479, .T. ) ;
#17057=LINE ( 'NONE', #3201, #17986 ) ;
#17061=ORIENTED_EDGE ( 'NONE', *, *, #2899, .F. ) ;
#17063=DIRECTION ( 'NONE',  ( 0.000000000000000000, 1.000000000000000000, 0.000000000000000000 ) ) ;
#17064=EDGE_CURVE ( 'NONE', #11474, #1178, #2912, .T. ) ;
#17067=CARTESIAN_POINT ( 'NONE',  ( -71.24615306438111872, 18.53690796522925055, -15.00000000000001421 ) ) ;
#17071=VECTOR ( 'NONE', #3402, 1000.000000000000000 ) ;
#17072=ORIENTED_EDGE ( 'NONE', *, *, #13514, .F. ) ;
#17080=VECTOR ( 'NONE', #11826, 1000.000000000000000 ) ;
#17082=ORIENTED_EDGE ( 'NONE', *, *, #8936, .T. ) ;
#17083=LINE ( 'NONE', #18410, #8494 ) ;
#17087=LINE ( 'NONE', #14288, #2488 ) ;
#17088=CARTESIAN_POINT ( 'NONE',  ( -68.99615306438094819, 71.12504998813029999, -167.1454815528550739 ) ) ;
#17090=VECTOR ( 'NONE', #11842, 1000.000000000000000 ) ;
#17091=FACE_OUTER_BOUND ( 'NONE', #15922, .T. ) ;
#17092=DIRECTION ( 'NONE',  ( -0.9396926207859069846, 0.3420201433256723766, 1.086737899652988166E-16 ) ) ;
#17096=VECTOR ( 'NONE', #5186, 1000.000000000000114 ) ;
#17097=FACE_OUTER_BOUND ( 'NONE', #8899, .T. ) ;
#17098=DIRECTION ( 'NONE',  ( 0.000000000000000000, 0.000000000000000000, 1.000000000000000000 ) ) ;
#17099=DIRECTION ( 'NONE',  ( 1.000000000000000000, 0.000000000000000000, 0.000000000000000000 ) ) ;
#17101=ORIENTED_EDGE ( 'NONE', *, *, #6957, .T. ) ;
#17102=ORIENTED_EDGE ( 'NONE', *, *, #15097, .F. ) ;
#17105=ORIENTED_EDGE ( 'NONE', *, *, #7120, .F. ) ;
#17106=VECTOR ( 'NONE', #2443, 1000.000000000000000 ) ;
#17110=ORIENTED_EDGE ( 'NONE', *, *, #8626, .T. ) ;
#17111=CARTESIAN_POINT ( 'NONE',  ( -68.99615306438120399, -1.746436818337276931, 15.00000000000006928 ) ) ;
#17114=CARTESIAN_POINT ( 'NONE',  ( -71.24615306438120399, 0.5762228045637918239, 15.00000000000006928 ) ) ;
#17117=VECTOR ( 'NONE', #11854, 1000.000000000000000 ) ;
#17120=VECTOR ( 'NONE', #14510, 1000.000000000000000 ) ;
#17123=LINE ( 'NONE', #15734, #3532 ) ;
#17125=ORIENTED_EDGE ( 'NONE', *, *, #14973, .F. ) ;
#17127=CARTESIAN_POINT ( 'NONE',  ( -71.24615306438074924, 126.2399288045637462, -15.00000000000001421 ) ) ;
#17128=CARTESIAN_POINT ( 'NONE',  ( -71.24615306438080609, 103.3599095152292193, -15.00000000000001421 ) ) ;
#17132=DIRECTION ( 'NONE',  ( 0.000000000000000000, 0.000000000000000000, 1.000000000000000000 ) ) ;
#17133=VECTOR ( 'NONE', #13142, 1000.000000000000000 ) ;
#17134=AXIS2_PLACEMENT_3D ( 'NONE', #9726, #2900, #15328 ) ;
#17136=ORIENTED_EDGE ( 'NONE', *, *, #123, .T. ) ;
#17146=VECTOR ( 'NONE', #1108, 1000.000000000000000 ) ;
#17150=DIRECTION ( 'NONE',  ( -0.9396926207859069846, 0.3420201433256723766, -4.890320548438442003E-16 ) ) ;
#17154=ORIENTED_EDGE ( 'NONE', *, *, #17540, .F. ) ;
#17156=EDGE_CURVE ( 'NONE', #15520, #11474, #1950, .T. ) ;
#17157=CARTESIAN_POINT ( 'NONE',  ( -71.24615306438091977, 78.22716831522920700, -15.00000000000001421 ) ) ;
#17160=DIRECTION ( 'NONE',  ( 0.3420201433256507828, -0.9396926207859149782, 0.000000000000000000 ) ) ;
#17165=EDGE_LOOP ( 'NONE', ( #12787, #3818, #16801, #6297 ) ) ;
#17166=DIRECTION ( 'NONE',  ( 0.000000000000000000, 0.000000000000000000, -1.000000000000000000 ) ) ;
#17174=VECTOR ( 'NONE', #16317, 1000.000000000000000 ) ;
#17175=VECTOR ( 'NONE', #1090, 1000.000000000000000 ) ;
#17177=LINE ( 'NONE', #4364, #15941 ) ;
#17185=ORIENTED_EDGE ( 'NONE', *, *, #11126, .F. ) ;
#17186=LINE ( 'NONE', #17346, #7496 ) ;
#17187=CARTESIAN_POINT ( 'NONE',  ( -127.5926225674732279, 47.87487112387803023, 15.00000000000004263 ) ) ;
#17189=ORIENTED_EDGE ( 'NONE', *, *, #4922, .F. ) ;
#17191=VECTOR ( 'NONE', #9176, 1000.000000000000000 ) ;
#17192=VECTOR ( 'NONE', #6214, 1000.000000000000000 ) ;
#17196=EDGE_LOOP ( 'NONE', ( #9039, #18061, #11924, #6146 ) ) ;
#17211=LINE ( 'NONE', #6664, #14098 ) ;
#17213=ORIENTED_EDGE ( 'NONE', *, *, #14638, .F. ) ;
#17218=LINE ( 'NONE', #10113, #9699 ) ;
#17219=DIRECTION ( 'NONE',  ( 0.9396926207859084279, 0.3420201433256686574, -1.086737899652989892E-16 ) ) ;
#17220=DIRECTION ( 'NONE',  ( 0.000000000000000000, 0.000000000000000000, 1.000000000000000000 ) ) ;
#17222=CARTESIAN_POINT ( 'NONE',  ( -71.24615306438089135, 82.25763170456374951, -15.00000000000001421 ) ) ;
#17230=CARTESIAN_POINT ( 'NONE',  ( -71.24615306438079188, 113.6735582045637045, 15.00000000000006928 ) ) ;
#17232=VERTEX_POINT ( 'NONE', #823 ) ;
#17234=CARTESIAN_POINT ( 'NONE',  ( -71.24615306438082030, 82.25763170456377793, 15.00000000000006928 ) ) ;
#17237=DIRECTION ( 'NONE',  ( -0.9396926207859084279, 0.3420201433256686574, 0.000000000000000000 ) ) ;
#17240=VERTEX_POINT ( 'NONE', #7935 ) ;
#17249=EDGE_CURVE ( 'NONE', #5018, #7663, #9235, .T. ) ;
#17257=DIRECTION ( 'NONE',  ( 0.000000000000000000, 0.000000000000000000, 1.000000000000000000 ) ) ;
#17263=CARTESIAN_POINT ( 'NONE',  ( -68.99615306438074924, 120.7756765316626542, -167.1454815528550739 ) ) ;
#17266=ORIENTED_EDGE ( 'NONE', *, *, #12248, .T. ) ;
#17267=LINE ( 'NONE', #10162, #5214 ) ;
#17271=DIRECTION ( 'NONE',  ( 0.000000000000000000, 1.000000000000000000, 0.000000000000000000 ) ) ;
#17272=EDGE_CURVE ( 'NONE', #18002, #5917, #12229, .T. ) ;
#17273=ORIENTED_EDGE ( 'NONE', *, *, #8000, .T. ) ;
#17276=EDGE_CURVE ( 'NONE', #4288, #6911, #1202, .T. ) ;
#17280=PLANE ( 'NONE',  #11742 ) ;
#17284=LINE ( 'NONE', #8528, #11823 ) ;
#17292=ORIENTED_EDGE ( 'NONE', *, *, #11562, .T. ) ;
#17293=FACE_OUTER_BOUND ( 'NONE', #3260, .T. ) ;
#17294=DIRECTION ( 'NONE',  ( 0.000000000000000000, 0.000000000000000000, 1.000000000000000000 ) ) ;
#17297=VERTEX_POINT ( 'NONE', #9805 ) ;
#17307=PLANE ( 'NONE',  #3363 ) ;
#17309=LINE ( 'NONE', #8450, #5363 ) ;
#17310=ORIENTED_EDGE ( 'NONE', *, *, #4315, .T. ) ;
#17314=VECTOR ( 'NONE', #387, 1000.000000000000000 ) ;
#17315=EDGE_CURVE ( 'NONE', #17987, #2873, #16705, .T. ) ;
#17318=LINE ( 'NONE', #11818, #18057 ) ;
#17322=ADVANCED_FACE ( 'NONE', ( #2505 ), #7095, .T. ) ;
#17327=LINE ( 'NONE', #10231, #15916 ) ;
#17328=ORIENTED_EDGE ( 'NONE', *, *, #3441, .F. ) ;
#17333=EDGE_LOOP ( 'NONE', ( #8444, #8169, #17552, #3132 ) ) ;
#17335=ORIENTED_EDGE ( 'NONE', *, *, #5847, .F. ) ;
#17336=VECTOR ( 'NONE', #8800, 1000.000000000000000 ) ;
#17337=VECTOR ( 'NONE', #2697, 1000.000000000000000 ) ;
#17338=DIRECTION ( 'NONE',  ( 0.9396926207859157554, 0.3420201433256481738, 4.890320548438487362E-16 ) ) ;
#17340=DIRECTION ( 'NONE',  ( 0.000000000000000000, 0.000000000000000000, -1.000000000000000000 ) ) ;
#17341=LINE ( 'NONE', #1553, #18203 ) ;
#17342=LINE ( 'NONE', #12988, #9003 ) ;
#17344=ORIENTED_EDGE ( 'NONE', *, *, #7352, .T. ) ;
#17345=ADVANCED_FACE ( 'NONE', ( #13929 ), #15505, .T. ) ;
#17346=CARTESIAN_POINT ( 'NONE',  ( -71.24615306438094819, 66.54966845456371516, -167.1454815528550739 ) ) ;
#17349=ORIENTED_EDGE ( 'NONE', *, *, #5617, .T. ) ;
#17350=VECTOR ( 'NONE', #3127, 1000.000000000000000 ) ;
#17351=CARTESIAN_POINT ( 'NONE',  ( -71.24615306438091977, 75.08557566522922855, -167.1454815528550739 ) ) ;
#17353=AXIS2_PLACEMENT_3D ( 'NONE', #13919, #1107, #11110 ) ;
#17354=ORIENTED_EDGE ( 'NONE', *, *, #12608, .F. ) ;
#17355=ADVANCED_FACE ( 'NONE', ( #8588 ), #2694, .T. ) ;
#17357=ADVANCED_FACE ( 'NONE', ( #8403 ), #4187, .T. ) ;
#17363=CARTESIAN_POINT ( 'NONE',  ( -68.99615306438111872, 14.57638228813026871, -15.00000000000001421 ) ) ;
#17365=ADVANCED_FACE ( 'NONE', ( #11400 ), #16998, .T. ) ;
#17366=EDGE_CURVE ( 'NONE', #4896, #10257, #14727, .T. ) ;
#17368=AXIS2_PLACEMENT_3D ( 'NONE', #17877, #10493, #12186 ) ;
#17370=CARTESIAN_POINT ( 'NONE',  ( -68.99615306438083451, 99.39938383813029077, -167.1454815528550739 ) ) ;
#17376=EDGE_CURVE ( 'NONE', #17860, #3439, #69, .T. ) ;
#17378=DIRECTION ( 'NONE',  ( 0.3420201433256689905, 0.9396926207859084279, -0.000000000000000000 ) ) ;
#17380=ORIENTED_EDGE ( 'NONE', *, *, #16132, .T. ) ;
#17384=VECTOR ( 'NONE', #8032, 1000.000000000000000 ) ;
#17387=VERTEX_POINT ( 'NONE', #11495 ) ;
#17389=CARTESIAN_POINT ( 'NONE',  ( -71.24615306438097662, 62.51920506522922949, -15.00000000000001421 ) ) ;
#17390=DIRECTION ( 'NONE',  ( 0.3420201433256649937, 0.9396926207859097602, -0.000000000000000000 ) ) ;
#17391=FACE_OUTER_BOUND ( 'NONE', #6560, .T. ) ;
#17392=EDGE_CURVE ( 'NONE', #12093, #15619, #15779, .T. ) ;
#17393=VECTOR ( 'NONE', #15094, 1000.000000000000114 ) ;
#17394=CARTESIAN_POINT ( 'NONE',  ( -71.24615306438100504, 49.95283446522918780, -167.1454815528550739 ) ) ;
#17395=DIRECTION ( 'NONE',  ( 1.000000000000000000, 0.000000000000000000, 0.000000000000000000 ) ) ;
#17396=VERTEX_POINT ( 'NONE', #4536 ) ;
#17398=DIRECTION ( 'NONE',  ( 0.000000000000000000, 1.000000000000000000, 0.000000000000000000 ) ) ;
#17403=CARTESIAN_POINT ( 'NONE',  ( -71.24615306438069240, 123.0983361545637393, 15.00000000000006928 ) ) ;
#17411=DIRECTION ( 'NONE',  ( -0.9396926207859022107, 0.3420201433256853663, 1.086737899652982620E-16 ) ) ;
#17413=DIRECTION ( 'NONE',  ( 0.000000000000000000, 0.000000000000000000, 1.000000000000000000 ) ) ;
#17415=ORIENTED_EDGE ( 'NONE', *, *, #9217, .F. ) ;
#17417=LINE ( 'NONE', #15674, #9301 ) ;
#17418=CARTESIAN_POINT ( 'NONE',  ( -68.99615306438077766, 123.9172691816626610, -167.1454815528550739 ) ) ;
#17424=VECTOR ( 'NONE', #7921, 999.9999999999998863 ) ;
#17428=APPLICATION_CONTEXT ( 'automotive_design' ) ;
#17431=LINE ( 'NONE', #4434, #7316 ) ;
#17435=DIRECTION ( 'NONE',  ( 0.3420201433256737644, -0.9396926207859066515, 0.000000000000000000 ) ) ;
#17437=DIRECTION ( 'NONE',  ( 1.000000000000000000, 0.000000000000000000, 0.000000000000000000 ) ) ;
#17439=DIRECTION ( 'NONE',  ( -0.9396926207859097602, 0.3420201433256649381, -4.890320548438455808E-16 ) ) ;
#17442=DIRECTION ( 'NONE',  ( 0.000000000000000000, 0.000000000000000000, -1.000000000000000000 ) ) ;
#17448=DIRECTION ( 'NONE',  ( 0.000000000000000000, 0.000000000000000000, -1.000000000000000000 ) ) ;
#17449=VECTOR ( 'NONE', #825, 1000.000000000000000 ) ;
#17450=LINE ( 'NONE', #4542, #3259 ) ;
#17453=AXIS2_PLACEMENT_3D ( 'NONE', #4224, #5249, #2832 ) ;
#17457=LINE ( 'NONE', #14913, #3099 ) ;
#17458=VECTOR ( 'NONE', #1791, 1000.000000000000000 ) ;
#17459=ORIENTED_EDGE ( 'NONE', *, *, #17850, .F. ) ;
#17462=CARTESIAN_POINT ( 'NONE',  ( -71.24615306438103346, 43.66964916522919538, -167.1454815528550739 ) ) ;
#17468=FACE_OUTER_BOUND ( 'NONE', #15353, .T. ) ;
#17470=DIRECTION ( 'NONE',  ( 1.000000000000000000, 0.000000000000000000, 0.000000000000000000 ) ) ;
#17475=CARTESIAN_POINT ( 'NONE',  ( -71.24615306438086293, 88.54081700456373483, 15.00000000000006928 ) ) ;
#17480=EDGE_CURVE ( 'NONE', #4782, #10561, #13250, .T. ) ;
#17483=CARTESIAN_POINT ( 'NONE',  ( -71.24615306438091977, 79.11603905456372843, -15.00000000000001421 ) ) ;
#17488=LINE ( 'NONE', #14776, #9416 ) ;
#17493=DIRECTION ( 'NONE',  ( 1.000000000000000000, 0.000000000000000000, 0.000000000000000000 ) ) ;
#17494=CARTESIAN_POINT ( 'NONE',  ( -71.24615306438074924, 119.9567435045637609, -15.00000000000001421 ) ) ;
#17496=LINE ( 'NONE', #16173, #14051 ) ;
#17497=VERTEX_POINT ( 'NONE', #246 ) ;
#17516=EDGE_CURVE ( 'NONE', #15187, #17628, #6587, .T. ) ;
#17521=VERTEX_POINT ( 'NONE', #18004 ) ;
#17522=ORIENTED_EDGE ( 'NONE', *, *, #6295, .T. ) ;
#17523=PLANE ( 'NONE',  #3394 ) ;
#17524=LINE ( 'NONE', #6108, #17133 ) ;
#17525=ORIENTED_EDGE ( 'NONE', *, *, #5699, .T. ) ;
#17526=CARTESIAN_POINT ( 'NONE',  ( -71.24615306438109030, 24.82009326522924297, -167.1454815528550739 ) ) ;
#17528=PLANE ( 'NONE',  #10899 ) ;
#17537=ORIENTED_EDGE ( 'NONE', *, *, #1627, .F. ) ;
#17538=ORIENTED_EDGE ( 'NONE', *, *, #14739, .T. ) ;
#17540=EDGE_CURVE ( 'NONE', #13143, #6193, #5191, .T. ) ;
#17544=FACE_OUTER_BOUND ( 'NONE', #14628, .T. ) ;
#17545=ORIENTED_EDGE ( 'NONE', *, *, #13183, .T. ) ;
#17546=PLANE ( 'NONE',  #11664 ) ;
#17549=CARTESIAN_POINT ( 'NONE',  ( -68.99615306438120399, -1.746436818337276931, -167.1454815528550739 ) ) ;
#17550=VECTOR ( 'NONE', #10609, 1000.000000000000000 ) ;
#17552=ORIENTED_EDGE ( 'NONE', *, *, #10078, .T. ) ;
#17554=VECTOR ( 'NONE', #4871, 1000.000000000000000 ) ;
#17556=VERTEX_POINT ( 'NONE', #7712 ) ;
#17561=AXIS2_PLACEMENT_3D ( 'NONE', #15446, #11151, #9747 ) ;
#17567=CARTESIAN_POINT ( 'NONE',  ( -68.99615306438080609, 105.0677132816627051, -167.1454815528550739 ) ) ;
#17569=DIRECTION ( 'NONE',  ( 0.000000000000000000, 0.000000000000000000, 1.000000000000000000 ) ) ;
#17570=EDGE_LOOP ( 'NONE', ( #895, #6544, #10333, #127 ) ) ;
#17572=ADVANCED_FACE ( 'NONE', ( #10707 ), #4908, .T. ) ;
#17586=CARTESIAN_POINT ( 'NONE',  ( -68.99615306438066398, 133.9569029881302527, 15.00000000000006928 ) ) ;
#17587=ORIENTED_EDGE ( 'NONE', *, *, #13922, .F. ) ;
#17589=CARTESIAN_POINT ( 'NONE',  ( -68.99615306438086293, 89.97460588813027016, -167.1454815528550739 ) ) ;
#17593=CARTESIAN_POINT ( 'NONE',  ( -68.99615306438117557, 5.151604338130305827, -167.1454815528550739 ) ) ;
#17597=EDGE_CURVE ( 'NONE', #7613, #6728, #7812, .T. ) ;
#17598=EDGE_LOOP ( 'NONE', ( #15096, #953, #4555, #10021 ) ) ;
#17606=VECTOR ( 'NONE', #1003, 1000.000000000000000 ) ;
#17607=EDGE_LOOP ( 'NONE', ( #7222, #15717, #5596, #3945 ) ) ;
#17613=DIRECTION ( 'NONE',  ( 0.000000000000000000, 0.000000000000000000, 1.000000000000000000 ) ) ;
#17615=DIRECTION ( 'NONE',  ( 1.000000000000000000, 0.000000000000000000, 0.000000000000000000 ) ) ;
#17616=ORIENTED_EDGE ( 'NONE', *, *, #3091, .T. ) ;
#17624=ORIENTED_EDGE ( 'NONE', *, *, #16899, .F. ) ;
#17627=PLANE ( 'NONE',  #1484 ) ;
#17628=VERTEX_POINT ( 'NONE', #13703 ) ;
#17631=VECTOR ( 'NONE', #12434, 1000.000000000000000 ) ;
#17638=PLANE ( 'NONE',  #7326 ) ;
#17640=DIRECTION ( 'NONE',  ( 0.000000000000000000, 0.000000000000000000, -1.000000000000000000 ) ) ;
#17641=ORIENTED_EDGE ( 'NONE', *, *, #8896, .T. ) ;
#17644=CARTESIAN_POINT ( 'NONE',  ( -68.99615306438104767, 27.14275288813030329, -15.00000000000001421 ) ) ;
#17645=DIRECTION ( 'NONE',  ( 0.000000000000000000, 0.000000000000000000, 1.000000000000000000 ) ) ;
#17649=VECTOR ( 'NONE', #165, 1000.000000000000000 ) ;
#17652=ORIENTED_EDGE ( 'NONE', *, *, #13629, .F. ) ;
#17654=LINE ( 'NONE', #4841, #3903 ) ;
#17656=EDGE_LOOP ( 'NONE', ( #8456, #11546, #7371, #4176 ) ) ;
#17659=ORIENTED_EDGE ( 'NONE', *, *, #18190, .F. ) ;
#17666=CARTESIAN_POINT ( 'NONE',  ( -71.24615306438079188, 101.1071876045637339, 15.00000000000006928 ) ) ;
#17672=ORIENTED_EDGE ( 'NONE', *, *, #10752, .T. ) ;
#17675=VECTOR ( 'NONE', #5693, 1000.000000000000000 ) ;
#17676=CARTESIAN_POINT ( 'NONE',  ( -71.24615306438106188, 37.38646386522923137, 15.00000000000006928 ) ) ;
#17677=ORIENTED_EDGE ( 'NONE', *, *, #11107, .T. ) ;
#17679=PRODUCT_DEFINITION_CONTEXT ( 'detailed design', #17428, 'design' ) ;
#17680=VECTOR ( 'NONE', #5905, 1000.000000000000000 ) ;
#17682=CARTESIAN_POINT ( 'NONE',  ( -68.99615306438100504, 39.09426763166271002, -167.1454815528550739 ) ) ;
#17683=DIRECTION ( 'NONE',  ( 0.9396926207859145341, 0.3420201433256518375, 0.000000000000000000 ) ) ;
#17684=CARTESIAN_POINT ( 'NONE',  ( -71.24615306438103346, 47.70011255456374499, -167.1454815528550739 ) ) ;
#17685=LINE ( 'NONE', #4967, #686 ) ;
#17688=LINE ( 'NONE', #6265, #6859 ) ;
#17694=CARTESIAN_POINT ( 'NONE',  ( -68.99615306438089135, 67.98345733813025049, -15.00000000000001421 ) ) ;
#17695=LINE ( 'NONE', #9199, #675 ) ;
#17696=ORIENTED_EDGE ( 'NONE', *, *, #4083, .T. ) ;
#17698=CARTESIAN_POINT ( 'NONE',  ( -68.99615306438084872, 89.97460588813027016, -15.00000000000001421 ) ) ;
#17703=EDGE_LOOP ( 'NONE', ( #4889, #3587, #16388, #7388 ) ) ;
#17704=VECTOR ( 'NONE', #9252, 1000.000000000000000 ) ;
#17707=VERTEX_POINT ( 'NONE', #988 ) ;
#17710=PLANE ( 'NONE',  #12704 ) ;
#17719=EDGE_CURVE ( 'NONE', #17860, #14842, #9690, .T. ) ;
#17724=LINE ( 'NONE', #427, #17090 ) ;
#17727=CARTESIAN_POINT ( 'NONE',  ( -71.24615306438106188, 38.27533460456375281, -15.00000000000001421 ) ) ;
#17728=EDGE_CURVE ( 'NONE', #16781, #3544, #16975, .T. ) ;
#17731=VERTEX_POINT ( 'NONE', #16682 ) ;
#17738=ORIENTED_EDGE ( 'NONE', *, *, #5739, .T. ) ;
#17741=ORIENTED_EDGE ( 'NONE', *, *, #716, .T. ) ;
#17743=LINE ( 'NONE', #4925, #9666 ) ;
#17746=LINE ( 'NONE', #13354, #6583 ) ;
#17747=DIRECTION ( 'NONE',  ( 1.000000000000000000, 0.000000000000000000, 0.000000000000000000 ) ) ;
#17751=VECTOR ( 'NONE', #4268, 1000.000000000000000 ) ;
#17753=VECTOR ( 'NONE', #13697, 1000.000000000000000 ) ;
#17755=LINE ( 'NONE', #13549, #9399 ) ;
#17758=ORIENTED_EDGE ( 'NONE', *, *, #6856, .T. ) ;
#17761=ORIENTED_EDGE ( 'NONE', *, *, #6767, .F. ) ;
#17767=CARTESIAN_POINT ( 'NONE',  ( -71.24615306438070661, 187.7866419848965052, -15.00000000000001421 ) ) ;
#17768=FACE_OUTER_BOUND ( 'NONE', #2133, .T. ) ;
#17769=LINE ( 'NONE', #1967, #16251 ) ;
#17770=DIRECTION ( 'NONE',  ( 0.9396926207859084279, 0.3420201433256686574, 0.000000000000000000 ) ) ;
#17775=CARTESIAN_POINT ( 'NONE',  ( -71.24615306438060713, 145.0894847045638016, 15.00000000000006928 ) ) ;
#17776=ORIENTED_EDGE ( 'NONE', *, *, #13630, .F. ) ;
#17777=AXIS2_PLACEMENT_3D ( 'NONE', #11046, #945, #12367 ) ;
#17778=LINE ( 'NONE', #17861, #6421 ) ;
#17780=VERTEX_POINT ( 'NONE', #16886 ) ;
#17789=VECTOR ( 'NONE', #18423, 1000.000000000000114 ) ;
#17797=ORIENTED_EDGE ( 'NONE', *, *, #17836, .T. ) ;
#17800=CARTESIAN_POINT ( 'NONE',  ( -68.99615306438072082, 140.2400882881302948, -167.1454815528550739 ) ) ;
#17801=ORIENTED_EDGE ( 'NONE', *, *, #10196, .F. ) ;
#17802=ORIENTED_EDGE ( 'NONE', *, *, #9045, .F. ) ;
#17803=DIRECTION ( 'NONE',  ( 0.000000000000000000, 0.000000000000000000, -1.000000000000000000 ) ) ;
#17805=ORIENTED_EDGE ( 'NONE', *, *, #15690, .T. ) ;
#17816=CARTESIAN_POINT ( 'NONE',  ( -68.99615306438094819, 71.12504998813029999, -167.1454815528550739 ) ) ;
#17825=EDGE_CURVE ( 'NONE', #6193, #3274, #668, .T. ) ;
#17831=DIRECTION ( 'NONE',  ( 1.000000000000000000, 0.000000000000000000, 0.000000000000000000 ) ) ;
#17833=CARTESIAN_POINT ( 'NONE',  ( -71.24615306438070661, 137.9174286652292096, -167.1454815528550739 ) ) ;
#17836=EDGE_CURVE ( 'NONE', #17497, #2025, #16464, .T. ) ;
#17837=ADVANCED_FACE ( 'NONE', ( #13487 ), #2339, .T. ) ;
#17840=DIRECTION ( 'NONE',  ( 0.3420201433256649937, 0.9396926207859097602, -0.000000000000000000 ) ) ;
#17841=ORIENTED_EDGE ( 'NONE', *, *, #14826, .F. ) ;
#17846=ORIENTED_EDGE ( 'NONE', *, *, #6061, .T. ) ;
#17847=ADVANCED_FACE ( 'NONE', ( #8152 ), #18071, .T. ) ;
#17850=EDGE_CURVE ( 'NONE', #11906, #5703, #4872, .T. ) ;
#17853=EDGE_CURVE ( 'NONE', #12932, #13576, #7869, .T. ) ;
#17860=VERTEX_POINT ( 'NONE', #3842 ) ;
#17861=CARTESIAN_POINT ( 'NONE',  ( -71.24615306438070661, 147.3422066152292871, -167.1454815528550739 ) ) ;
#17872=CARTESIAN_POINT ( 'NONE',  ( -71.24615306438117557, 2.828944715229236628, 15.00000000000006928 ) ) ;
#17876=CARTESIAN_POINT ( 'NONE',  ( -71.24615306438086293, 100.2183168652291982, 15.00000000000006928 ) ) ;
#17877=CARTESIAN_POINT ( 'NONE',  ( -127.5926225674731995, 47.87487112387803023, -15.00000000000000355 ) ) ;
#17881=DIRECTION ( 'NONE',  ( 0.000000000000000000, 0.000000000000000000, 1.000000000000000000 ) ) ;
#17882=EDGE_LOOP ( 'NONE', ( #8976, #6794, #1503, #6621 ) ) ;
#17883=LINE ( 'NONE', #13505, #9207 ) ;
#17888=EDGE_CURVE ( 'NONE', #12417, #8597, #16370, .T. ) ;
#17894=VERTEX_POINT ( 'NONE', #2159 ) ;
#17897=ORIENTED_EDGE ( 'NONE', *, *, #699, .F. ) ;
#17898=VECTOR ( 'NONE', #5760, 1000.000000000000000 ) ;
#17901=ORIENTED_EDGE ( 'NONE', *, *, #5942, .F. ) ;
#17902=VECTOR ( 'NONE', #16695, 1000.000000000000000 ) ;
#17903=DIRECTION ( 'NONE',  ( 1.000000000000000000, 0.000000000000000000, 0.000000000000000000 ) ) ;
#17906=ORIENTED_EDGE ( 'NONE', *, *, #8390, .T. ) ;
#17908=CARTESIAN_POINT ( 'NONE',  ( -71.24615306438104767, 22.56737135456382148, 15.00000000000006928 ) ) ;
#17913=CARTESIAN_POINT ( 'NONE',  ( -68.99615306438097662, 61.70027203813028649, 15.00000000000006928 ) ) ;
#17915=AXIS2_PLACEMENT_3D ( 'NONE', #3729, #2313, #9160 ) ;
#17920=DIRECTION ( 'NONE',  ( 0.000000000000000000, 0.000000000000000000, -1.000000000000000000 ) ) ;
#17923=ORIENTED_EDGE ( 'NONE', *, *, #3655, .F. ) ;
#17925=LINE ( 'NONE', #3523, #12707 ) ;
#17929=ORIENTED_EDGE ( 'NONE', *, *, #2974, .T. ) ;
#17934=VECTOR ( 'NONE', #1680, 1000.000000000000227 ) ;
#17937=EDGE_CURVE ( 'NONE', #1867, #2089, #8046, .T. ) ;
#17938=VECTOR ( 'NONE', #6871, 1000.000000000000000 ) ;
#17940=EDGE_CURVE ( 'NONE', #6562, #16328, #12275, .T. ) ;
#17942=LINE ( 'NONE', #547, #12668 ) ;
#17946=VECTOR ( 'NONE', #6682, 1000.000000000000000 ) ;
#17947=LINE ( 'NONE', #11141, #15978 ) ;
#17954=ORIENTED_EDGE ( 'NONE', *, *, #13378, .F. ) ;
#17968=CARTESIAN_POINT ( 'NONE',  ( -71.24615306438084872, 91.68240965456375591, -15.00000000000001421 ) ) ;
#17969=DIRECTION ( 'NONE',  ( 0.9396926207859097602, 0.3420201433256649381, 4.890320548438455808E-16 ) ) ;
#17974=CARTESIAN_POINT ( 'NONE',  ( -71.24615306438106188, 38.27533460456375281, -167.1454815528550739 ) ) ;
#17978=LINE ( 'NONE', #13500, #9040 ) ;
#17981=ORIENTED_EDGE ( 'NONE', *, *, #12894, .T. ) ;
#17982=CARTESIAN_POINT ( 'NONE',  ( -68.99615306438083451, 95.64293533166268446, 15.00000000000006928 ) ) ;
#17983=ORIENTED_EDGE ( 'NONE', *, *, #762, .T. ) ;
#17985=VERTEX_POINT ( 'NONE', #3938 ) ;
#17986=VECTOR ( 'NONE', #8834, 1000.000000000000000 ) ;
#17987=VERTEX_POINT ( 'NONE', #6838 ) ;
#17988=VECTOR ( 'NONE', #10679, 1000.000000000000000 ) ;
#17989=VECTOR ( 'NONE', #7154, 1000.000000000000000 ) ;
#17993=EDGE_LOOP ( 'NONE', ( #15343, #1303, #5907, #8333 ) ) ;
#17996=CARTESIAN_POINT ( 'NONE',  ( -71.24615306438111872, 22.56737135456379661, -15.00000000000001421 ) ) ;
#17997=ORIENTED_EDGE ( 'NONE', *, *, #10303, .F. ) ;
#17998=VECTOR ( 'NONE', #131, 1000.000000000000000 ) ;
#17999=DIRECTION ( 'NONE',  ( 0.000000000000000000, 1.000000000000000000, 0.000000000000000000 ) ) ;
#18002=VERTEX_POINT ( 'NONE', #17128 ) ;
#18004=CARTESIAN_POINT ( 'NONE',  ( -71.24615306438067819, 144.2006139652292518, -15.00000000000001421 ) ) ;
#18009=CARTESIAN_POINT ( 'NONE',  ( -71.24615306438114715, 12.25372266522925457, -167.1454815528550739 ) ) ;
#18013=CARTESIAN_POINT ( 'NONE',  ( -68.99615306438106188, 29.66948968166269296, 15.00000000000006928 ) ) ;
#18014=PLANE ( 'NONE',  #693 ) ;
#18017=VECTOR ( 'NONE', #15145, 999.9999999999998863 ) ;
#18020=AXIS2_PLACEMENT_3D ( 'NONE', #3626, #15041, #15229 ) ;
#18023=ORIENTED_EDGE ( 'NONE', *, *, #17937, .F. ) ;
#18024=EDGE_CURVE ( 'NONE', #5717, #15520, #15454, .T. ) ;
#18025=DIRECTION ( 'NONE',  ( 0.000000000000000000, 0.000000000000000000, 1.000000000000000000 ) ) ;
#18026=LINE ( 'NONE', #5209, #9431 ) ;
#18027=PLANE ( 'NONE',  #7337 ) ;
#18030=VERTEX_POINT ( 'NONE', #2833 ) ;
#18031=DIRECTION ( 'NONE',  ( 0.9396926207859171987, 0.3420201433256445100, 4.890320548438495251E-16 ) ) ;
#18033=VERTEX_POINT ( 'NONE', #15646 ) ;
#18038=ORIENTED_EDGE ( 'NONE', *, *, #4913, .T. ) ;
#18039=ORIENTED_EDGE ( 'NONE', *, *, #17366, .T. ) ;
#18042=ORIENTED_EDGE ( 'NONE', *, *, #2537, .T. ) ;
#18044=LINE ( 'NONE', #16270, #2179 ) ;
#18046=EDGE_CURVE ( 'NONE', #9806, #17985, #5709, .T. ) ;
#18047=CARTESIAN_POINT ( 'NONE',  ( -71.24615306438097662, 59.37761241522920841, -167.1454815528550739 ) ) ;
#18048=AXIS2_PLACEMENT_3D ( 'NONE', #8584, #8398, #4181 ) ;
#18053=ORIENTED_EDGE ( 'NONE', *, *, #6641, .T. ) ;
#18054=CARTESIAN_POINT ( 'NONE',  ( -71.24615306438079188, 112.7846874652292399, -167.1454815528550739 ) ) ;
#18055=CARTESIAN_POINT ( 'NONE',  ( -68.99615306438103346, 32.81108233166271759, -167.1454815528550739 ) ) ;
#18057=VECTOR ( 'NONE', #14527, 1000.000000000000000 ) ;
#18061=ORIENTED_EDGE ( 'NONE', *, *, #13159, .T. ) ;
#18067=VERTEX_POINT ( 'NONE', #18259 ) ;
#18071=PLANE ( 'NONE',  #371 ) ;
#18073=PLANE ( 'NONE',  #7297 ) ;
#18077=LINE ( 'NONE', #12672, #13211 ) ;
#18081=LINE ( 'NONE', #2264, #10795 ) ;
#18084=DIRECTION ( 'NONE',  ( -0.9396926207859084279, 0.3420201433256686574, -4.890320548438448905E-16 ) ) ;
#18087=CARTESIAN_POINT ( 'NONE',  ( -71.24615306438106188, 38.27533460456375281, -167.1454815528550739 ) ) ;
#18088=VERTEX_POINT ( 'NONE', #11436 ) ;
#18090=ADVANCED_FACE ( 'NONE', ( #11341 ), #8339, .T. ) ;
#18091=ADVANCED_FACE ( 'NONE', ( #5537 ), #11261, .T. ) ;
#18099=CARTESIAN_POINT ( 'NONE',  ( -71.24615306438114715, 9.112130015229229940, -167.1454815528550739 ) ) ;
#18102=EDGE_CURVE ( 'NONE', #12836, #11918, #12936, .T. ) ;
#18106=EDGE_LOOP ( 'NONE', ( #15824, #3701, #4758, #18173 ) ) ;
#18109=DIRECTION ( 'NONE',  ( 0.3420201433256686574, -0.9396926207859084279, 0.000000000000000000 ) ) ;
#18110=EDGE_LOOP ( 'NONE', ( #12265, #5459, #14599, #1973 ) ) ;
#18111=FACE_OUTER_BOUND ( 'NONE', #11147, .T. ) ;
#18115=DIRECTION ( 'NONE',  ( 0.000000000000000000, 0.000000000000000000, 1.000000000000000000 ) ) ;
#18117=ORIENTED_EDGE ( 'NONE', *, *, #6030, .T. ) ;
#18119=DIRECTION ( 'NONE',  ( 0.3420201433256675472, 0.9396926207859088720, -0.000000000000000000 ) ) ;
#18120=LINE ( 'NONE', #16692, #410 ) ;
#18122=ORIENTED_EDGE ( 'NONE', *, *, #11958, .F. ) ;
#18125=DIRECTION ( 'NONE',  ( 0.000000000000000000, 0.000000000000000000, -1.000000000000000000 ) ) ;
#18127=VERTEX_POINT ( 'NONE', #471 ) ;
#18128=LINE ( 'NONE', #2500, #917 ) ;
#18129=CARTESIAN_POINT ( 'NONE',  ( -68.99615306438077766, 111.3508985816626335, -15.00000000000001421 ) ) ;
#18133=ORIENTED_EDGE ( 'NONE', *, *, #11667, .T. ) ;
#18134=LINE ( 'NONE', #5308, #2234 ) ;
#18136=ORIENTED_EDGE ( 'NONE', *, *, #8011, .F. ) ;
#18140=EDGE_CURVE ( 'NONE', #3197, #18067, #8893, .T. ) ;
#18141=VERTEX_POINT ( 'NONE', #4666 ) ;
#18145=ORIENTED_EDGE ( 'NONE', *, *, #11845, .F. ) ;
#18146=LINE ( 'NONE', #1318, #14787 ) ;
#18151=CARTESIAN_POINT ( 'NONE',  ( -68.99615306438091977, 74.26664263813029265, -167.1454815528550739 ) ) ;
#18157=DIRECTION ( 'NONE',  ( 1.000000000000000000, 0.000000000000000000, 0.000000000000000000 ) ) ;
#18160=ORIENTED_EDGE ( 'NONE', *, *, #7284, .T. ) ;
#18165=EDGE_CURVE ( 'NONE', #17387, #13170, #4579, .T. ) ;
#18167=FACE_OUTER_BOUND ( 'NONE', #8167, .T. ) ;
#18173=ORIENTED_EDGE ( 'NONE', *, *, #15181, .F. ) ;
#18176=VECTOR ( 'NONE', #11832, 1000.000000000000000 ) ;
#18178=DIRECTION ( 'NONE',  ( 0.9396926207859043201, 0.3420201433256802037, 0.000000000000000000 ) ) ;
#18179=VERTEX_POINT ( 'NONE', #17483 ) ;
#18180=EDGE_CURVE ( 'NONE', #5451, #5525, #13292, .T. ) ;
#18182=ORIENTED_EDGE ( 'NONE', *, *, #14845, .T. ) ;
#18187=EDGE_CURVE ( 'NONE', #9316, #18141, #1509, .T. ) ;
#18188=VERTEX_POINT ( 'NONE', #4403 ) ;
#18190=EDGE_CURVE ( 'NONE', #17894, #16349, #8982, .T. ) ;
#18192=CARTESIAN_POINT ( 'NONE',  ( -71.24615306438103346, 47.70011255456374499, 15.00000000000006928 ) ) ;
#18197=ORIENTED_EDGE ( 'NONE', *, *, #16029, .T. ) ;
#18202=LINE ( 'NONE', #5473, #12740 ) ;
#18203=VECTOR ( 'NONE', #1730, 1000.000000000000000 ) ;
#18204=EDGE_CURVE ( 'NONE', #8426, #15763, #7311, .T. ) ;
#18205=LINE ( 'NONE', #11098, #17751 ) ;
#18207=EDGE_CURVE ( 'NONE', #10434, #2512, #13107, .T. ) ;
#18208=EDGE_CURVE ( 'NONE', #10713, #4400, #202, .T. ) ;
#18210=ORIENTED_EDGE ( 'NONE', *, *, #1425, .F. ) ;
#18212=CARTESIAN_POINT ( 'NONE',  ( -71.24615306438109030, 27.96168591522921076, -167.1454815528550739 ) ) ;
#18213=EDGE_CURVE ( 'NONE', #18272, #8741, #4486, .T. ) ;
#18216=CARTESIAN_POINT ( 'NONE',  ( -68.99615306438106188, 29.66948968166269651, -15.00000000000001421 ) ) ;
#18219=DIRECTION ( 'NONE',  ( 0.000000000000000000, 1.000000000000000000, 0.000000000000000000 ) ) ;
#18223=DIRECTION ( 'NONE',  ( 0.000000000000000000, 0.000000000000000000, 1.000000000000000000 ) ) ;
#18240=DIRECTION ( 'NONE',  ( -0.9396926207859084279, 0.3420201433256686574, -4.890320548438448905E-16 ) ) ;
#18243=VERTEX_POINT ( 'NONE', #1869 ) ;
#18246=VECTOR ( 'NONE', #10656, 1000.000000000000000 ) ;
#18247=CARTESIAN_POINT ( 'NONE',  ( -71.24615306438080609, 107.3903729045637192, -15.00000000000001421 ) ) ;
#18250=FACE_OUTER_BOUND ( 'NONE', #12410, .T. ) ;
#18259=CARTESIAN_POINT ( 'NONE',  ( -68.99615306438097662, 61.70027203813028649, -15.00000000000001421 ) ) ;
#18260=LINE ( 'NONE', #3843, #16254 ) ;
#18262=LINE ( 'NONE', #10034, #15833 ) ;
#18265=DIRECTION ( 'NONE',  ( 0.000000000000000000, 0.000000000000000000, 1.000000000000000000 ) ) ;
#18268=ORIENTED_EDGE ( 'NONE', *, *, #11071, .T. ) ;
#18269=VECTOR ( 'NONE', #6581, 1000.000000000000000 ) ;
#18272=VERTEX_POINT ( 'NONE', #4746 ) ;
#18274=VECTOR ( 'NONE', #14720, 999.9999999999998863 ) ;
#18276=ORIENTED_EDGE ( 'NONE', *, *, #13267, .T. ) ;
#18279=AXIS2_PLACEMENT_3D ( 'NONE', #8161, #1068, #6760 ) ;
#18288=EDGE_CURVE ( 'NONE', #2703, #1662, #13370, .T. ) ;
#18292=CARTESIAN_POINT ( 'NONE',  ( -71.24615306438120399, -0.3126479347707321610, 15.00000000000006928 ) ) ;
#18293=EDGE_CURVE ( 'NONE', #5859, #11918, #15045, .T. ) ;
#18294=DIRECTION ( 'NONE',  ( 0.000000000000000000, 0.000000000000000000, 1.000000000000000000 ) ) ;
#18296=CARTESIAN_POINT ( 'NONE',  ( -68.99615306438106188, 29.66948968166269296, -15.00000000000001421 ) ) ;
#18299=AXIS2_PLACEMENT_3D ( 'NONE', #1654, #12896, #68 ) ;
#18300=LINE ( 'NONE', #9587, #10324 ) ;
#18302=ADVANCED_FACE ( 'NONE', ( #17768 ), #15138, .T. ) ;
#18305=ORIENTED_EDGE ( 'NONE', *, *, #4285, .F. ) ;
#18308=CARTESIAN_POINT ( 'NONE',  ( -68.99615306438111872, 10.81993378166265529, -167.1454815528550739 ) ) ;
#18309=VECTOR ( 'NONE', #218, 1000.000000000000000 ) ;
#18311=EDGE_CURVE ( 'NONE', #13644, #11558, #6529, .T. ) ;
#18313=LINE ( 'NONE', #5486, #5934 ) ;
#18315=EDGE_CURVE ( 'NONE', #12217, #13601, #3353, .T. ) ;
#18316=FACE_OUTER_BOUND ( 'NONE', #372, .T. ) ;
#18319=DIRECTION ( 'NONE',  ( 0.000000000000000000, 0.000000000000000000, -1.000000000000000000 ) ) ;
#18323=EDGE_CURVE ( 'NONE', #11131, #16032, #18044, .T. ) ;
#18324=CARTESIAN_POINT ( 'NONE',  ( -68.99615306438091977, 74.26664263813029265, -167.1454815528550739 ) ) ;
#18329=EDGE_CURVE ( 'NONE', #14197, #3236, #17942, .T. ) ;
#18333=ADVANCED_FACE ( 'NONE', ( #14857 ), #5127, .T. ) ;
#18334=LINE ( 'NONE', #5679, #16735 ) ;
#18337=VECTOR ( 'NONE', #5888, 1000.000000000000000 ) ;
#18350=DIRECTION ( 'NONE',  ( 0.000000000000000000, 0.000000000000000000, 1.000000000000000000 ) ) ;
#18352=ADVANCED_FACE ( 'NONE', ( #14941 ), #13464, .T. ) ;
#18354=VECTOR ( 'NONE', #11009, 1000.000000000000000 ) ;
#18356=ORIENTED_EDGE ( 'NONE', *, *, #18288, .F. ) ;
#18361=ORIENTED_EDGE ( 'NONE', *, *, #9867, .F. ) ;
#18364=DIRECTION ( 'NONE',  ( 1.000000000000000000, 0.000000000000000000, 0.000000000000000000 ) ) ;
#18366=EDGE_CURVE ( 'NONE', #12199, #15122, #12163, .T. ) ;
#18375=ORIENTED_EDGE ( 'NONE', *, *, #5207, .T. ) ;
#18385=PLANE ( 'NONE',  #8455 ) ;
#18387=EDGE_LOOP ( 'NONE', ( #2723, #12233, #6206, #11255 ) ) ;
#18389=EDGE_LOOP ( 'NONE', ( #1569, #13341, #13956, #12106 ) ) ;
#18393=DIRECTION ( 'NONE',  ( -0.9396926207859084279, 0.3420201433256686574, 1.086737899652989892E-16 ) ) ;
#18395=PLANE ( 'NONE',  #9905 ) ;
#18400=ORIENTED_EDGE ( 'NONE', *, *, #4904, .F. ) ;
#18401=DIRECTION ( 'NONE',  ( 0.3420201433256701007, -0.9396926207859078728, 0.000000000000000000 ) ) ;
#18403=CARTESIAN_POINT ( 'NONE',  ( -68.99615306438072082, 139.6252324316626812, 15.00000000000006928 ) ) ;
#18406=AXIS2_PLACEMENT_3D ( 'NONE', #2027, #5012, #4653 ) ;
#18409=CARTESIAN_POINT ( 'NONE',  ( -68.99615306438120399, -1.746436818337276931, -15.00000000000001421 ) ) ;
#18410=CARTESIAN_POINT ( 'NONE',  ( -68.99615306438074924, 120.7756765316626542, 15.00000000000006928 ) ) ;
#18411=ORIENTED_EDGE ( 'NONE', *, *, #8873, .F. ) ;
#18413=CARTESIAN_POINT ( 'NONE',  ( -71.24615306438114715, 13.14259340456377956, -167.1454815528550739 ) ) ;
#18414=FACE_OUTER_BOUND ( 'NONE', #10605, .T. ) ;
#18415=DIRECTION ( 'NONE',  ( 0.3420201433256519485, 0.9396926207859145341, -0.000000000000000000 ) ) ;
#18416=ORIENTED_EDGE ( 'NONE', *, *, #10821, .T. ) ;
#18419=CARTESIAN_POINT ( 'NONE',  ( -71.24615306438076345, 119.0678727652292253, -167.1454815528550739 ) ) ;
#18421=DIRECTION ( 'NONE',  ( -0.9396926207859069846, 0.3420201433256723766, 0.000000000000000000 ) ) ;
#18423=DIRECTION ( 'NONE',  ( -0.9396926207859092051, 0.3420201433256663259, 1.086737899652990755E-16 ) ) ;
#18424=DIRECTION ( 'NONE',  ( 0.000000000000000000, 1.000000000000000000, 0.000000000000000000 ) ) ;
#18426=DIRECTION ( 'NONE',  ( 0.3420201433256727097, 0.9396926207859069846, -0.000000000000000000 ) ) ;
#18428=EDGE_CURVE ( 'NONE', #11558, #5703, #16827, .T. ) ;
#18433=DIRECTION ( 'NONE',  ( -0.9396926207859084279, 0.3420201433256686574, -4.890320548438448905E-16 ) ) ;
#18436=VERTEX_POINT ( 'NONE', #3918 ) ;
#18439=CARTESIAN_POINT ( 'NONE',  ( -68.99615306438070661, 137.0984956381303164, -167.1454815528550739 ) ) ;
#18440=ADVANCED_FACE ( 'NONE', ( #12452 ), #9628, .T. ) ;
#18443=CARTESIAN_POINT ( 'NONE',  ( -94.45685920050698314, -47.21335801510345220, 15.00000000000006928 ) ) ;
#18447=ORIENTED_EDGE ( 'NONE', *, *, #13860, .T. ) ;
#18450=LINE ( 'NONE', #13021, #11616 ) ;
#18458=CARTESIAN_POINT ( 'NONE',  ( -71.24615306438094819, 69.69126110456375045, -167.1454815528550739 ) ) ;
#18459=DIRECTION ( 'NONE',  ( 0.000000000000000000, 0.000000000000000000, -1.000000000000000000 ) ) ;
#18464=VERTEX_POINT ( 'NONE', #2810 ) ;
#18467=LINE ( 'NONE', #4233, #14152 ) ;
#18468=CARTESIAN_POINT ( 'NONE',  ( -68.99615306438072082, 133.9569029881302811, -167.1454815528550739 ) ) ;
#18474=VERTEX_POINT ( 'NONE', #14230 ) ;
#18475=ORIENTED_EDGE ( 'NONE', *, *, #1162, .F. ) ;
#18477=CARTESIAN_POINT ( 'NONE',  ( -68.99615306438077766, 118.2489397381302751, -15.00000000000001421 ) ) ;
#18478=VERTEX_POINT ( 'NONE', #1406 ) ;
#18483=VECTOR ( 'NONE', #10769, 1000.000000000000000 ) ;
#18486=VERTEX_POINT ( 'NONE', #14656 ) ;
#18490=AXIS2_PLACEMENT_3D ( 'NONE', #11125, #8307, #11311 ) ;
#18497=CARTESIAN_POINT ( 'NONE',  ( -71.24615306438069240, 141.9478920545637664, -15.00000000000001421 ) ) ;
#18499=ORIENTED_EDGE ( 'NONE', *, *, #8192, .T. ) ;
#18500=CARTESIAN_POINT ( 'NONE',  ( -71.24615306438106188, 37.38646386522923137, -167.1454815528550739 ) ) ;
#18505=CARTESIAN_POINT ( 'NONE',  ( -71.24615306438076345, 119.0678727652292253, -15.00000000000001421 ) ) ;
#18511=ADVANCED_FACE ( 'NONE', ( #15723 ), #8686, .T. ) ;
#18515=VECTOR ( 'NONE', #16988, 999.9999999999998863 ) ;
#18517=CARTESIAN_POINT ( 'NONE',  ( -68.99615306438094819, 64.22700883166265839, -167.1454815528550739 ) ) ;
#18519=ORIENTED_EDGE ( 'NONE', *, *, #3999, .F. ) ;
#18539=COLOUR_RGB('Light Blue',0.38,0.62,0.78);
#18540=FILL_AREA_STYLE_COLOUR('',#18539);
#18541=FILL_AREA_STYLE('',(#18540));
#18542=SURFACE_STYLE_FILL_AREA(#18541);
#18543=SURFACE_SIDE_STYLE('',(#18542));
#18544=SURFACE_STYLE_USAGE(.BOTH.,#18543);
#18545=PRESENTATION_STYLE_ASSIGNMENT((#18544));
ENDSEC;
END-ISO-10303-21;
